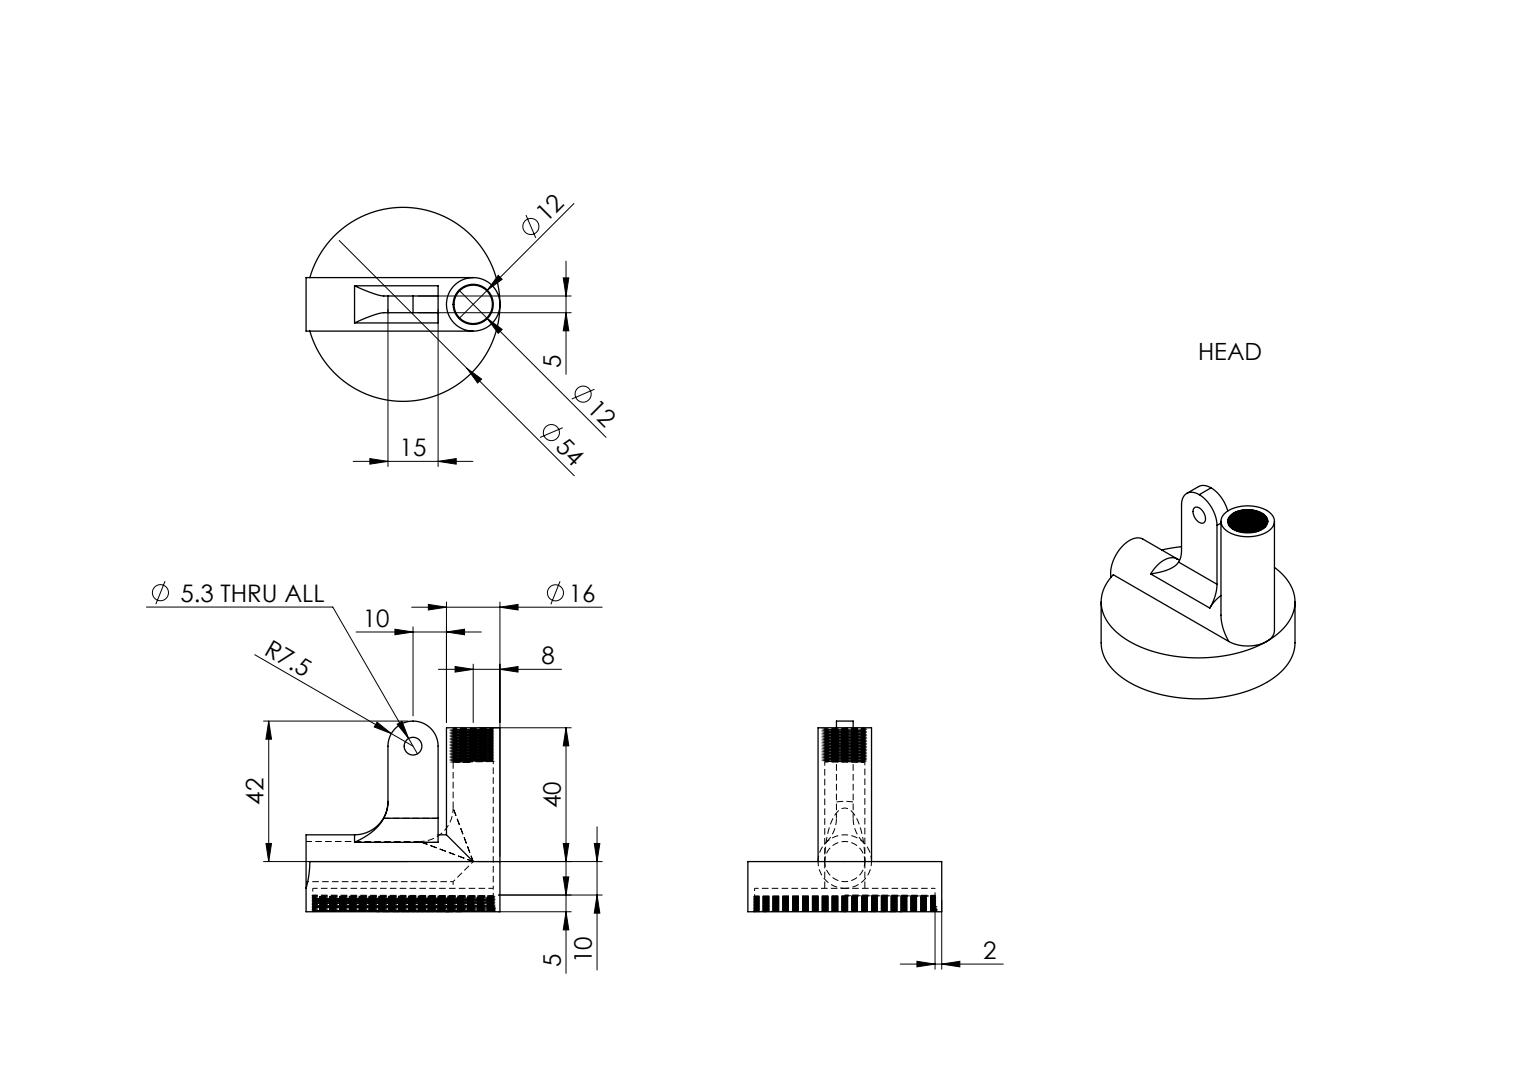
ISO-10303-21;
HEADER;
FILE_DESCRIPTION (('STEP AP214'),
    '1' );
FILE_NAME ('head.step',
    '2026-10-31T03:36:27',
    ( '' ),
    ( '' ),
    'SwSTEP 2.0',
    'SolidWorks 2026',
    '' );
FILE_SCHEMA (( 'AUTOMOTIVE_DESIGN' ));
ENDSEC;

DATA;
#9=CARTESIAN_POINT ( 'NONE',  ( -13.62178482187498396, 196.7843750006145456, 23.59362340125808188 ) ) ;
#16=CARTESIAN_POINT ( 'NONE',  ( 18.00000000000000000, 239.6312500012290343, -5.196152422706630247 ) ) ;
#27=CARTESIAN_POINT ( 'NONE',  ( 26.75643035624999655, 248.1718750006145342, -7.049594010296217766E-16 ) ) ;
#29=CARTESIAN_POINT ( 'NONE',  ( -17.60279642935561029, 194.9999999999999716, 20.73731651351060989 ) ) ;
#47=CARTESIAN_POINT ( 'NONE',  ( 22.60769515458672529, 246.3236538117967029, -6.000000000000004441 ) ) ;
#48=CARTESIAN_POINT ( 'NONE',  ( 26.75643035624999655, 244.7218750006145456, -3.323476615752271712 ) ) ;
#50=LINE ( 'NONE', #15224, #14231 ) ;
#52=ORIENTED_EDGE ( 'NONE', *, *, #4531, .T. ) ;
#54=CARTESIAN_POINT ( 'NONE',  ( 23.99999999999999645, 245.8562500012290570, -5.196152422706631135 ) ) ;
#63=ORIENTED_EDGE ( 'NONE', *, *, #14775, .T. ) ;
#69=CARTESIAN_POINT ( 'NONE',  ( 23.87821517812499650, 246.8968750006145285, -4.985214923628404904 ) ) ;
#73=CARTESIAN_POINT ( 'NONE',  ( 19.06670604969950489, 215.1554505341192964, -5.693556627486040966 ) ) ;
#95=DIRECTION ( 'NONE',  ( 0.000000000000000000, 0.000000000000000000, 1.000000000000000000 ) ) ;
#99=CARTESIAN_POINT ( 'NONE',  ( 5.727106289114498080E-15, 196.0625000000000000, 31.17691453623979214 ) ) ;
#102=CARTESIAN_POINT ( 'NONE',  ( 26.75643035624999655, 247.8718750006145228, -3.323476615752271268 ) ) ;
#110=CARTESIAN_POINT ( 'NONE',  ( 26.99999999999999645, 240.2874999999999659, 3.464101615137751278 ) ) ;
#116=VECTOR ( 'NONE', #35899, 1000.000000000000000 ) ;
#117=CARTESIAN_POINT ( 'NONE',  ( 26.99999999999999645, 194.9750000012290343, -15.58845726811990495 ) ) ;
#120=ADVANCED_FACE ( 'NONE', ( #26675 ), #705, .F. ) ;
#132=CARTESIAN_POINT ( 'NONE',  ( -1.926257025242585782E-15, 195.6968750006145683, -31.45816453501075927 ) ) ;
#144=CYLINDRICAL_SURFACE ( 'NONE', #32201, 27.00000000000000000 ) ;
#145=CARTESIAN_POINT ( 'NONE',  ( 22.60769515458672885, 244.9174038105676630, -5.999999999999998224 ) ) ;
#146=ADVANCED_FACE ( 'NONE', ( #11518 ), #17218, .F. ) ;
#148=CARTESIAN_POINT ( 'NONE',  ( -13.50000000000000533, 195.0875000012290457, -23.38268590217984411 ) ) ;
#149=VERTEX_POINT ( 'NONE', #2983 ) ;
#152=LINE ( 'NONE', #25749, #18668 ) ;
#156=CARTESIAN_POINT ( 'NONE',  ( 18.00000000000000355, 248.7249999999999943, 5.196152422706632912 ) ) ;
#157=CARTESIAN_POINT ( 'NONE',  ( 27.24356964374999279, 197.8156250006145171, -15.72908226750539207 ) ) ;
#163=CARTESIAN_POINT ( 'NONE',  ( -13.62178482187498396, 198.5281250006145228, 23.59362340125808188 ) ) ;
#164=CARTESIAN_POINT ( 'NONE',  ( 23.87821517812500005, 243.1468750006145285, 4.985214923628404016 ) ) ;
#169=CARTESIAN_POINT ( 'NONE',  ( 23.87821517812499650, 246.5593750006145228, -4.985214923628404904 ) ) ;
#173=CARTESIAN_POINT ( 'NONE',  ( 26.75643035624999655, 241.9093750006145171, -3.323476615752271268 ) ) ;
#175=EDGE_CURVE ( 'NONE', #2711, #16688, #11211, .T. ) ;
#176=CARTESIAN_POINT ( 'NONE',  ( 26.99999999999999645, 246.6812500012290457, -7.347880794884117764E-16 ) ) ;
#177=AXIS2_PLACEMENT_3D ( 'NONE', #6579, #20812, #23648 ) ;
#189=CARTESIAN_POINT ( 'NONE',  ( 21.00000000000000000, 241.9843750006145058, -6.646953231504538984 ) ) ;
#190=VERTEX_POINT ( 'NONE', #2796 ) ;
#196=DIRECTION ( 'NONE',  ( -0.000000000000000000, -0.000000000000000000, 1.000000000000000000 ) ) ;
#197=CARTESIAN_POINT ( 'NONE',  ( 5.778771075727756162E-15, 195.0218750006145569, 31.45816453501075927 ) ) ;
#198=EDGE_CURVE ( 'NONE', #717, #36155, #34079, .T. ) ;
#200=CARTESIAN_POINT ( 'NONE',  ( -7.234628195640263826, 196.8700961906613713, -27.00000000000003553 ) ) ;
#206=CARTESIAN_POINT ( 'NONE',  ( 26.75643035624999655, 249.4843750006145058, 3.323476615752267715 ) ) ;
#211=EDGE_CURVE ( 'NONE', #2909, #23659, #28387, .T. ) ;
#217=CARTESIAN_POINT ( 'NONE',  ( 15.24356964375000167, 248.4343750006145513, 3.323476615752272600 ) ) ;
#219=CARTESIAN_POINT ( 'NONE',  ( -17.17757150371551944, 194.9999999999999716, 21.09399746705422984 ) ) ;
#223=CARTESIAN_POINT ( 'NONE',  ( -28.99999999999999645, 201.9999999999999716, -1.007612034238798379E-23 ) ) ;
#224=CARTESIAN_POINT ( 'NONE',  ( 20.99999999999997868, 210.0000000000000000, -5.999999999999999112 ) ) ;
#234=CARTESIAN_POINT ( 'NONE',  ( 21.00000000000000000, 242.4625000000000057, 5.999999999999998224 ) ) ;
#237=CARTESIAN_POINT ( 'NONE',  ( 26.99999999999999645, 196.3250000012290570, -15.58845726811990495 ) ) ;
#239=CARTESIAN_POINT ( 'NONE',  ( 22.60769515458672885, 246.1388461906613827, 5.999999999999997335 ) ) ;
#240=CARTESIAN_POINT ( 'NONE',  ( 21.00000000000000000, 244.5718750006145115, 6.646953231504538984 ) ) ;
#245=CARTESIAN_POINT ( 'NONE',  ( 15.00000000000000000, 246.4562500012290513, 0.000000000000000000 ) ) ;
#248=CARTESIAN_POINT ( 'NONE',  ( 20.99999999999997868, 246.9625000000000057, 5.999999999999999112 ) ) ;
#253=VERTEX_POINT ( 'NONE', #25549 ) ;
#257=CARTESIAN_POINT ( 'NONE',  ( 15.24356964374999990, 246.1468750006145285, 0.000000000000000000 ) ) ;
#261=CARTESIAN_POINT ( 'NONE',  ( 17.34006124879648425, 219.7598366698888981, -4.770645753573318437 ) ) ;
#272=ORIENTED_EDGE ( 'NONE', *, *, #322, .F. ) ;
#282=LINE ( 'NONE', #23417, #32949 ) ;
#284=CARTESIAN_POINT ( 'NONE',  ( -26.99999999999998934, 195.9875000000000114, 15.58845726811991561 ) ) ;
#287=CARTESIAN_POINT ( 'NONE',  ( 20.99999999999999645, 245.9218750006145626, 6.646953231504538984 ) ) ;
#291=CARTESIAN_POINT ( 'NONE',  ( 20.99999999999999645, 185.0294372515228645, -5.999999999999999112 ) ) ;
#295=CARTESIAN_POINT ( 'NONE',  ( 26.99999999999999645, 241.6374999999999886, 3.464101615137751278 ) ) ;
#299=EDGE_LOOP ( 'NONE', ( #11498, #11713, #35971, #5755 ) ) ;
#306=CARTESIAN_POINT ( 'NONE',  ( 15.24356964374999990, 239.9593750006145285, 0.000000000000000000 ) ) ;
#316=CARTESIAN_POINT ( 'NONE',  ( 25.00272249592519103, 194.9999999999998863, 10.65893590749716324 ) ) ;
#317=CARTESIAN_POINT ( 'NONE',  ( -27.24356964375000345, 195.8093750006145513, 0.000000000000000000 ) ) ;
#321=CARTESIAN_POINT ( 'NONE',  ( 15.00000000000000000, 244.6187500012290741, -3.464101615137752610 ) ) ;
#322=EDGE_CURVE ( 'NONE', #20414, #21332, #8073, .T. ) ;
#334=CARTESIAN_POINT ( 'NONE',  ( -20.80563922340697403, 195.0000000000000284, -17.20829382900668136 ) ) ;
#339=CARTESIAN_POINT ( 'NONE',  ( -1.926257025242585782E-15, 196.5968750006145456, -31.45816453501076637 ) ) ;
#343=CARTESIAN_POINT ( 'NONE',  ( 26.99999999999999645, 249.3249999999999886, -7.347880794884117764E-16 ) ) ;
#344=CARTESIAN_POINT ( 'NONE',  ( 13.62178482187499640, 197.4031250006145228, -23.59362340125807123 ) ) ;
#346=APPLICATION_CONTEXT ( 'automotive_design' ) ;
#350=CARTESIAN_POINT ( 'NONE',  ( 27.24356964375000700, 195.0406250006145399, 15.72908226750537075 ) ) ;
#351=CARTESIAN_POINT ( 'NONE',  ( 21.00000000000000000, 241.5343750006145171, -6.646953231504538984 ) ) ;
#355=CARTESIAN_POINT ( 'NONE',  ( 15.24356964375000167, 248.0968750006145456, 3.323476615752272600 ) ) ;
#356=( BOUNDED_CURVE ( )  B_SPLINE_CURVE ( 2, ( #17925, #26623, #26814, #31940, #5972, #15073, #12223, #29469, #653 ),
 .UNSPECIFIED., .F., .F. ) 
 B_SPLINE_CURVE_WITH_KNOTS ( ( 3, 2, 2, 2, 3 ),
 ( 0.7934782608695651884, 0.7971014492753623060, 0.8043478260869565410, 0.8115942028985507761, 0.8152173913043478937 ),
 .UNSPECIFIED. ) 
 CURVE ( )  GEOMETRIC_REPRESENTATION_ITEM ( )  RATIONAL_B_SPLINE_CURVE ( ( 0.9330127018922194093, 0.9330127018922194093, 1.000000000000000000, 0.8660254037844387076, 1.000000000000000000, 0.8660254037844387076, 1.000000000000000000, 0.9330127018922182991, 0.9330127018922192983 ) ) 
 REPRESENTATION_ITEM ( '' )  );
#360=CARTESIAN_POINT ( 'NONE',  ( 23.87821517812499650, 241.9468750006145115, -4.985214923628404904 ) ) ;
#367=CARTESIAN_POINT ( 'NONE',  ( 0.000000000000000000, 210.0000000000000284, 0.000000000000000000 ) ) ;
#369=CARTESIAN_POINT ( 'NONE',  ( 12.48663586349064403, 194.9999999999999716, 24.21355016816918493 ) ) ;
#376=CARTESIAN_POINT ( 'NONE',  ( 23.87821517812499650, 241.4968750006144944, -4.985214923628404904 ) ) ;
#382=CARTESIAN_POINT ( 'NONE',  ( 26.99999999999999645, 241.6375000000000171, 3.464101615137751278 ) ) ;
#390=CARTESIAN_POINT ( 'NONE',  ( 26.75643035624999655, 248.6593750006145171, -3.323476615752271712 ) ) ;
#394=CARTESIAN_POINT ( 'NONE',  ( 2.999999999999997335, 244.5000000000000000, 2.500000000000000000 ) ) ;
#401=CARTESIAN_POINT ( 'NONE',  ( 20.99999999999999289, 245.4437500012290343, -5.999999999999997335 ) ) ;
#406=AXIS2_PLACEMENT_3D ( 'NONE', #8514, #8149, #2814 ) ;
#408=CARTESIAN_POINT ( 'NONE',  ( 15.00000000000000000, 248.6500000000000057, 0.000000000000000000 ) ) ;
#414=EDGE_CURVE ( 'NONE', #36155, #4778, #26130, .T. ) ;
#421=CARTESIAN_POINT ( 'NONE',  ( 13.50000000000001421, 195.7625000012290570, 23.38268590217984055 ) ) ;
#422=CARTESIAN_POINT ( 'NONE',  ( -1.045839947578415010E-13, 196.1750000012290229, 27.00000000000000355 ) ) ;
#425=EDGE_CURVE ( 'NONE', #21070, #14808, #25046, .T. ) ;
#426=CARTESIAN_POINT ( 'NONE',  ( 21.00000000000000000, 245.2468750006145228, -6.646953231504538984 ) ) ;
#428=CARTESIAN_POINT ( 'NONE',  ( 18.12178482187500350, 240.0343750006145171, 4.985214923628407568 ) ) ;
#431=VECTOR ( 'NONE', #33908, 1000.000000000000000 ) ;
#432=CARTESIAN_POINT ( 'NONE',  ( 21.00000000000000000, 247.2437500012290457, -6.928203230275506996 ) ) ;
#439=ORIENTED_EDGE ( 'NONE', *, *, #30910, .T. ) ;
#443=CARTESIAN_POINT ( 'NONE',  ( 26.75643035624999655, 247.6843750006145513, 3.323476615752267715 ) ) ;
#446=CARTESIAN_POINT ( 'NONE',  ( 20.28004929559795499, 210.7199507044251732, -5.999999999998712141 ) ) ;
#472=CARTESIAN_POINT ( 'NONE',  ( 26.75643035624999655, 245.6218750006145513, -3.323476615752271268 ) ) ;
#473=ORIENTED_EDGE ( 'NONE', *, *, #4147, .F. ) ;
#480=CARTESIAN_POINT ( 'NONE',  ( 15.00000000000000000, 241.4124999999999943, -3.464101615137752166 ) ) ;
#483=VERTEX_POINT ( 'NONE', #17594 ) ;
#485=ORIENTED_EDGE ( 'NONE', *, *, #35805, .T. ) ;
#488=CARTESIAN_POINT ( 'NONE',  ( 23.99999999999999645, 243.1000000000000227, -5.196152422706631135 ) ) ;
#493=CARTESIAN_POINT ( 'NONE',  ( 26.75643035624999655, 241.4968750006145228, 3.323476615752267715 ) ) ;
#502=CARTESIAN_POINT ( 'NONE',  ( 27.24356964374999635, 196.0718750006145683, -15.72908226750539029 ) ) ;
#511=( BOUNDED_CURVE ( )  B_SPLINE_CURVE ( 2, ( #32601, #35627, #6825, #12519, #18216, #9301, #29756, #1322, #32976, #12324, #3608, #27109, #24272, #35815, #30140, #26534, #15740, #564, #35248, #20873, #32412, #6454, #18026, #30707, #4726, #36373, #1507, #16302, #27480, #16490, #19157, #25003, #21994, #1694, #2070, #4909, #7769, #10976, #19347, #30522, #36559, #10419, #13082, #13268, #27849, #10231, #24636, #28038, #30328, #8146, #13644, #36187, #22180, #31076, #30886, #25197, #2254, #36750, #10790, #33727, #33359, #4541, #7394, #10600, #21806, #22364, #1882, #33912, #33541, #4352, #22547, #18967, #7954, #19529, #5099, #16678, #34096, #28225, #7581, #15932, #13453, #25379, #13833, #16118, #27669, #36929, #24820, #339, #20454, #34647, #20266, #34468, #5842, #5284, #28584, #37482, #8511, #14381, #6025, #22737, #2998, #20077, #34286, #23291, #19718, #14568, #31805, #8330, #16864, #8692, #37302, #19900, #17420, #11904, #23104, #5463, #28960, #35024, #11533, #34836, #31258, #2811, #31441, #17611, #28401, #17046, #14198, #26120, #25939, #31622, #2622 ),
 .UNSPECIFIED., .F., .F. ) 
 B_SPLINE_CURVE_WITH_KNOTS ( ( 3, 2, 2, 2, 2, 2, 2, 2, 2, 2, 2, 2, 2, 2, 2, 2, 2, 2, 2, 2, 2, 2, 2, 2, 2, 2, 2, 2, 2, 2, 2, 2, 2, 2, 2, 2, 2, 2, 2, 2, 2, 2, 2, 2, 2, 2, 2, 2, 2, 2, 2, 2, 2, 2, 2, 2, 2, 2, 2, 2, 2, 2, 2, 2, 2, 3 ),
 ( 0.000000000000000000, 0.01388888888888888812, 0.02777777777777777624, 0.04166666666666666435, 0.05555555555555555247, 0.06944444444444444753, 0.08333333333333332871, 0.09722222222222222376, 0.1111111111111111049, 0.1250000000000000000, 0.1388888888888888951, 0.1527777777777777901, 0.1666666666666666574, 0.1805555555555555525, 0.1944444444444444475, 0.2083333333333333426, 0.2222222222222222099, 0.2361111111111111049, 0.2500000000000000000, 0.2638888888888888951, 0.2777777777777777901, 0.2916666666666666852, 0.3055555555555555802, 0.3194444444444444198, 0.3333333333333333148, 0.3472222222222222099, 0.3611111111111111049, 0.3750000000000000000, 0.3888888888888888951, 0.4027777777777777901, 0.4166666666666666852, 0.4305555555555555802, 0.4444444444444444198, 0.4583333333333333148, 0.4722222222222222099, 0.4861111111111111049, 0.5000000000000000000, 0.5138888888888888395, 0.5277777777777777901, 0.5416666666666666297, 0.5555555555555555802, 0.5694444444444444198, 0.5833333333333333703, 0.5972222222222222099, 0.6111111111111111605, 0.6250000000000000000, 0.6388888888888888395, 0.6527777777777777901, 0.6666666666666666297, 0.6805555555555555802, 0.6944444444444444198, 0.7083333333333333703, 0.7222222222222222099, 0.7361111111111111605, 0.7500000000000000000, 0.7638888888888888395, 0.7777777777777777901, 0.7916666666666666297, 0.8055555555555555802, 0.8194444444444444198, 0.8333333333333333703, 0.8472222222222222099, 0.8611111111111111605, 0.8750000000000000000, 0.8888888888888888395, 0.8996968925187518451 ),
 .UNSPECIFIED. ) 
 CURVE ( )  GEOMETRIC_REPRESENTATION_ITEM ( )  RATIONAL_B_SPLINE_CURVE ( ( 1.000000000000000000, 0.8660254037844387076, 1.000000000000000000, 0.8660254037844387076, 1.000000000000000000, 0.8660254037844387076, 1.000000000000000000, 0.8660254037844387076, 1.000000000000000000, 0.8660254037844387076, 1.000000000000000000, 0.8660254037844387076, 1.000000000000000000, 0.8660254037844387076, 1.000000000000000000, 0.8660254037844387076, 1.000000000000000000, 0.8660254037844387076, 1.000000000000000000, 0.8660254037844387076, 1.000000000000000000, 0.8660254037844387076, 1.000000000000000000, 0.8660254037844387076, 1.000000000000000000, 0.8660254037844387076, 1.000000000000000000, 0.8660254037844387076, 1.000000000000000000, 0.8660254037844387076, 1.000000000000000000, 0.8660254037844387076, 1.000000000000000000, 0.8660254037844387076, 1.000000000000000000, 0.8660254037844387076, 1.000000000000000000, 0.8660254037844387076, 1.000000000000000000, 0.8660254037844387076, 1.000000000000000000, 0.8660254037844387076, 1.000000000000000000, 0.8660254037844387076, 1.000000000000000000, 0.8660254037844387076, 1.000000000000000000, 0.8660254037844387076, 1.000000000000000000, 0.8660254037844387076, 1.000000000000000000, 0.8660254037844387076, 1.000000000000000000, 0.8660254037844387076, 1.000000000000000000, 0.8660254037844387076, 1.000000000000000000, 0.8660254037844387076, 1.000000000000000000, 0.8660254037844387076, 1.000000000000000000, 0.8660254037844387076, 1.000000000000000000, 0.8660254037844387076, 1.000000000000000000, 0.8660254037844387076, 1.000000000000000000, 0.8660254037844387076, 1.000000000000000000, 0.8660254037844387076, 1.000000000000000000, 0.8660254037844387076, 1.000000000000000000, 0.8660254037844387076, 1.000000000000000000, 0.8660254037844387076, 1.000000000000000000, 0.8660254037844387076, 1.000000000000000000, 0.8660254037844387076, 1.000000000000000000, 0.8660254037844387076, 1.000000000000000000, 0.8660254037844387076, 1.000000000000000000, 0.8660254037844387076, 1.000000000000000000, 0.8660254037844387076, 1.000000000000000000, 0.8660254037844387076, 1.000000000000000000, 0.8660254037844387076, 1.000000000000000000, 0.8660254037844387076, 1.000000000000000000, 0.8660254037844387076, 1.000000000000000000, 0.8660254037844387076, 1.000000000000000000, 0.8660254037844387076, 1.000000000000000000, 0.8660254037844387076, 1.000000000000000000, 0.8660254037844387076, 1.000000000000000000, 0.8660254037844387076, 1.000000000000000000, 0.8660254037844387076, 1.000000000000000000, 0.8660254037844387076, 1.000000000000000000, 0.8660254037844387076, 1.000000000000000000, 0.8660254037844387076, 1.000000000000000000, 0.8660254037844387076, 1.000000000000000000, 0.8660254037844387076, 1.000000000000000000, 0.8660254037844387076, 1.000000000000000000, 0.8660254037844387076, 1.000000000000000000, 0.8660254037844387076, 1.000000000000000000, 0.8660254037844387076, 1.000000000000000000, 0.8660254037844387076, 1.000000000000000000, 0.8957441496010808413, 0.9537471549767810863 ) ) 
 REPRESENTATION_ITEM ( '' )  );
#516=CARTESIAN_POINT ( 'NONE',  ( 7.234628195640312676, 199.5299038117966859, -27.00000000000000711 ) ) ;
#521=CARTESIAN_POINT ( 'NONE',  ( 1.120210788295102201E-13, 195.5000000012290400, -27.00000000000000711 ) ) ;
#525=CARTESIAN_POINT ( 'NONE',  ( 23.99999999999999645, 248.0499999999999829, -5.196152422706631135 ) ) ;
#526=CARTESIAN_POINT ( 'NONE',  ( 27.24356964374999279, 197.3656250006145285, -15.72908226750539207 ) ) ;
#529=VERTEX_POINT ( 'NONE', #35570 ) ;
#530=ORIENTED_EDGE ( 'NONE', *, *, #7271, .T. ) ;
#531=CARTESIAN_POINT ( 'NONE',  ( 13.62178482187501416, 195.0031250006145456, 23.59362340125806767 ) ) ;
#532=CARTESIAN_POINT ( 'NONE',  ( 26.75643035624999655, 240.1093750006145342, -3.323476615752271712 ) ) ;
#536=CARTESIAN_POINT ( 'NONE',  ( 15.24356964374999990, 247.1218750006145228, -3.323476615752268604 ) ) ;
#542=CARTESIAN_POINT ( 'NONE',  ( 26.75643035624999655, 241.0093750006145115, -3.323476615752271268 ) ) ;
#549=CYLINDRICAL_SURFACE ( 'NONE', #10694, 27.00000000000000000 ) ;
#552=CARTESIAN_POINT ( 'NONE',  ( 26.99999999999999645, 248.4250000000000114, -7.347880794884117764E-16 ) ) ;
#556=CARTESIAN_POINT ( 'NONE',  ( 19.39230484541326049, 247.7138461906614282, -5.999999999999994671 ) ) ;
#557=ADVANCED_FACE ( 'NONE', ( #3167 ), #20623, .F. ) ;
#560=CARTESIAN_POINT ( 'NONE',  ( 21.00000000000000000, 242.8843750006145399, -6.646953231504538984 ) ) ;
#563=CARTESIAN_POINT ( 'NONE',  ( 21.00000000000000000, 243.8687500012290172, 5.999999999999998224 ) ) ;
#564=CARTESIAN_POINT ( 'NONE',  ( 27.24356964374999279, 199.2218750006145171, -15.72908226750539207 ) ) ;
#567=DIRECTION ( 'NONE',  ( -0.000000000000000000, 1.000000000000000000, -0.000000000000000000 ) ) ;
#572=CARTESIAN_POINT ( 'NONE',  ( 21.00000000000000000, 249.6343750006145399, -6.646953231504538984 ) ) ;
#576=CARTESIAN_POINT ( 'NONE',  ( 26.99999999999999645, 248.0124999999999602, -3.464101615137755275 ) ) ;
#577=EDGE_LOOP ( 'NONE', ( #17705, #26737, #27106, #20978 ) ) ;
#581=EDGE_CURVE ( 'NONE', #7872, #24534, #12201, .T. ) ;
#584=CARTESIAN_POINT ( 'NONE',  ( 20.99999999999999645, 248.5093750006144830, 6.646953231504538984 ) ) ;
#586=EDGE_CURVE ( 'NONE', #12855, #5744, #3208, .T. ) ;
#591=CARTESIAN_POINT ( 'NONE',  ( 18.00000000000000355, 248.7249999999999943, 5.196152422706632912 ) ) ;
#605=CARTESIAN_POINT ( 'NONE',  ( 20.99999999999999645, 185.0294372515228645, 5.999999999999999112 ) ) ;
#609=CARTESIAN_POINT ( 'NONE',  ( 15.24356964374999990, 243.1093750006145342, 0.000000000000000000 ) ) ;
#614=CARTESIAN_POINT ( 'NONE',  ( 15.00000000000000000, 245.5562500012290457, 0.000000000000000000 ) ) ;
#618=( BOUNDED_CURVE ( )  B_SPLINE_CURVE ( 2, ( #14056, #30566, #4584, #23146, #34688, #17273, #8919, #2664, #563 ),
 .UNSPECIFIED., .F., .F. ) 
 B_SPLINE_CURVE_WITH_KNOTS ( ( 3, 2, 2, 2, 3 ),
 ( 0.5326086956521739468, 0.5362318840579710644, 0.5434782608695651884, 0.5507246376811594235, 0.5543478260869565410 ),
 .UNSPECIFIED. ) 
 CURVE ( )  GEOMETRIC_REPRESENTATION_ITEM ( )  RATIONAL_B_SPLINE_CURVE ( ( 0.9330127018922194093, 0.9330127018922194093, 1.000000000000000000, 0.8660254037844387076, 1.000000000000000000, 0.8660254037844387076, 1.000000000000000000, 0.9330127018922194093, 0.9330127018922194093 ) ) 
 REPRESENTATION_ITEM ( '' )  );
#627=CARTESIAN_POINT ( 'NONE',  ( 18.12178482187499640, 246.0718750006145115, -4.985214923628404904 ) ) ;
#637=( BOUNDED_CURVE ( )  B_SPLINE_CURVE ( 2, ( #9247, #31797, #17784, #9061, #32362, #11896, #20632, #20820, #23284 ),
 .UNSPECIFIED., .F., .F. ) 
 B_SPLINE_CURVE_WITH_KNOTS ( ( 3, 2, 2, 2, 3 ),
 ( 0.4021739130434782705, 0.4057971014492753881, 0.4130434782608695676, 0.4202898550724637472, 0.4239130434782608647 ),
 .UNSPECIFIED. ) 
 CURVE ( )  GEOMETRIC_REPRESENTATION_ITEM ( )  RATIONAL_B_SPLINE_CURVE ( ( 0.9330127018922194093, 0.9330127018922194093, 1.000000000000000000, 0.8660254037844387076, 1.000000000000000000, 0.8660254037844387076, 1.000000000000000000, 0.9330127018922194093, 0.9330127018922194093 ) ) 
 REPRESENTATION_ITEM ( '' )  );
#645=CARTESIAN_POINT ( 'NONE',  ( 19.95811093400027403, 239.6067736145540152, -5.908846518073574750 ) ) ;
#647=AXIS2_PLACEMENT_3D ( 'NONE', #18195, #29735, #18006 ) ;
#649=CARTESIAN_POINT ( 'NONE',  ( 21.00000000000001066, 247.0187500012290513, 5.999999999999998224 ) ) ;
#653=CARTESIAN_POINT ( 'NONE',  ( 20.99999999999995381, 241.1687500012290570, 5.999999999999998224 ) ) ;
#656=CARTESIAN_POINT ( 'NONE',  ( 20.99999999999999645, 245.6968750006145399, -6.646953231504538984 ) ) ;
#659=DIRECTION ( 'NONE',  ( 0.000000000000000000, 0.000000000000000000, -1.000000000000000000 ) ) ;
#660=DIRECTION ( 'NONE',  ( 0.000000000000000000, 1.000000000000000000, 0.000000000000000000 ) ) ;
#663=CARTESIAN_POINT ( 'NONE',  ( 21.00000000000000000, 241.1125000000000114, 6.928203230275506996 ) ) ;
#670=EDGE_CURVE ( 'NONE', #32512, #7058, #35888, .T. ) ;
#677=CARTESIAN_POINT ( 'NONE',  ( 20.99999999999999289, 249.2125000000000057, 5.999999999999999112 ) ) ;
#679=VECTOR ( 'NONE', #1496, 1000.000000000000000 ) ;
#688=CARTESIAN_POINT ( 'NONE',  ( -1.926257025242585782E-15, 198.3406250006145228, -31.45816453501075927 ) ) ;
#691=ORIENTED_EDGE ( 'NONE', *, *, #2981, .T. ) ;
#693=CARTESIAN_POINT ( 'NONE',  ( 18.00000000000000000, 244.5812500012290513, -5.196152422706630247 ) ) ;
#700=CARTESIAN_POINT ( 'NONE',  ( 20.99999999999999645, 250.0000000000000000, -5.999999999999999112 ) ) ;
#704=CARTESIAN_POINT ( 'NONE',  ( -29.00000000000002487, 210.0000000000000000, 0.000000000000000000 ) ) ;
#705=CYLINDRICAL_SURFACE ( 'NONE', #13506, 5.999999999999999112 ) ;
#713=CARTESIAN_POINT ( 'NONE',  ( 26.99999999999999645, 247.9375000000000000, 3.464101615137751278 ) ) ;
#714=CARTESIAN_POINT ( 'NONE',  ( 13.62178482187499640, 195.6031250006145115, -23.59362340125807123 ) ) ;
#717=VERTEX_POINT ( 'NONE', #4111 ) ;
#718=CARTESIAN_POINT ( 'NONE',  ( -27.24356964374999635, 196.6906250006145456, 15.72908226750539384 ) ) ;
#719=CARTESIAN_POINT ( 'NONE',  ( 19.00081547855239350, 239.7604221912915818, -5.492723509887031952 ) ) ;
#722=CARTESIAN_POINT ( 'NONE',  ( 23.87821517812499650, 248.8093750006145228, -4.985214923628404904 ) ) ;
#730=CARTESIAN_POINT ( 'NONE',  ( 20.99999999999999645, 241.5343750006145171, -6.646953231504538984 ) ) ;
#741=CARTESIAN_POINT ( 'NONE',  ( 26.99999999999999645, 248.4625000000000057, -3.464101615137755275 ) ) ;
#749=CARTESIAN_POINT ( 'NONE',  ( 21.00000000000000000, 243.3343750006145285, -6.646953231504538984 ) ) ;
#764=CARTESIAN_POINT ( 'NONE',  ( 21.00000000000000000, 246.4843750006145058, -6.646953231504538984 ) ) ;
#770=EDGE_LOOP ( 'NONE', ( #13450, #36497, #28822 ) ) ;
#776=EDGE_CURVE ( 'NONE', #35917, #28635, #13022, .T. ) ;
#778=CARTESIAN_POINT ( 'NONE',  ( 18.00000000000000355, 245.6312500012290343, 5.196152422706632912 ) ) ;
#779=CARTESIAN_POINT ( 'NONE',  ( 13.50000000000001421, 196.5500000000000114, 23.38268590217984055 ) ) ;
#784=CARTESIAN_POINT ( 'NONE',  ( 2.999999999999997335, 252.0000000000000000, -2.500000000000000000 ) ) ;
#799=CARTESIAN_POINT ( 'NONE',  ( 1.255007937094097924E-14, 199.4375000000000284, -27.00000000000000355 ) ) ;
#806=CARTESIAN_POINT ( 'NONE',  ( 26.99999999999999645, 244.3937500012290513, 3.464101615137751278 ) ) ;
#809=FACE_BOUND ( 'NONE', #24901, .T. ) ;
#818=CARTESIAN_POINT ( 'NONE',  ( 26.75643035624999655, 244.1593750006145171, -3.323476615752271712 ) ) ;
#819=ADVANCED_FACE ( 'NONE', ( #19094 ), #30646, .F. ) ;
#824=FILL_AREA_STYLE_COLOUR ( '', #4427 ) ;
#843=CARTESIAN_POINT ( 'NONE',  ( -27.00000000000000355, 195.4625000000000057, -15.58845726811989429 ) ) ;
#847=CARTESIAN_POINT ( 'NONE',  ( 26.75643035624999655, 246.0718750006145399, -3.323476615752271268 ) ) ;
#848=CIRCLE ( 'NONE', #26888, 5.999999999999999112 ) ;
#862=CARTESIAN_POINT ( 'NONE',  ( 27.00000000000000355, 196.7375000012290229, -3.306546357697854128E-15 ) ) ;
#864=CARTESIAN_POINT ( 'NONE',  ( 27.00000000000001421, 195.2375000000000114, 15.58845726811988897 ) ) ;
#869=CARTESIAN_POINT ( 'NONE',  ( 11.24016333012528257, 213.6599387512013095, 4.770645753574775050 ) ) ;
#878=CARTESIAN_POINT ( 'NONE',  ( 15.00000000000000000, 241.0000000000000000, 0.000000000000000000 ) ) ;
#879=CARTESIAN_POINT ( 'NONE',  ( -13.62178482187498396, 199.4281250006145569, 23.59362340125808188 ) ) ;
#884=CARTESIAN_POINT ( 'NONE',  ( -5.023457906468643763, 224.4868866335225448, -2.499999999999999556 ) ) ;
#885=CARTESIAN_POINT ( 'NONE',  ( 20.00041244883536606, 239.7473985345926053, -5.668978318349186196 ) ) ;
#889=EDGE_CURVE ( 'NONE', #36288, #26422, #2026, .T. ) ;
#897=CARTESIAN_POINT ( 'NONE',  ( 21.00000000000000000, 247.4687500012290400, 5.999999999999998224 ) ) ;
#898=ORIENTED_EDGE ( 'NONE', *, *, #5997, .F. ) ;
#906=CARTESIAN_POINT ( 'NONE',  ( 24.00000000000000000, 247.4500000000000171, 5.196152422706629359 ) ) ;
#907=CARTESIAN_POINT ( 'NONE',  ( -13.62178482187498396, 196.7281250006145399, 23.59362340125808188 ) ) ;
#913=CARTESIAN_POINT ( 'NONE',  ( -27.24356964374999990, 196.1656250006145399, -15.72908226750537786 ) ) ;
#918=TOROIDAL_SURFACE ( 'NONE', #30587, 18.00000000000000355, 10.00000000000000000 ) ;
#919=CARTESIAN_POINT ( 'NONE',  ( 21.00000000000000000, 248.1718750006145342, 6.646953231504538984 ) ) ;
#921=CARTESIAN_POINT ( 'NONE',  ( 1.069080835302379631E-14, 197.9750000012290343, 27.00000000000000000 ) ) ;
#925=CARTESIAN_POINT ( 'NONE',  ( 15.24356964374999990, 240.7093750006144717, -3.323476615752268604 ) ) ;
#935=CARTESIAN_POINT ( 'NONE',  ( 5.438367727407757144E-14, 198.5374999999999943, -27.00000000000000000 ) ) ;
#940=CARTESIAN_POINT ( 'NONE',  ( 26.75643035624999655, 240.4843750006145058, 3.323476615752267715 ) ) ;
#944=CARTESIAN_POINT ( 'NONE',  ( 22.60769515458672885, 242.4825961894323143, 5.999999999999997335 ) ) ;
#947=DIRECTION ( 'NONE',  ( -0.000000000000000000, 1.000000000000000000, -0.000000000000000000 ) ) ;
#953=CARTESIAN_POINT ( 'NONE',  ( 26.75643035624999655, 247.7218750006145171, -7.049594010296217766E-16 ) ) ;
#959=ORIENTED_EDGE ( 'NONE', *, *, #15902, .F. ) ;
#966=CARTESIAN_POINT ( 'NONE',  ( 20.99999999999999645, 245.5843750006145285, -6.646953231504538984 ) ) ;
#981=CARTESIAN_POINT ( 'NONE',  ( 3.253724281355069334E-15, 199.8875000000000455, -27.00000000000000355 ) ) ;
#987=CARTESIAN_POINT ( 'NONE',  ( 27.00000000000000355, 195.2750000000000057, -3.306546357697854128E-15 ) ) ;
#989=DIRECTION ( 'NONE',  ( 0.000000000000000000, 0.000000000000000000, -1.000000000000000000 ) ) ;
#994=CARTESIAN_POINT ( 'NONE',  ( 24.00000000000000000, 243.9062500012290400, 5.196152422706629359 ) ) ;
#997=CARTESIAN_POINT ( 'NONE',  ( 18.00000000000000355, 242.8750000000000000, 5.196152422706632912 ) ) ;
#1000=ORIENTED_EDGE ( 'NONE', *, *, #22405, .T. ) ;
#1001=ORIENTED_EDGE ( 'NONE', *, *, #29790, .F. ) ;
#1003=CARTESIAN_POINT ( 'NONE',  ( 15.24356964374999990, 244.3468750006145171, 0.000000000000000000 ) ) ;
#1018=VECTOR ( 'NONE', #12976, 1000.000000000000000 ) ;
#1028=EDGE_CURVE ( 'NONE', #1047, #2118, #24063, .T. ) ;
#1030=DIRECTION ( 'NONE',  ( -0.000000000000000000, 1.000000000000000000, -0.000000000000000000 ) ) ;
#1034=CARTESIAN_POINT ( 'NONE',  ( 20.99999999999999645, 240.7187500012290400, 5.999999999999998224 ) ) ;
#1036=CARTESIAN_POINT ( 'NONE',  ( 20.99999999999999645, 247.2718750006145001, 6.646953231504538984 ) ) ;
#1047=VERTEX_POINT ( 'NONE', #31380 ) ;
#1048=CARTESIAN_POINT ( 'NONE',  ( 1.120210788295102201E-13, 196.8500000012290343, -27.00000000000000711 ) ) ;
#1054=CARTESIAN_POINT ( 'NONE',  ( 22.60769515458672885, 243.4388461906613657, 5.999999999999997335 ) ) ;
#1066=CARTESIAN_POINT ( 'NONE',  ( 26.99999999999999645, 247.0374999999999943, 3.464101615137751278 ) ) ;
#1067=CARTESIAN_POINT ( 'NONE',  ( 13.62178482187499640, 197.8531250006145399, -23.59362340125807123 ) ) ;
#1074=CARTESIAN_POINT ( 'NONE',  ( 18.00000000000000355, 244.7312500012290570, 5.196152422706632912 ) ) ;
#1081=CARTESIAN_POINT ( 'NONE',  ( 15.00000000000000000, 240.6062500012290286, 0.000000000000000000 ) ) ;
#1083=DIRECTION ( 'NONE',  ( 0.000000000000000000, 0.000000000000000000, 1.000000000000000000 ) ) ;
#1086=CARTESIAN_POINT ( 'NONE',  ( 22.60769515458672885, 247.6736538117966973, -6.000000000000000000 ) ) ;
#1094=CARTESIAN_POINT ( 'NONE',  ( 15.00000000000000000, 246.8500000000000227, 0.000000000000000000 ) ) ;
#1095=CARTESIAN_POINT ( 'NONE',  ( -13.62178482187500528, 196.5781250006145342, -23.59362340125807123 ) ) ;
#1102=CARTESIAN_POINT ( 'NONE',  ( 5.778771075727756162E-15, 195.4156250006145399, 31.45816453501075927 ) ) ;
#1103=CARTESIAN_POINT ( 'NONE',  ( 18.12178482187499640, 239.7718750006145001, -4.985214923628404904 ) ) ;
#1106=CARTESIAN_POINT ( 'NONE',  ( 26.75643035624999655, 245.1718750006145058, -3.323476615752271712 ) ) ;
#1109=EDGE_CURVE ( 'NONE', #28768, #2711, #7134, .T. ) ;
#1112=VECTOR ( 'NONE', #33253, 1000.000000000000000 ) ;
#1114=CARTESIAN_POINT ( 'NONE',  ( 27.24356964374999635, 199.6718750006145058, -15.72908226750539029 ) ) ;
#1126=CARTESIAN_POINT ( 'NONE',  ( 15.00000000000000178, 248.2937500012290286, 3.464101615137757051 ) ) ;
#1129=CARTESIAN_POINT ( 'NONE',  ( 19.00081571707366379, 239.7604221881839521, -5.492723647597353320 ) ) ;
#1140=ORIENTED_EDGE ( 'NONE', *, *, #13192, .F. ) ;
#1141=CARTESIAN_POINT ( 'NONE',  ( 26.75643035624999655, 245.8843750006145399, 3.323476615752267715 ) ) ;
#1147=FACE_BOUND ( 'NONE', #16732, .T. ) ;
#1148=VERTEX_POINT ( 'NONE', #21138 ) ;
#1156=CARTESIAN_POINT ( 'NONE',  ( 20.99999999999999645, 245.8093750006144944, 6.646953231504538984 ) ) ;
#1176=CARTESIAN_POINT ( 'NONE',  ( -27.24356964375000345, 199.4093750006145456, 0.000000000000000000 ) ) ;
#1182=CARTESIAN_POINT ( 'NONE',  ( 23.99999999999999645, 244.0562500012290457, -5.196152422706631135 ) ) ;
#1185=CARTESIAN_POINT ( 'NONE',  ( 27.24356964375000700, 199.5406250006145683, 15.72908226750537075 ) ) ;
#1190=CARTESIAN_POINT ( 'NONE',  ( 26.75643035624999655, 244.1218750006145228, -7.049594010296217766E-16 ) ) ;
#1195=( LENGTH_UNIT ( ) NAMED_UNIT ( * ) SI_UNIT ( .MILLI., .METRE. ) );
#1205=DIRECTION ( 'NONE',  ( 1.000000000000000000, 0.000000000000000000, 0.000000000000000000 ) ) ;
#1208=LINE ( 'NONE', #15819, #2920 ) ;
#1218=CARTESIAN_POINT ( 'NONE',  ( 21.00000000000000000, 249.2968750006145342, -6.646953231504538984 ) ) ;
#1220=CARTESIAN_POINT ( 'NONE',  ( 23.87821517812499650, 244.3093750006145228, -4.985214923628404904 ) ) ;
#1227=CARTESIAN_POINT ( 'NONE',  ( 0.000000000000000000, 210.0000000000000284, 0.000000000000000000 ) ) ;
#1232=ORIENTED_EDGE ( 'NONE', *, *, #16331, .T. ) ;
#1233=CARTESIAN_POINT ( 'NONE',  ( -13.50000000000000533, 195.8750000000000284, -23.38268590217984411 ) ) ;
#1241=DIRECTION ( 'NONE',  ( 0.000000000000000000, 1.000000000000000000, 0.000000000000000000 ) ) ;
#1243=CARTESIAN_POINT ( 'NONE',  ( 15.00000000000000178, 243.7937500012290570, 3.464101615137757051 ) ) ;
#1251=AXIS2_PLACEMENT_3D ( 'NONE', #32704, #15845, #15660 ) ;
#1253=CARTESIAN_POINT ( 'NONE',  ( -27.24356964375000345, 197.5531250006145285, 0.000000000000000000 ) ) ;
#1256=ORIENTED_EDGE ( 'NONE', *, *, #6674, .F. ) ;
#1267=CARTESIAN_POINT ( 'NONE',  ( 20.99999999999995381, 242.9124999999999943, 5.999999999999998224 ) ) ;
#1270=CARTESIAN_POINT ( 'NONE',  ( 26.99999999999999645, 247.6187500012290741, -3.464101615137755275 ) ) ;
#1276=CARTESIAN_POINT ( 'NONE',  ( -13.49999999999998401, 195.6875000012290400, 23.38268590217985476 ) ) ;
#1279=CARTESIAN_POINT ( 'NONE',  ( 23.99999999999999645, 245.3500000000000227, -5.196152422706631135 ) ) ;
#1280=CARTESIAN_POINT ( 'NONE',  ( 13.62178482187499640, 195.1531250006145513, -23.59362340125807123 ) ) ;
#1284=AXIS2_PLACEMENT_3D ( 'NONE', #6745, #7064, #30364 ) ;
#1286=CARTESIAN_POINT ( 'NONE',  ( 27.00000000000000355, 198.0875000012290457, -3.306546357697854128E-15 ) ) ;
#1291=CARTESIAN_POINT ( 'NONE',  ( 23.87821517812500005, 244.1593750006145171, 4.985214923628404016 ) ) ;
#1294=FACE_OUTER_BOUND ( 'NONE', #9316, .T. ) ;
#1299=CARTESIAN_POINT ( 'NONE',  ( 26.75643035624999655, 240.0718750006145399, -7.049594010296217766E-16 ) ) ;
#1305=CYLINDRICAL_SURFACE ( 'NONE', #17735, 27.00000000000000000 ) ;
#1307=VECTOR ( 'NONE', #7532, 1000.000000000000000 ) ;
#1314=( BOUNDED_CURVE ( )  B_SPLINE_CURVE ( 3, ( #224, #25821, #19966, #5910 ),
 .UNSPECIFIED., .F., .F. ) 
 B_SPLINE_CURVE_WITH_KNOTS ( ( 4, 4 ),
 ( 4.712388980384690562, 6.283185307179586232 ),
 .UNSPECIFIED. ) 
 CURVE ( )  GEOMETRIC_REPRESENTATION_ITEM ( )  RATIONAL_B_SPLINE_CURVE ( ( 1.000000000000000000, 0.8047378541243652705, 0.8047378541243652705, 1.000000000000000000 ) ) 
 REPRESENTATION_ITEM ( '' )  );
#1317=CARTESIAN_POINT ( 'NONE',  ( 15.24356964374999990, 249.8218750006145399, -3.323476615752268604 ) ) ;
#1321=EDGE_CURVE ( 'NONE', #18637, #7872, #9377, .T. ) ;
#1322=CARTESIAN_POINT ( 'NONE',  ( 27.24356964375000700, 199.5968750006145740, 15.72908226750537075 ) ) ;
#1323=CARTESIAN_POINT ( 'NONE',  ( 2.999999999999997780, 244.5000000000000000, 2.500000000000000000 ) ) ;
#1326=CARTESIAN_POINT ( 'NONE',  ( 26.75643035624999655, 241.9843750006145342, -7.049594010296217766E-16 ) ) ;
#1331=ORIENTED_EDGE ( 'NONE', *, *, #25346, .T. ) ;
#1333=CARTESIAN_POINT ( 'NONE',  ( 21.00000000000000000, 247.8343750006144717, -6.646953231504538984 ) ) ;
#1338=VERTEX_POINT ( 'NONE', #20951 ) ;
#1345=CARTESIAN_POINT ( 'NONE',  ( 26.75643035624999655, 246.7843750006145171, 3.323476615752267271 ) ) ;
#1347=CARTESIAN_POINT ( 'NONE',  ( -26.99999999999999645, 199.2500000012290116, 15.58845726811991561 ) ) ;
#1358=CARTESIAN_POINT ( 'NONE',  ( 20.99999999999997513, 246.3437500012290684, -5.999999999999999112 ) ) ;
#1369=CARTESIAN_POINT ( 'NONE',  ( -26.99999999999998934, 196.4375000000000284, 15.58845726811991561 ) ) ;
#1374=EDGE_LOOP ( 'NONE', ( #17403, #25108, #14081, #5850 ) ) ;
#1376=CARTESIAN_POINT ( 'NONE',  ( 26.99999999999999645, 243.9437500012290343, 3.464101615137751278 ) ) ;
#1383=CARTESIAN_POINT ( 'NONE',  ( 23.87821517812499650, 245.0968750006145171, -4.985214923628404904 ) ) ;
#1388=DIRECTION ( 'NONE',  ( -0.000000000000000000, 1.000000000000000000, -0.000000000000000000 ) ) ;
#1393=CARTESIAN_POINT ( 'NONE',  ( -3.253724281355068545E-15, 196.2874999999999659, -27.00000000000000355 ) ) ;
#1400=CARTESIAN_POINT ( 'NONE',  ( -4.500000000000000888, 210.0000000000000284, 2.500000000000000000 ) ) ;
#1405=CARTESIAN_POINT ( 'NONE',  ( 1.069080835302379631E-14, 199.2125000000000057, 27.00000000000000000 ) ) ;
#1409=CARTESIAN_POINT ( 'NONE',  ( 15.24356964374999990, 248.9593750006145285, 0.000000000000000000 ) ) ;
#1411=CARTESIAN_POINT ( 'NONE',  ( 23.87821517812499650, 245.2093750006145569, -4.985214923628404904 ) ) ;
#1413=CARTESIAN_POINT ( 'NONE',  ( -29.00000000000002487, 210.0000000000000000, 0.000000000000000000 ) ) ;
#1422=ORIENTED_EDGE ( 'NONE', *, *, #30812, .T. ) ;
#1425=FACE_OUTER_BOUND ( 'NONE', #9140, .T. ) ;
#1431=AXIS2_PLACEMENT_3D ( 'NONE', #12225, #7297, #26816 ) ;
#1432=CARTESIAN_POINT ( 'NONE',  ( -4.694659320240884604E-14, 197.4124999999999943, 27.00000000000000000 ) ) ;
#1433=CARTESIAN_POINT ( 'NONE',  ( 19.39230484541326049, 243.6638461906613600, -5.999999999999997335 ) ) ;
#1441=CARTESIAN_POINT ( 'NONE',  ( 18.00000000000000355, 241.0750000000000171, 5.196152422706632912 ) ) ;
#1442=CARTESIAN_POINT ( 'NONE',  ( -1.926257025242585782E-15, 198.7906250006145399, -31.45816453501075927 ) ) ;
#1445=ORIENTED_EDGE ( 'NONE', *, *, #16238, .T. ) ;
#1448=CARTESIAN_POINT ( 'NONE',  ( -13.49999999999998401, 197.8249999999999886, 23.38268590217985476 ) ) ;
#1459=STYLED_ITEM('',(#37556),#33379);
#1466=ORIENTED_EDGE ( 'NONE', *, *, #32719, .T. ) ;
#1471=CARTESIAN_POINT ( 'NONE',  ( 18.00000000000000355, 245.1250000000000000, 5.196152422706632912 ) ) ;
#1477=CARTESIAN_POINT ( 'NONE',  ( -13.49999999999998401, 199.2875000012290627, 23.38268590217985476 ) ) ;
#1481=CARTESIAN_POINT ( 'NONE',  ( 26.75643035624999655, 244.6468750006145285, 3.323476615752267715 ) ) ;
#1487=EDGE_CURVE ( 'NONE', #21289, #23722, #29129, .T. ) ;
#1496=DIRECTION ( 'NONE',  ( -0.000000000000000000, 1.000000000000000000, -0.000000000000000000 ) ) ;
#1502=CARTESIAN_POINT ( 'NONE',  ( 15.24356964374999990, 240.7093750006145285, -3.323476615752268604 ) ) ;
#1507=CARTESIAN_POINT ( 'NONE',  ( -13.62178482187500528, 198.8843750006145399, -23.59362340125807123 ) ) ;
#1509=DIRECTION ( 'NONE',  ( 0.000000000000000000, 0.000000000000000000, 1.000000000000000000 ) ) ;
#1511=CARTESIAN_POINT ( 'NONE',  ( 15.24356964374999990, 244.0093750006145399, 0.000000000000000000 ) ) ;
#1516=CARTESIAN_POINT ( 'NONE',  ( 21.00000000000000000, 247.1593750006145171, 6.646953231504538984 ) ) ;
#1524=ORIENTED_EDGE ( 'NONE', *, *, #889, .T. ) ;
#1530=CARTESIAN_POINT ( 'NONE',  ( 15.24356964375000167, 247.5343750006144887, 3.323476615752272600 ) ) ;
#1533=EDGE_CURVE ( 'NONE', #6008, #20414, #27720, .T. ) ;
#1553=CARTESIAN_POINT ( 'NONE',  ( 10.49999999999999467, 215.7563705986615901, -5.555555555555558911 ) ) ;
#1554=CARTESIAN_POINT ( 'NONE',  ( 27.24356964375000700, 196.8968750006145285, 15.72908226750537075 ) ) ;
#1559=CARTESIAN_POINT ( 'NONE',  ( 26.99999999999999645, 243.4937500012290741, 3.464101615137751278 ) ) ;
#1562=CARTESIAN_POINT ( 'NONE',  ( 20.99999999999999645, 242.9687500012290684, 5.999999999999998224 ) ) ;
#1579=ADVANCED_FACE ( 'NONE', ( #30215 ), #27924, .F. ) ;
#1590=CARTESIAN_POINT ( 'NONE',  ( -28.86277965861013328, 202.5120511701786654, -2.828156894100585461 ) ) ;
#1597=CARTESIAN_POINT ( 'NONE',  ( -27.00000000000000355, 195.5000000000000000, 0.000000000000000000 ) ) ;
#1599=CARTESIAN_POINT ( 'NONE',  ( 21.00000000000000000, 247.4968750006145513, -6.646953231504538984 ) ) ;
#1601=CARTESIAN_POINT ( 'NONE',  ( 23.87821517812500005, 243.7093750006145285, 4.985214923628404016 ) ) ;
#1621=ADVANCED_FACE ( 'NONE', ( #36077 ), #7283, .F. ) ;
#1622=CARTESIAN_POINT ( 'NONE',  ( -13.49999999999998401, 197.3750000000000284, 23.38268590217985476 ) ) ;
#1623=CARTESIAN_POINT ( 'NONE',  ( 16.22935424640221669, 222.7217220096020469, 3.659938751166898374 ) ) ;
#1633=CARTESIAN_POINT ( 'NONE',  ( -27.24356964374999990, 196.1656250006145399, -15.72908226750537786 ) ) ;
#1660=CARTESIAN_POINT ( 'NONE',  ( 26.99999999999999645, 245.6875000000000000, 3.464101615137751278 ) ) ;
#1666=CARTESIAN_POINT ( 'NONE',  ( 13.49999999999999645, 199.0625000012290400, -23.38268590217984766 ) ) ;
#1667=CARTESIAN_POINT ( 'NONE',  ( -26.99999999999999645, 196.8875000000000171, 15.58845726811991561 ) ) ;
#1668=AXIS2_PLACEMENT_3D ( 'NONE', #15479, #33098, #18715 ) ;
#1671=CARTESIAN_POINT ( 'NONE',  ( 15.24356964374999990, 244.4218750006145058, -3.323476615752268604 ) ) ;
#1677=CARTESIAN_POINT ( 'NONE',  ( 20.99999999999999645, 240.1843750006145513, -6.646953231504538984 ) ) ;
#1689=CARTESIAN_POINT ( 'NONE',  ( 26.75643035624999655, 240.9718750006145171, -7.049594010296217766E-16 ) ) ;
#1690=ORIENTED_EDGE ( 'NONE', *, *, #33509, .F. ) ;
#1692=VECTOR ( 'NONE', #23370, 1000.000000000000000 ) ;
#1694=CARTESIAN_POINT ( 'NONE',  ( 5.778771075727756162E-15, 198.6218750006145513, 31.45816453501076637 ) ) ;
#1695=CARTESIAN_POINT ( 'NONE',  ( 20.99999999999999645, 185.0294372515228645, 0.000000000000000000 ) ) ;
#1697=CARTESIAN_POINT ( 'NONE',  ( 15.24356964374999990, 243.0718750006145115, -3.323476615752268604 ) ) ;
#1699=EDGE_CURVE ( 'NONE', #7705, #7058, #22066, .T. ) ;
#1704=CARTESIAN_POINT ( 'NONE',  ( 23.87821517812499650, 244.1968750006145115, -4.985214923628404904 ) ) ;
#1720=CARTESIAN_POINT ( 'NONE',  ( 26.75643035624999655, 247.2718750006145001, -7.049594010296217766E-16 ) ) ;
#1726=EDGE_CURVE ( 'NONE', #9537, #27444, #10675, .T. ) ;
#1741=( BOUNDED_CURVE ( )  B_SPLINE_CURVE ( 2, ( #21748, #9984, #1448, #6767, #30269, #15304, #18727, #13212, #12645 ),
 .UNSPECIFIED., .F., .F. ) 
 B_SPLINE_CURVE_WITH_KNOTS ( ( 3, 2, 2, 2, 3 ),
 ( 0.3958333333333333703, 0.4027777777777777901, 0.4166666666666666852, 0.4305555555555555802, 0.4375000000000000000 ),
 .UNSPECIFIED. ) 
 CURVE ( )  GEOMETRIC_REPRESENTATION_ITEM ( )  RATIONAL_B_SPLINE_CURVE ( ( 0.9330127018922194093, 0.9330127018922196314, 1.000000000000000000, 0.8660254037844387076, 1.000000000000000000, 0.8660254037844387076, 1.000000000000000000, 0.9330127018922194093, 0.9330127018922194093 ) ) 
 REPRESENTATION_ITEM ( '' )  );
#1743=CARTESIAN_POINT ( 'NONE',  ( -27.24356964374999635, 198.5468750006145626, 15.72908226750539384 ) ) ;
#1745=CARTESIAN_POINT ( 'NONE',  ( 24.00000000000000000, 243.8500000000000227, 5.196152422706629359 ) ) ;
#1748=ORIENTED_EDGE ( 'NONE', *, *, #10047, .T. ) ;
#1749=CARTESIAN_POINT ( 'NONE',  ( 23.99999999999999645, 241.3562500012290286, -5.196152422706631135 ) ) ;
#1753=CARTESIAN_POINT ( 'NONE',  ( 5.778771075727756162E-15, 199.4656250006145797, 31.45816453501075927 ) ) ;
#1769=CARTESIAN_POINT ( 'NONE',  ( -12.83399793243727238, 216.5739059620414082, -4.792798303949182603 ) ) ;
#1776=EDGE_CURVE ( 'NONE', #14300, #10569, #1955, .T. ) ;
#1785=CARTESIAN_POINT ( 'NONE',  ( 21.00000000000000000, 247.0468750006145058, -6.646953231504538984 ) ) ;
#1787=CARTESIAN_POINT ( 'NONE',  ( 26.75643035624999655, 243.2968750006145342, 3.323476615752267271 ) ) ;
#1790=CARTESIAN_POINT ( 'NONE',  ( 15.00000000000000000, 248.7062500012290229, 0.000000000000000000 ) ) ;
#1803=CARTESIAN_POINT ( 'NONE',  ( 19.39230484541326760, 242.0486538117967257, 5.999999999999999112 ) ) ;
#1808=CARTESIAN_POINT ( 'NONE',  ( 15.61591388112558398, 224.3575629836673500, -2.655215585728295302 ) ) ;
#1810=DIRECTION ( 'NONE',  ( -0.000000000000000000, 1.000000000000000000, -0.000000000000000000 ) ) ;
#1817=CARTESIAN_POINT ( 'NONE',  ( -27.24356964374999635, 196.2406250006145285, 15.72908226750539384 ) ) ;
#1820=EDGE_LOOP ( 'NONE', ( #14528, #16312, #11727, #22043 ) ) ;
#1821=DIRECTION ( 'NONE',  ( 0.000000000000000000, 0.000000000000000000, -1.000000000000000000 ) ) ;
#1840=CARTESIAN_POINT ( 'NONE',  ( 19.39230484541326760, 241.9924038105676800, 5.999999999999999112 ) ) ;
#1845=CARTESIAN_POINT ( 'NONE',  ( 26.99999999999999645, 246.2125000000000057, -3.464101615137755275 ) ) ;
#1852=CARTESIAN_POINT ( 'NONE',  ( 13.49999999999999645, 197.2625000012290286, -23.38268590217984766 ) ) ;
#1853=CARTESIAN_POINT ( 'NONE',  ( -13.50000000000000533, 196.7750000000000057, -23.38268590217984411 ) ) ;
#1856=CARTESIAN_POINT ( 'NONE',  ( 23.87821517812499650, 244.7593750006145399, -4.985214923628404904 ) ) ;
#1862=CARTESIAN_POINT ( 'NONE',  ( 13.62178482187499640, 197.9093750006145456, -23.59362340125807123 ) ) ;
#1867=CARTESIAN_POINT ( 'NONE',  ( 18.00000000000000355, 247.3750000000000000, 5.196152422706632912 ) ) ;
#1879=ORIENTED_EDGE ( 'NONE', *, *, #30260, .F. ) ;
#1882=CARTESIAN_POINT ( 'NONE',  ( 27.24356964375000345, 197.3843750006145399, -3.336375036156643733E-15 ) ) ;
#1886=CARTESIAN_POINT ( 'NONE',  ( 21.00000000000000000, 243.4468750006145683, -6.646953231504538984 ) ) ;
#1892=CARTESIAN_POINT ( 'NONE',  ( 26.75643035624999655, 245.4718750006145171, -7.049594010296217766E-16 ) ) ;
#1896=CARTESIAN_POINT ( 'NONE',  ( 26.99999999999999645, 244.3750000000000000, -7.347880794884117764E-16 ) ) ;
#1905=CARTESIAN_POINT ( 'NONE',  ( 23.87821517812499650, 243.7468750006145228, -4.985214923628404904 ) ) ;
#1906=DIRECTION ( 'NONE',  ( 1.000000000000000000, 0.000000000000000000, 0.000000000000000000 ) ) ;
#1909=EDGE_CURVE ( 'NONE', #28735, #6593, #13629, .T. ) ;
#1912=CARTESIAN_POINT ( 'NONE',  ( 20.99999999999999289, 245.4437500012290343, -5.999999999999997335 ) ) ;
#1925=CARTESIAN_POINT ( 'NONE',  ( 27.24356964375000345, 199.1843750006145228, -3.336375036156643733E-15 ) ) ;
#1926=CARTESIAN_POINT ( 'NONE',  ( -29.00000000000002487, 210.0000000000000000, 0.000000000000000000 ) ) ;
#1927=CARTESIAN_POINT ( 'NONE',  ( 26.99999999999999645, 242.0875000000000057, 3.464101615137751278 ) ) ;
#1932=CARTESIAN_POINT ( 'NONE',  ( 18.00000000000000355, 242.4812500012290570, 5.196152422706632912 ) ) ;
#1935=CARTESIAN_POINT ( 'NONE',  ( 27.24356964374999635, 198.2656250006145058, -15.72908226750539029 ) ) ;
#1944=CARTESIAN_POINT ( 'NONE',  ( -3.253724281355068545E-15, 197.3000000012290229, -27.00000000000000355 ) ) ;
#1948=EDGE_CURVE ( 'NONE', #16763, #28735, #10973, .T. ) ;
#1955=LINE ( 'NONE', #28988, #36989 ) ;
#1959=CARTESIAN_POINT ( 'NONE',  ( 20.99999999999997868, 246.9625000000000057, 5.999999999999999112 ) ) ;
#1962=CARTESIAN_POINT ( 'NONE',  ( -13.50000000000000533, 195.9875000012290229, -23.38268590217984411 ) ) ;
#1968=CARTESIAN_POINT ( 'NONE',  ( 23.87821517812499650, 246.5593750006145228, -4.985214923628404904 ) ) ;
#1970=CARTESIAN_POINT ( 'NONE',  ( 15.24356964375000167, 243.5968750006144887, 3.323476615752272600 ) ) ;
#1973=EDGE_CURVE ( 'NONE', #30190, #35202, #32023, .T. ) ;
#1974=CARTESIAN_POINT ( 'NONE',  ( 18.00000000000000355, 248.7812500012290400, 5.196152422706632912 ) ) ;
#1980=AXIS2_PLACEMENT_3D ( 'NONE', #7089, #18659, #4225 ) ;
#1987=CYLINDRICAL_SURFACE ( 'NONE', #10033, 27.00000000000000000 ) ;
#1989=CARTESIAN_POINT ( 'NONE',  ( 15.24356964374999990, 248.8468750006145171, 0.000000000000000000 ) ) ;
#1993=CARTESIAN_POINT ( 'NONE',  ( 15.20136072254650372, 225.4630380732105550, -1.553813268098525935 ) ) ;
#1995=CARTESIAN_POINT ( 'NONE',  ( 20.99999999999999645, 185.0294372515228645, 5.999999999999999112 ) ) ;
#2002=CARTESIAN_POINT ( 'NONE',  ( -1.926257025242585782E-15, 196.9906250006145569, -31.45816453501075927 ) ) ;
#2006=DIRECTION ( 'NONE',  ( -1.000000000000000000, -6.123233995736766036E-17, 0.000000000000000000 ) ) ;
#2012=AXIS2_PLACEMENT_3D ( 'NONE', #21693, #33244, #1205 ) ;
#2019=CARTESIAN_POINT ( 'NONE',  ( 13.50000000000001421, 198.3499999999999943, 23.38268590217984055 ) ) ;
#2023=CARTESIAN_POINT ( 'NONE',  ( 27.00000000000001421, 198.5000000012290684, 15.58845726811988897 ) ) ;
#2024=ORIENTED_EDGE ( 'NONE', *, *, #23373, .F. ) ;
#2026=( BOUNDED_CURVE ( )  B_SPLINE_CURVE ( 2, ( #36868, #8629, #22677, #14501, #31560, #34036, #13771, #7894, #14135 ),
 .UNSPECIFIED., .F., .F. ) 
 B_SPLINE_CURVE_WITH_KNOTS ( ( 3, 2, 2, 2, 3 ),
 ( 0.05434782608695652717, 0.05797101449275362389, 0.06521739130434782428, 0.07246376811594203160, 0.07608695652173913526 ),
 .UNSPECIFIED. ) 
 CURVE ( )  GEOMETRIC_REPRESENTATION_ITEM ( )  RATIONAL_B_SPLINE_CURVE ( ( 0.9330127018922194093, 0.9330127018922194093, 1.000000000000000000, 0.8660254037844387076, 1.000000000000000000, 0.8660254037844387076, 1.000000000000000000, 0.9330127018922191873, 0.9330127018922192983 ) ) 
 REPRESENTATION_ITEM ( '' )  );
#2031=CARTESIAN_POINT ( 'NONE',  ( 24.00000000000000000, 242.5000000000000000, 5.196152422706629359 ) ) ;
#2036=ORIENTED_EDGE ( 'NONE', *, *, #21240, .F. ) ;
#2037=CARTESIAN_POINT ( 'NONE',  ( 27.00000000000000355, 197.1875000012290400, -3.306546357697854128E-15 ) ) ;
#2041=CARTESIAN_POINT ( 'NONE',  ( 15.24356964374999990, 243.1093750006145342, 0.000000000000000000 ) ) ;
#2048=CARTESIAN_POINT ( 'NONE',  ( -1.926257025242585782E-15, 198.3968750006145285, -31.45816453501075927 ) ) ;
#2054=EDGE_CURVE ( 'NONE', #32985, #22802, #12313, .T. ) ;
#2066=CARTESIAN_POINT ( 'NONE',  ( 22.60769515458673240, 248.3888461906613543, 6.000000000000000000 ) ) ;
#2070=CARTESIAN_POINT ( 'NONE',  ( -13.62178482187498396, 198.5843750006145569, 23.59362340125808188 ) ) ;
#2072=( BOUNDED_CURVE ( )  B_SPLINE_CURVE ( 2, ( #2525, #25644, #36454, #34361, #8407, #24903, #1962, #36644, #3266 ),
 .UNSPECIFIED., .F., .F. ) 
 B_SPLINE_CURVE_WITH_KNOTS ( ( 3, 2, 2, 2, 3 ),
 ( 0.6458333333333333703, 0.6527777777777777901, 0.6666666666666666297, 0.6805555555555555802, 0.6875000000000000000 ),
 .UNSPECIFIED. ) 
 CURVE ( )  GEOMETRIC_REPRESENTATION_ITEM ( )  RATIONAL_B_SPLINE_CURVE ( ( 0.9330127018922192983, 0.9330127018922198534, 1.000000000000000000, 0.8660254037844387076, 1.000000000000000000, 0.8660254037844387076, 1.000000000000000000, 0.9330127018922194093, 0.9330127018922194093 ) ) 
 REPRESENTATION_ITEM ( '' )  );
#2075=CARTESIAN_POINT ( 'NONE',  ( 26.99999999999999645, 249.7750000000000057, -7.347880794884117764E-16 ) ) ;
#2082=CARTESIAN_POINT ( 'NONE',  ( 21.00000000000000000, 245.3593750006145342, 6.646953231504538984 ) ) ;
#2087=CARTESIAN_POINT ( 'NONE',  ( 20.99999999999999645, 244.2624999999999602, 5.999999999999998224 ) ) ;
#2095=CARTESIAN_POINT ( 'NONE',  ( 15.24356964374999990, 244.3093750006144944, -3.323476615752268604 ) ) ;
#2096=CARTESIAN_POINT ( 'NONE',  ( -4.694659320240884604E-14, 197.5250000012290172, 27.00000000000000000 ) ) ;
#2110=CYLINDRICAL_SURFACE ( 'NONE', #30301, 5.999999999999999112 ) ;
#2112=CARTESIAN_POINT ( 'NONE',  ( 18.00000000000000355, 246.9812500012290570, 5.196152422706632912 ) ) ;
#2113=CARTESIAN_POINT ( 'NONE',  ( -27.24356964374999635, 197.1968750006145115, 15.72908226750539384 ) ) ;
#2115=CARTESIAN_POINT ( 'NONE',  ( 21.00000000000000000, 242.0124999999999886, 5.999999999999998224 ) ) ;
#2118=VERTEX_POINT ( 'NONE', #15541 ) ;
#2119=CARTESIAN_POINT ( 'NONE',  ( 26.99999999999999645, 242.2187500012290684, -3.464101615137755275 ) ) ;
#2122=CARTESIAN_POINT ( 'NONE',  ( -27.24356964374999635, 198.9406250006145171, 15.72908226750539384 ) ) ;
#2133=CARTESIAN_POINT ( 'NONE',  ( -26.99999999999999645, 196.4375000000000284, 15.58845726811991561 ) ) ;
#2138=DIRECTION ( 'NONE',  ( 0.000000000000000000, 0.000000000000000000, 1.000000000000000000 ) ) ;
#2146=VERTEX_POINT ( 'NONE', #35428 ) ;
#2154=CARTESIAN_POINT ( 'NONE',  ( 21.00000000000000000, 247.7218750006145171, 6.646953231504538984 ) ) ;
#2156=CARTESIAN_POINT ( 'NONE',  ( 23.87821517812499650, 242.5093750006145399, -4.985214923628404904 ) ) ;
#2158=CYLINDRICAL_SURFACE ( 'NONE', #6659, 5.999999999999999112 ) ;
#2159=CARTESIAN_POINT ( 'NONE',  ( 24.00000000000000000, 247.9562500012290229, 5.196152422706629359 ) ) ;
#2166=VERTEX_POINT ( 'NONE', #35239 ) ;
#2167=VERTEX_POINT ( 'NONE', #29940 ) ;
#2173=CARTESIAN_POINT ( 'NONE',  ( 18.12178482187500350, 248.0218750006145001, 4.985214923628407568 ) ) ;
#2177=CARTESIAN_POINT ( 'NONE',  ( 15.38158308873944158, 224.9824450966943346, -2.114697272284929763 ) ) ;
#2183=ADVANCED_FACE ( 'NONE', ( #24261 ), #18015, .T. ) ;
#2185=CARTESIAN_POINT ( 'NONE',  ( -13.62178482187498396, 197.1781250006145569, 23.59362340125808188 ) ) ;
#2189=VERTEX_POINT ( 'NONE', #21239 ) ;
#2204=CARTESIAN_POINT ( 'NONE',  ( 26.99999999999999645, 197.5624999999999716, -15.58845726811990495 ) ) ;
#2208=CARTESIAN_POINT ( 'NONE',  ( 15.24356964375000167, 248.9968750006145513, 3.323476615752272600 ) ) ;
#2215=CARTESIAN_POINT ( 'NONE',  ( 21.00000000000000000, 244.4874999999999829, -6.928203230275506996 ) ) ;
#2216=CARTESIAN_POINT ( 'NONE',  ( 1.069080835302379631E-14, 195.6124999999999829, 27.00000000000000000 ) ) ;
#2220=CARTESIAN_POINT ( 'NONE',  ( 13.49999999999999645, 196.8125000012290400, -23.38268590217984766 ) ) ;
#2226=CARTESIAN_POINT ( 'NONE',  ( 21.00000000000000000, 242.0968750006145456, -6.646953231504538984 ) ) ;
#2228=VECTOR ( 'NONE', #19325, 1000.000000000000000 ) ;
#2229=CARTESIAN_POINT ( 'NONE',  ( 20.00041244883536606, 239.7473985345926053, -5.668978318349186196 ) ) ;
#2234=CARTESIAN_POINT ( 'NONE',  ( -13.62178482187498396, 199.0343750006145456, 23.59362340125808188 ) ) ;
#2249=CARTESIAN_POINT ( 'NONE',  ( 26.99999999999999645, 248.5187500012290513, -3.464101615137755275 ) ) ;
#2250=ORIENTED_EDGE ( 'NONE', *, *, #33561, .F. ) ;
#2253=AXIS2_PLACEMENT_3D ( 'NONE', #35133, #26231, #3115 ) ;
#2254=CARTESIAN_POINT ( 'NONE',  ( 13.62178482187501416, 197.7593750006145399, 23.59362340125806767 ) ) ;
#2258=CARTESIAN_POINT ( 'NONE',  ( 26.75643035624999655, 241.0468750006145058, 3.323476615752267715 ) ) ;
#2259=DIRECTION ( 'NONE',  ( 0.000000000000000000, 0.000000000000000000, -1.000000000000000000 ) ) ;
#2264=CARTESIAN_POINT ( 'NONE',  ( 15.24356964374999990, 244.3468750006145171, 0.000000000000000000 ) ) ;
#2278=CARTESIAN_POINT ( 'NONE',  ( 20.99999999999999645, 243.7843750006145171, -6.646953231504538984 ) ) ;
#2285=DIRECTION ( 'NONE',  ( -0.000000000000000000, -1.000000000000000000, -0.000000000000000000 ) ) ;
#2295=CARTESIAN_POINT ( 'NONE',  ( 20.99999999999999645, 185.0294372515228645, 0.000000000000000000 ) ) ;
#2300=CARTESIAN_POINT ( 'NONE',  ( -13.62178482187498396, 197.6843750006145228, 23.59362340125808188 ) ) ;
#2301=EDGE_CURVE ( 'NONE', #8916, #12071, #18778, .T. ) ;
#2307=ORIENTED_EDGE ( 'NONE', *, *, #11411, .F. ) ;
#2309=CARTESIAN_POINT ( 'NONE',  ( 23.99999999999999645, 240.9062500012290684, -5.196152422706631135 ) ) ;
#2317=AXIS2_PLACEMENT_3D ( 'NONE', #21030, #26883, #32566 ) ;
#2329=CARTESIAN_POINT ( 'NONE',  ( -28.81129111113878594, 202.7130252932614383, 3.311965150308325612 ) ) ;
#2342=CARTESIAN_POINT ( 'NONE',  ( -3.253724281355068545E-15, 198.9874999999999829, -27.00000000000000000 ) ) ;
#2346=CARTESIAN_POINT ( 'NONE',  ( 18.12178482187499640, 247.9843750006145342, -4.985214923628404904 ) ) ;
#2348=CARTESIAN_POINT ( 'NONE',  ( 20.99999999999999645, 242.5468750006145342, -6.646953231504538984 ) ) ;
#2349=ORIENTED_EDGE ( 'NONE', *, *, #7960, .F. ) ;
#2363=FACE_OUTER_BOUND ( 'NONE', #30294, .T. ) ;
#2364=CARTESIAN_POINT ( 'NONE',  ( 21.00000000000000000, 249.6343750006145399, -6.646953231504538984 ) ) ;
#2367=CARTESIAN_POINT ( 'NONE',  ( 5.205286459873386562, 215.9230175775471423, -0.9779651927395711652 ) ) ;
#2369=CARTESIAN_POINT ( 'NONE',  ( 1.120210788295102201E-13, 197.1875000000000568, -27.00000000000000711 ) ) ;
#2375=CARTESIAN_POINT ( 'NONE',  ( 13.62178482187499640, 196.5031250006145456, -23.59362340125807123 ) ) ;
#2379=CARTESIAN_POINT ( 'NONE',  ( 20.99999999999999289, 240.8874999999999886, -5.999999999999997335 ) ) ;
#2392=CARTESIAN_POINT ( 'NONE',  ( -1.909035429704832693E-15, 198.0875000000000341, -31.17691453623979214 ) ) ;
#2393=CYLINDRICAL_SURFACE ( 'NONE', #17194, 5.999999999999999112 ) ;
#2396=CARTESIAN_POINT ( 'NONE',  ( 15.24356964375000167, 249.4468750006144830, 3.323476615752272600 ) ) ;
#2397=ORIENTED_EDGE ( 'NONE', *, *, #35638, .F. ) ;
#2402=CARTESIAN_POINT ( 'NONE',  ( 18.00000000000000000, 244.5250000000000057, -5.196152422706630247 ) ) ;
#2407=VERTEX_POINT ( 'NONE', #6535 ) ;
#2408=CARTESIAN_POINT ( 'NONE',  ( -13.49999999999998401, 196.1375000012290286, 23.38268590217985476 ) ) ;
#2413=CARTESIAN_POINT ( 'NONE',  ( 23.87821517812500005, 241.9093750006145456, 4.985214923628404016 ) ) ;
#2421=CARTESIAN_POINT ( 'NONE',  ( -27.24356964374999990, 197.5718750006145399, -15.72908226750537786 ) ) ;
#2427=CARTESIAN_POINT ( 'NONE',  ( 20.99999999999999289, 242.2374999999999545, -5.999999999999997335 ) ) ;
#2430=AXIS2_PLACEMENT_3D ( 'NONE', #11023, #32038, #6068 ) ;
#2434=CARTESIAN_POINT ( 'NONE',  ( 22.60769515458672885, 248.9674038105676459, -5.999999999999998224 ) ) ;
#2439=CARTESIAN_POINT ( 'NONE',  ( -1.045839947578415010E-13, 196.0625000000000284, 27.00000000000000355 ) ) ;
#2440=EDGE_CURVE ( 'NONE', #17126, #14209, #3309, .T. ) ;
#2443=CARTESIAN_POINT ( 'NONE',  ( 1.069080835302379631E-14, 198.3124999999999716, 27.00000000000000000 ) ) ;
#2444=CARTESIAN_POINT ( 'NONE',  ( 18.12178482187499640, 241.2343750006145342, -4.985214923628404904 ) ) ;
#2445=CARTESIAN_POINT ( 'NONE',  ( -27.24356964375000345, 198.9031250006145228, 0.000000000000000000 ) ) ;
#2451=CARTESIAN_POINT ( 'NONE',  ( 23.87821517812499650, 243.2968750006145058, -4.985214923628404904 ) ) ;
#2452=EDGE_CURVE ( 'NONE', #25376, #8033, #29837, .T. ) ;
#2461=ADVANCED_FACE ( 'NONE', ( #21331 ), #11842, .F. ) ;
#2463=CARTESIAN_POINT ( 'NONE',  ( 20.99999999999999645, 243.5593750006144944, 6.646953231504538984 ) ) ;
#2475=CARTESIAN_POINT ( 'NONE',  ( 22.60769515458672885, 244.5236538117967200, -5.999999999999998224 ) ) ;
#2479=ORIENTED_EDGE ( 'NONE', *, *, #2440, .F. ) ;
#2483=DIRECTION ( 'NONE',  ( 0.000000000000000000, 0.000000000000000000, 1.000000000000000000 ) ) ;
#2484=CARTESIAN_POINT ( 'NONE',  ( -1.926257025242585782E-15, 195.2468750006145513, -31.45816453501075927 ) ) ;
#2488=DIRECTION ( 'NONE',  ( -0.000000000000000000, -1.000000000000000000, -0.000000000000000000 ) ) ;
#2490=CARTESIAN_POINT ( 'NONE',  ( 15.00000000000000000, 242.4062500012290400, 0.000000000000000000 ) ) ;
#2495=AXIS2_PLACEMENT_3D ( 'NONE', #12120, #9663, #15162 ) ;
#2496=ORIENTED_EDGE ( 'NONE', *, *, #19625, .T. ) ;
#2504=EDGE_CURVE ( 'NONE', #13411, #31515, #16569, .T. ) ;
#2507=EDGE_CURVE ( 'NONE', #149, #36238, #24352, .T. ) ;
#2511=CARTESIAN_POINT ( 'NONE',  ( 1.069080835302379631E-14, 197.9750000012290343, 27.00000000000000000 ) ) ;
#2517=EDGE_CURVE ( 'NONE', #18936, #37055, #3453, .T. ) ;
#2525=CARTESIAN_POINT ( 'NONE',  ( -1.045839947578415010E-13, 196.1750000012290229, 27.00000000000000355 ) ) ;
#2530=CARTESIAN_POINT ( 'NONE',  ( 20.99999999999999645, 250.0000000000000000, 5.999999999999999112 ) ) ;
#2531=( BOUNDED_CURVE ( )  B_SPLINE_CURVE ( 2, ( #12084, #1086, #27060, #1270, #30091, #29707, #24408, #4496, #897 ),
 .UNSPECIFIED., .F., .F. ) 
 B_SPLINE_CURVE_WITH_KNOTS ( ( 3, 2, 2, 2, 3 ),
 ( 0.1847826086956521618, 0.1884057971014492794, 0.1956521739130434867, 0.2028985507246376940, 0.2065217391304347838 ),
 .UNSPECIFIED. ) 
 CURVE ( )  GEOMETRIC_REPRESENTATION_ITEM ( )  RATIONAL_B_SPLINE_CURVE ( ( 0.9330127018922194093, 0.9330127018922190762, 1.000000000000000000, 0.8660254037844387076, 1.000000000000000000, 0.8660254037844387076, 1.000000000000000000, 0.9330127018922194093, 0.9330127018922194093 ) ) 
 REPRESENTATION_ITEM ( '' )  );
#2532=CARTESIAN_POINT ( 'NONE',  ( 15.24356964375000167, 244.4968750006145228, 3.323476615752272600 ) ) ;
#2534=CARTESIAN_POINT ( 'NONE',  ( 26.75643035624999655, 241.5718750006145399, -3.323476615752271268 ) ) ;
#2538=CARTESIAN_POINT ( 'NONE',  ( 18.00000000000000355, 249.2312500012290570, 5.196152422706632912 ) ) ;
#2551=CARTESIAN_POINT ( 'NONE',  ( 26.75643035624999655, 248.1343750006145115, 3.323476615752267715 ) ) ;
#2554=CARTESIAN_POINT ( 'NONE',  ( 4.999999999999997335, 215.9999999999999716, 0.1963495407219033040 ) ) ;
#2571=( BOUNDED_CURVE ( )  B_SPLINE_CURVE ( 2, ( #3457, #27152, #12370, #29227, #32263, #20914, #421, #23939, #15026 ),
 .UNSPECIFIED., .F., .F. ) 
 B_SPLINE_CURVE_WITH_KNOTS ( ( 3, 2, 2, 2, 3 ),
 ( 0.6875000000000000000, 0.6944444444444444198, 0.7083333333333333703, 0.7222222222222222099, 0.7291666666666667407 ),
 .UNSPECIFIED. ) 
 CURVE ( )  GEOMETRIC_REPRESENTATION_ITEM ( )  RATIONAL_B_SPLINE_CURVE ( ( 0.9330127018922194093, 0.9330127018922194093, 1.000000000000000000, 0.8660254037844387076, 1.000000000000000000, 0.8660254037844387076, 1.000000000000000000, 0.9330127018922187432, 0.9330127018922192983 ) ) 
 REPRESENTATION_ITEM ( '' )  );
#2576=VECTOR ( 'NONE', #17244, 1000.000000000000000 ) ;
#2579=CARTESIAN_POINT ( 'NONE',  ( 26.99999999999999645, 198.0125000000000455, -15.58845726811990495 ) ) ;
#2581=CARTESIAN_POINT ( 'NONE',  ( 26.75643035624999655, 248.7718750006145001, -3.323476615752271268 ) ) ;
#2584=CARTESIAN_POINT ( 'NONE',  ( 23.99999999999999645, 243.5499999999999829, -5.196152422706631135 ) ) ;
#2588=CARTESIAN_POINT ( 'NONE',  ( 15.00000000000000000, 243.2500000000000000, 0.000000000000000000 ) ) ;
#2593=CARTESIAN_POINT ( 'NONE',  ( -27.00000000000000355, 196.9250000012290229, -15.58845726811989429 ) ) ;
#2597=CARTESIAN_POINT ( 'NONE',  ( 23.87821517812500005, 243.2593750006145399, 4.985214923628404016 ) ) ;
#2603=CARTESIAN_POINT ( 'NONE',  ( 27.10290335425204233, 195.0000000000000000, -0.6671862432530482057 ) ) ;
#2604=CARTESIAN_POINT ( 'NONE',  ( -27.24356964374999990, 199.3718750006145513, -15.72908226750537786 ) ) ;
#2609=CARTESIAN_POINT ( 'NONE',  ( 23.99999999999999645, 245.3500000000000227, -5.196152422706631135 ) ) ;
#2613=DIRECTION ( 'NONE',  ( 0.000000000000000000, 0.000000000000000000, -1.000000000000000000 ) ) ;
#2617=CARTESIAN_POINT ( 'NONE',  ( 22.60769515458673595, 249.8674038105676516, -6.000000000000000000 ) ) ;
#2618=DIRECTION ( 'NONE',  ( -0.000000000000000000, 1.000000000000000000, -0.000000000000000000 ) ) ;
#2622=CARTESIAN_POINT ( 'NONE',  ( -7.946041369334237991, 195.0000000000000000, 26.05901981062767092 ) ) ;
#2626=CARTESIAN_POINT ( 'NONE',  ( 26.99999999999999645, 249.7374999999999829, 3.464101615137751278 ) ) ;
#2627=CARTESIAN_POINT ( 'NONE',  ( -1.926257025242585782E-15, 199.6906250006145456, -31.45816453501076637 ) ) ;
#2632=CARTESIAN_POINT ( 'NONE',  ( 23.87821517812500005, 241.3468750006145171, 4.985214923628404016 ) ) ;
#2643=CARTESIAN_POINT ( 'NONE',  ( 15.24356964375000167, 243.4843750006145058, 3.323476615752272600 ) ) ;
#2650=CARTESIAN_POINT ( 'NONE',  ( -7.234628195640302017, 198.8549038117967029, 27.00000000000000711 ) ) ;
#2652=EDGE_CURVE ( 'NONE', #21280, #24290, #22616, .T. ) ;
#2659=ORIENTED_EDGE ( 'NONE', *, *, #22083, .T. ) ;
#2664=CARTESIAN_POINT ( 'NONE',  ( 22.60769515458672885, 243.8888461906613543, 5.999999999999997335 ) ) ;
#2667=CARTESIAN_POINT ( 'NONE',  ( -13.62178482187498396, 195.8843750006145399, 23.59362340125808188 ) ) ;
#2673=ORIENTED_EDGE ( 'NONE', *, *, #581, .F. ) ;
#2674=VERTEX_POINT ( 'NONE', #1959 ) ;
#2675=CARTESIAN_POINT ( 'NONE',  ( 26.75643035624999655, 249.0718750006145115, -7.049594010296217766E-16 ) ) ;
#2688=CARTESIAN_POINT ( 'NONE',  ( -18.84057396323613176, 195.0000000000000000, 19.60903927252854118 ) ) ;
#2708=CARTESIAN_POINT ( 'NONE',  ( 15.24356964375000167, 245.8468750006145171, 3.323476615752272600 ) ) ;
#2710=CARTESIAN_POINT ( 'NONE',  ( 20.99999999999999645, 240.9718750006145456, 6.646953231504538984 ) ) ;
#2711=VERTEX_POINT ( 'NONE', #28480 ) ;
#2712=DIRECTION ( 'NONE',  ( 0.000000000000000000, 0.000000000000000000, 1.000000000000000000 ) ) ;
#2714=CARTESIAN_POINT ( 'NONE',  ( 21.00000000000000000, 245.6687500012290570, 6.928203230275506996 ) ) ;
#2715=ORIENTED_EDGE ( 'NONE', *, *, #2992, .F. ) ;
#2723=ORIENTED_EDGE ( 'NONE', *, *, #30417, .T. ) ;
#2735=CARTESIAN_POINT ( 'NONE',  ( 17.03503949639525317, 220.5732280096082150, -4.520320870633828036 ) ) ;
#2745=AXIS2_PLACEMENT_3D ( 'NONE', #12131, #34882, #9488 ) ;
#2746=VERTEX_POINT ( 'NONE', #16751 ) ;
#2752=( BOUNDED_CURVE ( )  B_SPLINE_CURVE ( 2, ( #3093, #17700, #34931, #3280, #8976, #14661, #11625, #23200, #20925 ),
 .UNSPECIFIED., .F., .F. ) 
 B_SPLINE_CURVE_WITH_KNOTS ( ( 3, 2, 2, 2, 3 ),
 ( 0.2708333333333333703, 0.2777777777777777901, 0.2916666666666666852, 0.3055555555555555802, 0.3125000000000000000 ),
 .UNSPECIFIED. ) 
 CURVE ( )  GEOMETRIC_REPRESENTATION_ITEM ( )  RATIONAL_B_SPLINE_CURVE ( ( 0.9330127018922194093, 0.9330127018922196314, 1.000000000000000000, 0.8660254037844387076, 1.000000000000000000, 0.8660254037844387076, 1.000000000000000000, 0.9330127018922194093, 0.9330127018922194093 ) ) 
 REPRESENTATION_ITEM ( '' )  );
#2758=CARTESIAN_POINT ( 'NONE',  ( 18.00000000000000355, 243.3812500012290343, 5.196152422706632912 ) ) ;
#2760=CARTESIAN_POINT ( 'NONE',  ( 27.00000000000001066, 197.4875000000000114, 15.58845726811988897 ) ) ;
#2763=CARTESIAN_POINT ( 'NONE',  ( 15.24356964375000167, 248.0968750006145456, 3.323476615752272600 ) ) ;
#2770=CARTESIAN_POINT ( 'NONE',  ( 21.00000000000000000, 240.8875000000000171, -6.928203230275506996 ) ) ;
#2771=EDGE_CURVE ( 'NONE', #31898, #11836, #30370, .T. ) ;
#2777=CARTESIAN_POINT ( 'NONE',  ( 13.49999999999999645, 195.9125000012290343, -23.38268590217984766 ) ) ;
#2782=CARTESIAN_POINT ( 'NONE',  ( 23.87821517812500005, 243.7093750006145285, 4.985214923628404016 ) ) ;
#2789=CARTESIAN_POINT ( 'NONE',  ( 17.55485740163879527, 195.0000000000000000, 20.80657516995691836 ) ) ;
#2790=CARTESIAN_POINT ( 'NONE',  ( -13.62178482187498396, 196.3343750006145285, 23.59362340125808188 ) ) ;
#2792=( BOUNDED_CURVE ( )  B_SPLINE_CURVE ( 2, ( #25036, #28068, #36593, #19750, #10633, #31109, #13862, #25410, #22580 ),
 .UNSPECIFIED., .F., .F. ) 
 B_SPLINE_CURVE_WITH_KNOTS ( ( 3, 2, 2, 2, 3 ),
 ( 0.06250000000000000000, 0.06944444444444444753, 0.08333333333333332871, 0.09722222222222222376, 0.1041666666666666713 ),
 .UNSPECIFIED. ) 
 CURVE ( )  GEOMETRIC_REPRESENTATION_ITEM ( )  RATIONAL_B_SPLINE_CURVE ( ( 0.9330127018922194093, 0.9330127018922194093, 1.000000000000000000, 0.8660254037844387076, 1.000000000000000000, 0.8660254037844387076, 1.000000000000000000, 0.9330127018922192983, 0.9330127018922194093 ) ) 
 REPRESENTATION_ITEM ( '' )  );
#2794=ORIENTED_EDGE ( 'NONE', *, *, #25444, .T. ) ;
#2796=CARTESIAN_POINT ( 'NONE',  ( -4.694659320240884604E-14, 197.8625000000000114, 27.00000000000000000 ) ) ;
#2797=LINE ( 'NONE', #14369, #8396 ) ;
#2803=CARTESIAN_POINT ( 'NONE',  ( 0.000000000000000000, 210.0000000000000284, 0.000000000000000000 ) ) ;
#2807=CARTESIAN_POINT ( 'NONE',  ( -7.234628195640302017, 195.2549038117967086, 27.00000000000000711 ) ) ;
#2811=CARTESIAN_POINT ( 'NONE',  ( -27.24356964375000345, 195.3218750006145399, -15.72908226750537786 ) ) ;
#2814=DIRECTION ( 'NONE',  ( 0.000000000000000000, 0.000000000000000000, 1.000000000000000000 ) ) ;
#2815=CARTESIAN_POINT ( 'NONE',  ( 21.00000000000000000, 240.9718750006145456, 6.646953231504538984 ) ) ;
#2816=CARTESIAN_POINT ( 'NONE',  ( 5.778771075727756162E-15, 199.0156250006145342, 31.45816453501076637 ) ) ;
#2819=ORIENTED_EDGE ( 'NONE', *, *, #13347, .T. ) ;
#2821=CARTESIAN_POINT ( 'NONE',  ( 5.778771075727756162E-15, 197.2156250006145513, 31.45816453501075927 ) ) ;
#2822=CARTESIAN_POINT ( 'NONE',  ( 18.12178482187499640, 241.1218750006145228, -4.985214923628404904 ) ) ;
#2829=CARTESIAN_POINT ( 'NONE',  ( 23.87821517812500005, 242.6968750006145115, 4.985214923628404016 ) ) ;
#2832=CARTESIAN_POINT ( 'NONE',  ( 22.60769515458672885, 240.2325961894323143, 5.999999999999997335 ) ) ;
#2836=CARTESIAN_POINT ( 'NONE',  ( 26.99999999999999645, 239.8937500012290229, 3.464101615137751278 ) ) ;
#2842=CARTESIAN_POINT ( 'NONE',  ( 15.00000000000000000, 241.4687500012290684, -3.464101615137752610 ) ) ;
#2844=EDGE_CURVE ( 'NONE', #14300, #3985, #33020, .T. ) ;
#2845=ORIENTED_EDGE ( 'NONE', *, *, #16439, .F. ) ;
#2849=DIRECTION ( 'NONE',  ( -0.000000000000000000, 1.000000000000000000, -0.000000000000000000 ) ) ;
#2851=CARTESIAN_POINT ( 'NONE',  ( -27.24356964374999990, 195.3218750006145399, -15.72908226750537786 ) ) ;
#2858=CARTESIAN_POINT ( 'NONE',  ( 18.12178482187499640, 248.3218750006145115, -4.985214923628404904 ) ) ;
#2870=CARTESIAN_POINT ( 'NONE',  ( 15.24356964374999990, 249.7468750006145228, 0.000000000000000000 ) ) ;
#2871=CARTESIAN_POINT ( 'NONE',  ( -27.03767660310608889, 194.9999999999999432, 1.836876173757454378 ) ) ;
#2890=CARTESIAN_POINT ( 'NONE',  ( 7.234628195640363302, 196.3799038117967086, -26.99999999999996803 ) ) ;
#2891=CARTESIAN_POINT ( 'NONE',  ( 20.99999999999999645, 185.0294372515228645, 0.000000000000000000 ) ) ;
#2893=CARTESIAN_POINT ( 'NONE',  ( 15.24356964375000167, 246.2968750006145626, 3.323476615752272600 ) ) ;
#2895=CARTESIAN_POINT ( 'NONE',  ( 26.75643035624999655, 240.5968750006145456, 3.323476615752267271 ) ) ;
#2900=CARTESIAN_POINT ( 'NONE',  ( 15.00000000000000178, 246.9437500012290343, 3.464101615137757051 ) ) ;
#2903=ADVANCED_FACE ( 'NONE', ( #26909 ), #32593, .F. ) ;
#2909=VERTEX_POINT ( 'NONE', #15165 ) ;
#2915=CARTESIAN_POINT ( 'NONE',  ( 26.75643035624999655, 247.7218750006145171, -7.049594010296217766E-16 ) ) ;
#2920=VECTOR ( 'NONE', #26806, 1000.000000000000000 ) ;
#2935=CARTESIAN_POINT ( 'NONE',  ( 15.00000000000000000, 243.2500000000000000, 0.000000000000000000 ) ) ;
#2938=CARTESIAN_POINT ( 'NONE',  ( 26.99999999999999645, 247.1687500012290286, -3.464101615137755275 ) ) ;
#2945=CARTESIAN_POINT ( 'NONE',  ( 27.00000000000000355, 196.6250000000000284, -3.306546357697854128E-15 ) ) ;
#2946=CARTESIAN_POINT ( 'NONE',  ( 20.99999999999998579, 247.9187500012290002, 5.999999999999998224 ) ) ;
#2948=CARTESIAN_POINT ( 'NONE',  ( 18.12178482187499640, 247.9843750006145342, -4.985214923628404904 ) ) ;
#2951=CARTESIAN_POINT ( 'NONE',  ( 22.60769515458672885, 243.5674038105676686, -5.999999999999998224 ) ) ;
#2956=CARTESIAN_POINT ( 'NONE',  ( 26.99999999999999645, 241.6750000000000114, -7.347880794884117764E-16 ) ) ;
#2960=ORIENTED_EDGE ( 'NONE', *, *, #36329, .F. ) ;
#2961=CARTESIAN_POINT ( 'NONE',  ( 20.99999999999999289, 245.8374999999999773, -5.999999999999997335 ) ) ;
#2962=EDGE_CURVE ( 'NONE', #18271, #22884, #7403, .T. ) ;
#2963=CARTESIAN_POINT ( 'NONE',  ( 13.49999999999999645, 195.0125000012290570, -23.38268590217984766 ) ) ;
#2976=CARTESIAN_POINT ( 'NONE',  ( 26.08383412631443932, 195.0000000000000284, 7.525172168543629247 ) ) ;
#2977=CARTESIAN_POINT ( 'NONE',  ( 13.62178482187501416, 195.0593750006145513, 23.59362340125806767 ) ) ;
#2981=EDGE_CURVE ( 'NONE', #11333, #2407, #9779, .T. ) ;
#2983=CARTESIAN_POINT ( 'NONE',  ( 20.99999999999999645, 210.0000000000000284, -8.000000000000000000 ) ) ;
#2992=EDGE_CURVE ( 'NONE', #29774, #30702, #21427, .T. ) ;
#2998=CARTESIAN_POINT ( 'NONE',  ( 13.62178482187499640, 196.1093750006145342, -23.59362340125807123 ) ) ;
#3002=CARTESIAN_POINT ( 'NONE',  ( 23.99999999999999645, 248.5000000000000000, -5.196152422706631135 ) ) ;
#3003=CARTESIAN_POINT ( 'NONE',  ( -27.24356964375000345, 197.9656250006145797, -15.72908226750537786 ) ) ;
#3008=VERTEX_POINT ( 'NONE', #7021 ) ;
#3009=CARTESIAN_POINT ( 'NONE',  ( -13.62178482187500528, 198.8281250006145342, -23.59362340125807123 ) ) ;
#3010=CARTESIAN_POINT ( 'NONE',  ( 18.12178482187499640, 242.4718750006145171, -4.985214923628404904 ) ) ;
#3013=CARTESIAN_POINT ( 'NONE',  ( 18.12178482187500350, 248.1343750006145399, 4.985214923628407568 ) ) ;
#3018=CARTESIAN_POINT ( 'NONE',  ( 23.87821517812500005, 243.1468750006145285, 4.985214923628404016 ) ) ;
#3021=VECTOR ( 'NONE', #31303, 1000.000000000000000 ) ;
#3025=FACE_OUTER_BOUND ( 'NONE', #7069, .T. ) ;
#3029=DIRECTION ( 'NONE',  ( -0.000000000000000000, -1.000000000000000000, -0.000000000000000000 ) ) ;
#3030=CARTESIAN_POINT ( 'NONE',  ( 24.00000000000000000, 244.3562500012290286, 5.196152422706629359 ) ) ;
#3033=CARTESIAN_POINT ( 'NONE',  ( 23.87821517812500005, 242.6968750006145115, 4.985214923628404016 ) ) ;
#3041=CARTESIAN_POINT ( 'NONE',  ( 27.24356964375000700, 196.4468750006145115, 15.72908226750537075 ) ) ;
#3048=CARTESIAN_POINT ( 'NONE',  ( 26.75643035624999655, 248.2093750006145285, -3.323476615752271712 ) ) ;
#3058=VECTOR ( 'NONE', #11865, 1000.000000000000000 ) ;
#3060=CARTESIAN_POINT ( 'NONE',  ( 23.87821517812500005, 249.4468750006145115, 4.985214923628404016 ) ) ;
#3062=CARTESIAN_POINT ( 'NONE',  ( -27.10924108586912951, 194.9999999999999716, 0.1804593864224422750 ) ) ;
#3066=ORIENTED_EDGE ( 'NONE', *, *, #18177, .T. ) ;
#3067=CARTESIAN_POINT ( 'NONE',  ( -13.50000000000000533, 197.7875000012290627, -23.38268590217984411 ) ) ;
#3074=( BOUNDED_CURVE ( )  B_SPLINE_CURVE ( 2, ( #2369, #22106, #7509, #33655, #37044, #16605, #13379, #13568, #11091 ),
 .UNSPECIFIED., .F., .F. ) 
 B_SPLINE_CURVE_WITH_KNOTS ( ( 3, 2, 2, 2, 3 ),
 ( 0.5208333333333333703, 0.5277777777777777901, 0.5416666666666666297, 0.5555555555555555802, 0.5625000000000000000 ),
 .UNSPECIFIED. ) 
 CURVE ( )  GEOMETRIC_REPRESENTATION_ITEM ( )  RATIONAL_B_SPLINE_CURVE ( ( 0.9330127018922192983, 0.9330127018922198534, 1.000000000000000000, 0.8660254037844387076, 1.000000000000000000, 0.8660254037844387076, 1.000000000000000000, 0.9330127018922194093, 0.9330127018922194093 ) ) 
 REPRESENTATION_ITEM ( '' )  );
#3075=VERTEX_POINT ( 'NONE', #29563 ) ;
#3080=CARTESIAN_POINT ( 'NONE',  ( 1.120210788295102201E-13, 196.4000000012290741, -27.00000000000000711 ) ) ;
#3081=CYLINDRICAL_SURFACE ( 'NONE', #6138, 5.999999999999999112 ) ;
#3083=CARTESIAN_POINT ( 'NONE',  ( 15.24356964374999990, 245.8093750006145228, 0.000000000000000000 ) ) ;
#3090=CARTESIAN_POINT ( 'NONE',  ( 24.00000000000000000, 245.7062500012290513, 5.196152422706629359 ) ) ;
#3093=CARTESIAN_POINT ( 'NONE',  ( 5.438367727407757144E-14, 198.2000000012290002, -27.00000000000000000 ) ) ;
#3102=CARTESIAN_POINT ( 'NONE',  ( 18.12178482187500350, 247.1218750006145228, 4.985214923628407568 ) ) ;
#3110=VECTOR ( 'NONE', #6108, 1000.000000000000000 ) ;
#3115=DIRECTION ( 'NONE',  ( -1.000000000000000000, 0.000000000000000000, 0.000000000000000000 ) ) ;
#3118=ORIENTED_EDGE ( 'NONE', *, *, #23504, .F. ) ;
#3130=CARTESIAN_POINT ( 'NONE',  ( 1.120210788295102201E-13, 195.8375000000000057, -27.00000000000000711 ) ) ;
#3132=CARTESIAN_POINT ( 'NONE',  ( 26.99999999999999645, 195.3125000000000284, -15.58845726811990495 ) ) ;
#3133=CARTESIAN_POINT ( 'NONE',  ( 18.00000000000000355, 240.1750000000000114, 5.196152422706632912 ) ) ;
#3135=CARTESIAN_POINT ( 'NONE',  ( 23.87821517812500005, 246.4093750006145171, 4.985214923628404016 ) ) ;
#3143=CARTESIAN_POINT ( 'NONE',  ( 18.00000000000000000, 241.8250000000000171, -5.196152422706630247 ) ) ;
#3163=CARTESIAN_POINT ( 'NONE',  ( 5.778771075727756162E-15, 195.4718750006145456, 31.45816453501075927 ) ) ;
#3167=FACE_OUTER_BOUND ( 'NONE', #12620, .T. ) ;
#3168=DIRECTION ( 'NONE',  ( 0.000000000000000000, 0.000000000000000000, 1.000000000000000000 ) ) ;
#3172=( BOUNDED_CURVE ( )  B_SPLINE_CURVE ( 2, ( #15702, #26489, #1276, #3372, #29711, #20828, #17981, #12847, #521 ),
 .UNSPECIFIED., .F., .F. ) 
 B_SPLINE_CURVE_WITH_KNOTS ( ( 3, 2, 2, 2, 3 ),
 ( 0.7291666666666667407, 0.7361111111111111605, 0.7500000000000000000, 0.7638888888888888395, 0.7708333333333333703 ),
 .UNSPECIFIED. ) 
 CURVE ( )  GEOMETRIC_REPRESENTATION_ITEM ( )  RATIONAL_B_SPLINE_CURVE ( ( 0.9330127018922192983, 0.9330127018922198534, 1.000000000000000000, 0.8660254037844387076, 1.000000000000000000, 0.8660254037844387076, 1.000000000000000000, 0.9330127018922187432, 0.9330127018922192983 ) ) 
 REPRESENTATION_ITEM ( '' )  );
#3182=CARTESIAN_POINT ( 'NONE',  ( 7.234628195640309123, 196.2674038105676573, -27.00000000000000711 ) ) ;
#3185=CARTESIAN_POINT ( 'NONE',  ( -27.00000000000000355, 198.2000000000000171, 0.000000000000000000 ) ) ;
#3186=CARTESIAN_POINT ( 'NONE',  ( 21.00000000000000000, 247.8625000000000114, 6.928203230275506996 ) ) ;
#3187=CARTESIAN_POINT ( 'NONE',  ( -13.62178482187498396, 198.0781250006145342, 23.59362340125808188 ) ) ;
#3190=EDGE_LOOP ( 'NONE', ( #2250, #8751, #30136, #10651 ) ) ;
#3192=CARTESIAN_POINT ( 'NONE',  ( -27.24356964374999990, 198.8656250006145569, -15.72908226750537786 ) ) ;
#3193=CARTESIAN_POINT ( 'NONE',  ( 21.00000000000000000, 241.9843750006145058, -6.646953231504538984 ) ) ;
#3197=CARTESIAN_POINT ( 'NONE',  ( 23.87821517812500005, 248.2093750006145285, 4.985214923628404016 ) ) ;
#3204=CARTESIAN_POINT ( 'NONE',  ( 18.12178482187500350, 243.0718750006145399, 4.985214923628407568 ) ) ;
#3208=CIRCLE ( 'NONE', #26199, 2.649999999999990585 ) ;
#3213=DIRECTION ( 'NONE',  ( -0.000000000000000000, -1.000000000000000000, -0.000000000000000000 ) ) ;
#3222=CARTESIAN_POINT ( 'NONE',  ( 26.75643035624999655, 241.8343750006145001, 3.323476615752267715 ) ) ;
#3227=CARTESIAN_POINT ( 'NONE',  ( 22.60769515458672885, 241.7674038105676573, -5.999999999999998224 ) ) ;
#3228=FACE_OUTER_BOUND ( 'NONE', #7592, .T. ) ;
#3229=CARTESIAN_POINT ( 'NONE',  ( 20.99999999999999645, 202.0000000000000000, 5.999999999999999112 ) ) ;
#3231=CARTESIAN_POINT ( 'NONE',  ( -13.50000000000000533, 196.8875000012290286, -23.38268590217984411 ) ) ;
#3236=CARTESIAN_POINT ( 'NONE',  ( 18.91622474583366653, 239.6197971919061160, -5.725135026351895640 ) ) ;
#3241=VECTOR ( 'NONE', #12985, 1000.000000000000000 ) ;
#3242=FACE_OUTER_BOUND ( 'NONE', #33221, .T. ) ;
#3248=CARTESIAN_POINT ( 'NONE',  ( 23.87821517812500005, 248.5468750006145058, 4.985214923628404016 ) ) ;
#3250=CARTESIAN_POINT ( 'NONE',  ( -26.01826704599283246, 194.9999999999999716, -7.493920110828625525 ) ) ;
#3254=ORIENTED_EDGE ( 'NONE', *, *, #14770, .T. ) ;
#3255=CARTESIAN_POINT ( 'NONE',  ( 22.60769515458673240, 247.9388461906613372, 6.000000000000000000 ) ) ;
#3266=CARTESIAN_POINT ( 'NONE',  ( -3.253724281355068545E-15, 195.9500000012290002, -27.00000000000000000 ) ) ;
#3272=CARTESIAN_POINT ( 'NONE',  ( 18.12178482187500350, 245.4343750006145228, 4.985214923628407568 ) ) ;
#3277=CARTESIAN_POINT ( 'NONE',  ( 15.00000000000000000, 245.5187500012290513, -3.464101615137752166 ) ) ;
#3280=CARTESIAN_POINT ( 'NONE',  ( 26.99999999999999645, 198.1250000012290400, -15.58845726811990495 ) ) ;
#3281=( BOUNDED_CURVE ( )  B_SPLINE_CURVE ( 2, ( #18782, #2434, #5458, #16859, #34091, #20072, #28396, #25559, #34281 ),
 .UNSPECIFIED., .F., .F. ) 
 B_SPLINE_CURVE_WITH_KNOTS ( ( 3, 2, 2, 2, 3 ),
 ( 0.09782608695652174335, 0.1014492753623188470, 0.1086956521739130405, 0.1159420289855072478, 0.1195652173913043653 ),
 .UNSPECIFIED. ) 
 CURVE ( )  GEOMETRIC_REPRESENTATION_ITEM ( )  RATIONAL_B_SPLINE_CURVE ( ( 0.9330127018922194093, 0.9330127018922194093, 1.000000000000000000, 0.8660254037844387076, 1.000000000000000000, 0.8660254037844387076, 1.000000000000000000, 0.9330127018922190762, 0.9330127018922194093 ) ) 
 REPRESENTATION_ITEM ( '' )  );
#3285=ORIENTED_EDGE ( 'NONE', *, *, #31093, .F. ) ;
#3290=CARTESIAN_POINT ( 'NONE',  ( 18.12178482187500350, 246.2218750006145171, 4.985214923628407568 ) ) ;
#3293=CARTESIAN_POINT ( 'NONE',  ( 17.52409618573022954, 213.4759038142404677, -5.188047882447234471 ) ) ;
#3299=( BOUNDED_CURVE ( )  B_SPLINE_CURVE ( 2, ( #8475, #19868, #31773, #37452, #17573, #8846, #31961, #22887, #5993 ),
 .UNSPECIFIED., .F., .T. ) 
 B_SPLINE_CURVE_WITH_KNOTS ( ( 3, 2, 2, 2, 3 ),
 ( 0.5625000000000000000, 0.5694444444444444198, 0.5833333333333333703, 0.5972222222222222099, 0.6041666666666667407 ),
 .UNSPECIFIED. ) 
 CURVE ( )  GEOMETRIC_REPRESENTATION_ITEM ( )  RATIONAL_B_SPLINE_CURVE ( ( 0.9330127018922194093, 0.9330127018922194093, 1.000000000000000000, 0.8660254037844387076, 1.000000000000000000, 0.8660254037844387076, 1.000000000000000000, 0.9330127018922187432, 0.9330127018922192983 ) ) 
 REPRESENTATION_ITEM ( '' )  );
#3304=ORIENTED_EDGE ( 'NONE', *, *, #22225, .T. ) ;
#3305=CARTESIAN_POINT ( 'NONE',  ( 21.00000000000000000, 240.6624999999999943, 5.999999999999998224 ) ) ;
#3309=LINE ( 'NONE', #27184, #33714 ) ;
#3318=CARTESIAN_POINT ( 'NONE',  ( -27.24356964375000345, 199.8593750006145342, 0.000000000000000000 ) ) ;
#3321=CARTESIAN_POINT ( 'NONE',  ( 18.12178482187500350, 247.6843750006145228, 4.985214923628407568 ) ) ;
#3328=CARTESIAN_POINT ( 'NONE',  ( 23.99999999999999645, 242.1999999999999886, -5.196152422706631135 ) ) ;
#3334=CARTESIAN_POINT ( 'NONE',  ( -27.00000000000000355, 194.6888594429640591, -9.827195528215911580 ) ) ;
#3340=EDGE_CURVE ( 'NONE', #18271, #21289, #36364, .T. ) ;
#3344=DIRECTION ( 'NONE',  ( 1.000000000000000000, 0.000000000000000000, 0.000000000000000000 ) ) ;
#3350=AXIS2_PLACEMENT_3D ( 'NONE', #33502, #24964, #10381 ) ;
#3351=CARTESIAN_POINT ( 'NONE',  ( 20.71295208575482505, 194.9999999999999716, -17.38774714927576071 ) ) ;
#3352=CARTESIAN_POINT ( 'NONE',  ( 27.24356964375000345, 195.1343750006145399, -3.336375036156643733E-15 ) ) ;
#3358=CARTESIAN_POINT ( 'NONE',  ( 15.00000000000000000, 247.2999999999999829, 0.000000000000000000 ) ) ;
#3365=CARTESIAN_POINT ( 'NONE',  ( 26.99999999999999645, 244.8249999999999886, -7.347880794884117764E-16 ) ) ;
#3369=CARTESIAN_POINT ( 'NONE',  ( 26.99999999999999645, 244.8812500012290343, -7.347880794884117764E-16 ) ) ;
#3372=CARTESIAN_POINT ( 'NONE',  ( -26.99999999999999645, 195.6500000012290457, 15.58845726811991561 ) ) ;
#3377=CARTESIAN_POINT ( 'NONE',  ( 23.99999999999999645, 247.5999999999999943, -5.196152422706631135 ) ) ;
#3378=CARTESIAN_POINT ( 'NONE',  ( 13.62178482187501416, 195.0031250006145456, 23.59362340125806767 ) ) ;
#3383=VERTEX_POINT ( 'NONE', #33905 ) ;
#3384=CARTESIAN_POINT ( 'NONE',  ( -27.24356964375001056, 194.8294844423495533, -9.915847621322177119 ) ) ;
#3389=CARTESIAN_POINT ( 'NONE',  ( 15.24356964375000167, 247.1968750006145115, 3.323476615752272600 ) ) ;
#3395=CARTESIAN_POINT ( 'NONE',  ( 15.24356964374999990, 242.0593750006145228, -3.323476615752268604 ) ) ;
#3400=AXIS2_PLACEMENT_3D ( 'NONE', #30928, #4582, #28263 ) ;
#3406=CARTESIAN_POINT ( 'NONE',  ( 20.99999999999999289, 244.0374999999999943, -5.999999999999997335 ) ) ;
#3408=CARTESIAN_POINT ( 'NONE',  ( 1.069080835302379631E-14, 198.8750000012290400, 27.00000000000000000 ) ) ;
#3411=CARTESIAN_POINT ( 'NONE',  ( 21.00000000000000000, 241.3093750006145228, 6.646953231504538984 ) ) ;
#3417=DIRECTION ( 'NONE',  ( 1.000000000000000000, 0.000000000000000000, 0.000000000000000000 ) ) ;
#3419=CARTESIAN_POINT ( 'NONE',  ( 20.99999999999997868, 210.0000000000000000, 5.999999999999999112 ) ) ;
#3424=CARTESIAN_POINT ( 'NONE',  ( 18.00000000000000355, 240.2312500012290570, 5.196152422706632912 ) ) ;
#3431=ORIENTED_EDGE ( 'NONE', *, *, #30942, .T. ) ;
#3435=DIRECTION ( 'NONE',  ( -0.000000000000000000, -1.000000000000000000, -0.000000000000000000 ) ) ;
#3437=CARTESIAN_POINT ( 'NONE',  ( -26.52865046747503186, 195.0000000000000568, 5.702742731586317504 ) ) ;
#3442=CARTESIAN_POINT ( 'NONE',  ( -27.89350125246770418, 208.9432337700812354, 7.934313662097031816 ) ) ;
#3453=( BOUNDED_CURVE ( )  B_SPLINE_CURVE ( 2, ( #12781, #30602, #22258, #36451, #21517, #36082, #10679, #7847, #4619 ),
 .UNSPECIFIED., .F., .F. ) 
 B_SPLINE_CURVE_WITH_KNOTS ( ( 3, 2, 2, 2, 3 ),
 ( 0.5108695652173913526, 0.5144927536231883591, 0.5217391304347825942, 0.5289855072463768293, 0.5326086956521739468 ),
 .UNSPECIFIED. ) 
 CURVE ( )  GEOMETRIC_REPRESENTATION_ITEM ( )  RATIONAL_B_SPLINE_CURVE ( ( 0.9330127018922192983, 0.9330127018922202975, 1.000000000000000000, 0.8660254037844387076, 1.000000000000000000, 0.8660254037844387076, 1.000000000000000000, 0.9330127018922194093, 0.9330127018922194093 ) ) 
 REPRESENTATION_ITEM ( '' )  );
#3457=CARTESIAN_POINT ( 'NONE',  ( -3.253724281355068545E-15, 195.9500000012290002, -27.00000000000000000 ) ) ;
#3458=DIRECTION ( 'NONE',  ( -0.000000000000000000, -1.000000000000000000, -0.000000000000000000 ) ) ;
#3461=CARTESIAN_POINT ( 'NONE',  ( 18.12178482187500350, 241.8343750006145285, 4.985214923628407568 ) ) ;
#3464=ORIENTED_EDGE ( 'NONE', *, *, #11515, .T. ) ;
#3468=CARTESIAN_POINT ( 'NONE',  ( 26.99999999999999645, 246.6437500012290513, 3.464101615137751278 ) ) ;
#3479=CARTESIAN_POINT ( 'NONE',  ( 18.12178482187500350, 245.7718750006145001, 4.985214923628407568 ) ) ;
#3502=( BOUNDED_CURVE ( )  B_SPLINE_CURVE ( 2, ( #28574, #14557, #25554, #31432, #5640, #7943, #28762, #11523, #28951 ),
 .UNSPECIFIED., .F., .F. ) 
 B_SPLINE_CURVE_WITH_KNOTS ( ( 3, 2, 2, 2, 3 ),
 ( 0.4375000000000000000, 0.4444444444444444198, 0.4583333333333333148, 0.4722222222222222099, 0.4791666666666666852 ),
 .UNSPECIFIED. ) 
 CURVE ( )  GEOMETRIC_REPRESENTATION_ITEM ( )  RATIONAL_B_SPLINE_CURVE ( ( 0.9330127018922194093, 0.9330127018922194093, 1.000000000000000000, 0.8660254037844387076, 1.000000000000000000, 0.8660254037844387076, 1.000000000000000000, 0.9330127018922190762, 0.9330127018922194093 ) ) 
 REPRESENTATION_ITEM ( '' )  );
#3505=CARTESIAN_POINT ( 'NONE',  ( 19.39230484541326049, 249.0075961894323484, -5.999999999999997335 ) ) ;
#3509=CARTESIAN_POINT ( 'NONE',  ( 15.24356964374999990, 246.2218750006145456, -3.323476615752268604 ) ) ;
#3517=CARTESIAN_POINT ( 'NONE',  ( 21.00000000000000000, 242.0125000000000171, 6.928203230275506996 ) ) ;
#3518=CARTESIAN_POINT ( 'NONE',  ( -5.732297079746171420, 222.9518338469886203, 2.500000000000000000 ) ) ;
#3522=VECTOR ( 'NONE', #2849, 1000.000000000000000 ) ;
#3525=CARTESIAN_POINT ( 'NONE',  ( 18.00000000000000355, 243.7750000000000057, 5.196152422706632912 ) ) ;
#3532=( BOUNDED_CURVE ( )  B_SPLINE_CURVE ( 2, ( #34643, #20262, #20450, #31992, #17788, #6021, #334 ),
 .UNSPECIFIED., .F., .F. ) 
 B_SPLINE_CURVE_WITH_KNOTS ( ( 3, 2, 2, 3 ),
 ( 0.8958333333333333703, 0.9027777777777777901, 0.9166666666666666297, 0.9257860730087129619 ),
 .UNSPECIFIED. ) 
 CURVE ( )  GEOMETRIC_REPRESENTATION_ITEM ( )  RATIONAL_B_SPLINE_CURVE ( ( 0.9330127018922192983, 0.9330127018922198534, 1.000000000000000000, 0.8660254037844387076, 1.000000000000000000, 0.9120326476671077875, 0.9395835397633095498 ) ) 
 REPRESENTATION_ITEM ( '' )  );
#3544=CARTESIAN_POINT ( 'NONE',  ( 27.24356964374999635, 199.1656250006145399, -15.72908226750539029 ) ) ;
#3547=ORIENTED_EDGE ( 'NONE', *, *, #27779, .F. ) ;
#3549=CARTESIAN_POINT ( 'NONE',  ( 26.99999999999999645, 245.2937500012290570, 3.464101615137751278 ) ) ;
#3559=EDGE_CURVE ( 'NONE', #17126, #2909, #8345, .T. ) ;
#3562=DIRECTION ( 'NONE',  ( -0.000000000000000000, 1.000000000000000000, -0.000000000000000000 ) ) ;
#3569=CARTESIAN_POINT ( 'NONE',  ( -4.694659320240884604E-14, 197.0750000012290570, 27.00000000000000000 ) ) ;
#3570=CARTESIAN_POINT ( 'NONE',  ( 18.00000000000000000, 249.0250000000000057, -5.196152422706630247 ) ) ;
#3571=CARTESIAN_POINT ( 'NONE',  ( -27.24356964375000345, 196.1656250006145399, -15.72908226750537786 ) ) ;
#3576=CARTESIAN_POINT ( 'NONE',  ( 27.24356964374999635, 195.5656250006145171, -15.72908226750539029 ) ) ;
#3577=CARTESIAN_POINT ( 'NONE',  ( 23.87821517812499650, 240.5968750006145171, -4.985214923628404904 ) ) ;
#3580=CARTESIAN_POINT ( 'NONE',  ( 18.12178482187499640, 247.9843750006145342, -4.985214923628404904 ) ) ;
#3582=CARTESIAN_POINT ( 'NONE',  ( 0.000000000000000000, 210.0000000000000284, 0.000000000000000000 ) ) ;
#3585=ADVANCED_FACE ( 'NONE', ( #34639 ), #144, .F. ) ;
#3587=CARTESIAN_POINT ( 'NONE',  ( 15.24356964374999990, 242.0968750006145171, 0.000000000000000000 ) ) ;
#3603=CARTESIAN_POINT ( 'NONE',  ( 18.12178482187499640, 241.1218750006145228, -4.985214923628404904 ) ) ;
#3608=CARTESIAN_POINT ( 'NONE',  ( -13.62178482187498396, 199.4843750006145626, 23.59362340125808188 ) ) ;
#3615=ORIENTED_EDGE ( 'NONE', *, *, #16784, .F. ) ;
#3617=CARTESIAN_POINT ( 'NONE',  ( 23.87821517812500005, 248.0968750006144887, 4.985214923628404016 ) ) ;
#3639=CARTESIAN_POINT ( 'NONE',  ( 18.00000000000000000, 249.0812500012290513, -5.196152422706630247 ) ) ;
#3647=AXIS2_PLACEMENT_3D ( 'NONE', #15808, #1388, #36069 ) ;
#3651=CARTESIAN_POINT ( 'NONE',  ( 1.255007937094097924E-14, 199.1000000012290627, -27.00000000000000355 ) ) ;
#3655=CARTESIAN_POINT ( 'NONE',  ( 15.00000000000000178, 242.8937500012290513, 3.464101615137757051 ) ) ;
#3662=ORIENTED_EDGE ( 'NONE', *, *, #5683, .T. ) ;
#3667=CARTESIAN_POINT ( 'NONE',  ( 15.24356964374999990, 246.1093750006145342, -3.323476615752268604 ) ) ;
#3683=CARTESIAN_POINT ( 'NONE',  ( 20.99999999999999645, 185.0294372515228645, -5.999999999999999112 ) ) ;
#3687=DIRECTION ( 'NONE',  ( -0.000000000000000000, 1.000000000000000000, -0.000000000000000000 ) ) ;
#3693=CARTESIAN_POINT ( 'NONE',  ( 27.00000000000001421, 195.6875000000000000, 15.58845726811988897 ) ) ;
#3695=CARTESIAN_POINT ( 'NONE',  ( 15.24356964374999990, 249.4093750006145171, 0.000000000000000000 ) ) ;
#3697=CARTESIAN_POINT ( 'NONE',  ( 15.24356964375000167, 245.3968750006145285, 3.323476615752272600 ) ) ;
#3700=DIRECTION ( 'NONE',  ( -1.000000000000000000, -4.130293990420971855E-17, 0.000000000000000000 ) ) ;
#3701=DIRECTION ( 'NONE',  ( -0.000000000000000000, 1.000000000000000000, -0.000000000000000000 ) ) ;
#3708=DIRECTION ( 'NONE',  ( -1.000000000000000000, -6.123233995736766036E-17, -0.000000000000000000 ) ) ;
#3711=CARTESIAN_POINT ( 'NONE',  ( 20.99999999999995381, 242.9124999999999943, 5.999999999999998224 ) ) ;
#3724=CARTESIAN_POINT ( 'NONE',  ( -13.62178482187498396, 197.6281250006145171, 23.59362340125808188 ) ) ;
#3741=CARTESIAN_POINT ( 'NONE',  ( 20.99999999999999645, 185.0294372515228645, 5.999999999999999112 ) ) ;
#3743=CARTESIAN_POINT ( 'NONE',  ( 20.99999999999997513, 244.9937500012290457, -5.999999999999999112 ) ) ;
#3745=CARTESIAN_POINT ( 'NONE',  ( -7.234628195640302017, 198.4049038117967143, 27.00000000000000711 ) ) ;
#3749=CARTESIAN_POINT ( 'NONE',  ( 21.00000000000000000, 247.6374999999999886, -6.928203230275506996 ) ) ;
#3750=CARTESIAN_POINT ( 'NONE',  ( -27.24356964375000345, 195.7531250006145456, 0.000000000000000000 ) ) ;
#3754=EDGE_LOOP ( 'NONE', ( #7663, #26831, #26253, #20177 ) ) ;
#3756=CARTESIAN_POINT ( 'NONE',  ( -27.00000000000000355, 199.6250000012290684, -15.58845726811989429 ) ) ;
#3757=CARTESIAN_POINT ( 'NONE',  ( 15.24356964375000167, 240.3343750006145001, 3.323476615752272600 ) ) ;
#3760=CARTESIAN_POINT ( 'NONE',  ( 15.24356964374999990, 247.6093750006145342, 0.000000000000000000 ) ) ;
#3763=DIRECTION ( 'NONE',  ( 0.000000000000000000, 0.000000000000000000, -1.000000000000000000 ) ) ;
#3767=CARTESIAN_POINT ( 'NONE',  ( 18.12178482187499640, 240.2218750006145171, -4.985214923628404904 ) ) ;
#3777=DIRECTION ( 'NONE',  ( -0.000000000000000000, 1.000000000000000000, -0.000000000000000000 ) ) ;
#3783=CARTESIAN_POINT ( 'NONE',  ( 26.75643035624999655, 242.2843750006145171, 3.323476615752267715 ) ) ;
#3787=CARTESIAN_POINT ( 'NONE',  ( 19.96869161633227208, 239.9653672772770392, -5.848880403311082610 ) ) ;
#3788=DIRECTION ( 'NONE',  ( -0.000000000000000000, 1.000000000000000000, -0.000000000000000000 ) ) ;
#3789=CARTESIAN_POINT ( 'NONE',  ( 20.99999999999999645, 185.0294372515228645, 5.999999999999999112 ) ) ;
#3790=ADVANCED_FACE ( 'NONE', ( #17412 ), #34826, .F. ) ;
#3795=ORIENTED_EDGE ( 'NONE', *, *, #10580, .F. ) ;
#3796=CARTESIAN_POINT ( 'NONE',  ( 23.87821517812499650, 246.4468750006145115, -4.985214923628404904 ) ) ;
#3801=EDGE_CURVE ( 'NONE', #23017, #36288, #12273, .T. ) ;
#3810=CARTESIAN_POINT ( 'NONE',  ( 26.75643035624999655, 245.9593750006145285, -3.323476615752271268 ) ) ;
#3818=CARTESIAN_POINT ( 'NONE',  ( 26.99999999999999645, 241.7312500012290570, -7.347880794884117764E-16 ) ) ;
#3839=CARTESIAN_POINT ( 'NONE',  ( 23.87821517812499650, 240.2593750006145399, -4.985214923628404904 ) ) ;
#3840=ORIENTED_EDGE ( 'NONE', *, *, #24664, .F. ) ;
#3841=CARTESIAN_POINT ( 'NONE',  ( 18.00000000000000000, 244.1312500012290343, -5.196152422706630247 ) ) ;
#3845=CARTESIAN_POINT ( 'NONE',  ( -29.00000000000002487, 210.0000000000000000, 0.000000000000000000 ) ) ;
#3852=CARTESIAN_POINT ( 'NONE',  ( 26.75643035624999655, 245.4343750006145228, 3.323476615752267715 ) ) ;
#3858=( LENGTH_UNIT ( ) NAMED_UNIT ( * ) SI_UNIT ( .MILLI., .METRE. ) );
#3877=CYLINDRICAL_SURFACE ( 'NONE', #6782, 5.999999999999999112 ) ;
#3881=CARTESIAN_POINT ( 'NONE',  ( 26.75643035624999655, 249.6343750006145399, -7.049594010296217766E-16 ) ) ;
#3883=CARTESIAN_POINT ( 'NONE',  ( 23.87821517812499650, 246.5593750006145228, -4.985214923628404904 ) ) ;
#3884=ORIENTED_EDGE ( 'NONE', *, *, #7534, .T. ) ;
#3893=DIRECTION ( 'NONE',  ( -0.000000000000000000, -1.000000000000000000, -0.000000000000000000 ) ) ;
#3896=VERTEX_POINT ( 'NONE', #700 ) ;
#3898=CARTESIAN_POINT ( 'NONE',  ( 1.120210788295102201E-13, 195.8375000000000057, -27.00000000000000711 ) ) ;
#3904=CARTESIAN_POINT ( 'NONE',  ( 0.000000000000000000, 210.0000000000000284, 0.000000000000000000 ) ) ;
#3913=CARTESIAN_POINT ( 'NONE',  ( 20.99999999999999289, 248.8187500012290911, 5.999999999999999112 ) ) ;
#3914=CARTESIAN_POINT ( 'NONE',  ( 27.24356964374999635, 198.2656250006145058, -15.72908226750539029 ) ) ;
#3919=DIRECTION ( 'NONE',  ( 1.000000000000000000, 0.000000000000000000, 0.000000000000000000 ) ) ;
#3936=CARTESIAN_POINT ( 'NONE',  ( -7.234628195640289583, 198.2200961906613372, -27.00000000000001421 ) ) ;
#3939=CARTESIAN_POINT ( 'NONE',  ( 18.00000000000000000, 244.9749999999999943, -5.196152422706630247 ) ) ;
#3940=CARTESIAN_POINT ( 'NONE',  ( -13.62178482187498396, 195.3781250006145171, 23.59362340125808188 ) ) ;
#3944=ORIENTED_EDGE ( 'NONE', *, *, #27886, .F. ) ;
#3946=CARTESIAN_POINT ( 'NONE',  ( 13.49999999999999645, 199.5125000012290286, -23.38268590217984766 ) ) ;
#3947=CARTESIAN_POINT ( 'NONE',  ( 26.75643035624999655, 240.5593750006145513, -3.323476615752271712 ) ) ;
#3951=CARTESIAN_POINT ( 'NONE',  ( 21.00000000000000000, 245.4718750006145456, 6.646953231504538984 ) ) ;
#3963=FACE_OUTER_BOUND ( 'NONE', #10758, .T. ) ;
#3968=CARTESIAN_POINT ( 'NONE',  ( 1.069080835302379631E-14, 198.3124999999999716, 27.00000000000000000 ) ) ;
#3971=( BOUNDED_SURFACE ( )  B_SPLINE_SURFACE ( 1, 2, ( 
 ( #4071, #21527, #18305, #29845, #30037, #23988, #3881, #15455, #21340, #27007, #29659, #15643, #3695, #18688, #27193, #1218, #24360, #35903, #9946, #33073, #7117, #4255, #15831, #27379, #1409, #34185, #33997, #30790, #16760, #37018, #13541, #22266, #16207, #24908, #10502, #13167, #27938, #4627, #8230, #8041, #11064, #27755, #33819, #4813, #7857, #25094, #22638, #28307, #36651, #10877, #2346, #19429, #36273, #31340, #13735, #21891, #22450, #2154, #36460, #16393, #10688, #19805, #19059, #1599, #30979, #4997, #28124, #19617, #5367, #25283, #10318, #30611, #33440, #36834, #19250, #1785, #16579, #16946, #13918, #31163, #24722, #7481, #33632, #13353, #5186, #22080, #25468, #7671, #1968, #8781, #20162, #25835, #17504, #31895, #28859, #2893, #14652, #17693, #11435, #17317, #11991, #6111, #20539, #5924, #26393, #23190, #14466, #2708, #3083, #11615, #23002, #28488, #23563, #5549, #17134, #9156, #26020, #34551, #3272, #28670, #37203, #14098, #37383, #426, #20353, #14284, #20723, #8591, #31710, #34738, #29039, #5737, #32267, #29232, #35108, #32082, #14845, #48, #26203, #31523, #11804, #240, #6310, #2532, #23374, #34923, #25650, #8967, #11250, #22820, #34369, #8412, #19981, #33544, #16306, #30331, #1511, #32980, #4174, #27295, #29427, #7218, #20918, #13457, #13270, #27853, #7034, #13085, #10046, #24639, #4355, #1886, #7586, #15935, #27671, #19162, #36190, #15031, #10604, #30525, #609, #1697, #18970, #15744, #21623, #27484, #25007, #35291, #17882, #10234, #21809, #7398, #24823, #36563, #4545, #26580, #9347, #12178, #16121, #36008, #18601, #33362, #22184, #30711, #36376, #33732, #23752, #12894, #30144, #10422, #1326, #21997, #4731, #24459, #3461, #33174, #18790, #34291, #11168, #8150, #19722, #31445, #34472, #28229, #34100, #28775, #22927, #37306, #22741, #5654, #2444, #31262, #19532, #19904, #28405, #2258, #7773, #2815, #22368, #33916, #25943, #5288, #13837, #20082, #7958, #16494, #30890, #16682, #17236, #37120, #31080, #37486, #5103, #25384, #14018, #25568, #36934, #11537, #8515, #14385, #11356, #31626, #10980, #8334, #10795, #28588, #16868, #23108, #19351 ),
 ( #36754, #4913, #22551, #5468, #17050, #28042, #2075, #2626, #14202, #13648, #25753, #25201, #26875, #9260, #17424, #6412, #35210, #20458, #343, #20642, #18175, #14572, #34652, #29339, #32189, #23666, #3570, #15324, #20832, #5846, #26124, #28963, #32374, #14761, #156, #6223, #32559, #35397, #17796, #6601, #3002, #29145, #34840, #15131, #17615, #17987, #29530, #31999, #14946, #26306, #6029, #26683, #525, #35028, #9072, #713, #23858, #3186, #23475, #29716, #12285, #9445, #12092, #3749, #3377, #26493, #8880, #21024, #906, #11908, #8696, #12476, #11721, #23295, #20270, #31809, #18559, #36334, #24231, #32750, #9634, #32937, #21955, #15894, #1094, #16268, #12663, #4133, #30290, #4315, #30101, #4686, #13234, #33501, #27630, #10380, #35775, #24600, #27070, #7359, #21585, #1845, #27817, #35966, #10004, #21211, #27439, #7546, #18361, #15705, #24044, #15514, #19118, #18931, #27256, #1660, #30668, #33132, #7175, #9819, #21396, #6991, #35589, #12850, #1279, #6787, #30484, #29910, #24418, #18748, #1471, #13045, #24783, #36150, #3939, #10193, #21769, #33319, #4504, #16081, #36713, #25712, #31405, #10565, #37265, #5424, #2402, #2215, #10940, #25344, #22142, #22880, #13797, #4875, #8468, #20038, #19680, #5248, #22703, #7919, #33877, #8106, #25158, #19493, #31039, #36893, #5061, #28732, #22513, #24963, #19862, #31219, #13977, #16825, #28367, #33688, #31584, #34060, #17005, #17192, #2588, #34247, #19312, #25527, #13415, #37080, #11126, #36521, #7729, #14158, #30850, #11312, #16454, #28184, #10752, #27998, #13609, #34431, #8290, #28546, #2031, #5608, #22325, #16643, #8652, #23249, #31767, #12235, #3328, #14899, #6553, #20975, #34795, #3517, #20595, #29100, #17565, #23063, #3143, #12047, #26259, #20782, #2956, #295, #20221, #17378, #26447, #26081, #11860, #480, #35162, #32136, #5798, #9211, #11494, #20411, #35347, #663, #28921, #18126, #17748, #9400, #14711, #2770, #15084, #8839, #32508, #14343, #25897, #34609, #31953, #37445, #32325, #23617, #29480, #5985, #14525, #6365, #17936, #110, #26634, #11674, #23429, #34981, #23806, #9023, #6176, #29289, #27579 ) ),
 .UNSPECIFIED., .F., .F., .F. ) 
 B_SPLINE_SURFACE_WITH_KNOTS ( ( 2, 2 ),
 ( 3, 2, 2, 2, 2, 2, 2, 2, 2, 2, 2, 2, 2, 2, 2, 2, 2, 2, 2, 2, 2, 2, 2, 2, 2, 2, 2, 2, 2, 2, 2, 2, 2, 2, 2, 2, 2, 2, 2, 2, 2, 2, 2, 2, 2, 2, 2, 2, 2, 2, 2, 2, 2, 2, 2, 2, 2, 2, 2, 2, 2, 2, 2, 2, 2, 2, 2, 2, 2, 2, 2, 2, 2, 2, 2, 2, 2, 2, 2, 2, 2, 2, 2, 2, 2, 2, 2, 2, 2, 2, 2, 2, 2, 2, 2, 2, 2, 2, 2, 2, 2, 2, 2, 2, 2, 2, 2, 2, 2, 2, 2, 2, 2, 2, 2, 2, 2, 2, 2, 2, 2, 2, 2, 2, 2, 2, 2, 2, 2, 2, 2, 2, 2, 2, 3 ),
 ( 0.000000000000000000, 1.000000000000000000 ),
 ( 0.000000000000000000, 0.007246376811594202987, 0.01449275362318840597, 0.02173913043478260809, 0.02898550724637681195, 0.03623188405797101580, 0.04347826086956521618, 0.05072463768115942351, 0.05797101449275362389, 0.06521739130434782428, 0.07246376811594203160, 0.07971014492753622505, 0.08695652173913043237, 0.09420289855072463969, 0.1014492753623188470, 0.1086956521739130405, 0.1159420289855072478, 0.1231884057971014551, 0.1304347826086956486, 0.1376811594202898559, 0.1449275362318840632, 0.1521739130434782705, 0.1594202898550724501, 0.1666666666666666574, 0.1739130434782608647, 0.1811594202898550721, 0.1884057971014492794, 0.1956521739130434867, 0.2028985507246376940, 0.2101449275362318736, 0.2173913043478260809, 0.2246376811594202882, 0.2318840579710144956, 0.2391304347826087029, 0.2463768115942029102, 0.2536231884057971175, 0.2608695652173912971, 0.2681159420289855322, 0.2753623188405797118, 0.2826086956521738913, 0.2898550724637681264, 0.2971014492753623060, 0.3043478260869565410, 0.3115942028985507206, 0.3188405797101449002, 0.3260869565217391353, 0.3333333333333333148, 0.3405797101449275499, 0.3478260869565217295, 0.3550724637681159646, 0.3623188405797101441, 0.3695652173913043237, 0.3768115942028985588, 0.3840579710144927383, 0.3913043478260869734, 0.3985507246376811530, 0.4057971014492753881, 0.4130434782608695676, 0.4202898550724637472, 0.4275362318840579823, 0.4347826086956521618, 0.4420289855072463969, 0.4492753623188405765, 0.4565217391304347561, 0.4637681159420289911, 0.4710144927536231707, 0.4782608695652174058, 0.4855072463768115854, 0.4927536231884058204, 0.5000000000000000000, 0.5072463768115942351, 0.5144927536231883591, 0.5217391304347825942, 0.5289855072463768293, 0.5362318840579710644, 0.5434782608695651884, 0.5507246376811594235, 0.5579710144927536586, 0.5652173913043477826, 0.5724637681159420177, 0.5797101449275362528, 0.5869565217391304879, 0.5942028985507246119, 0.6014492753623188470, 0.6086956521739130821, 0.6159420289855072062, 0.6231884057971014412, 0.6304347826086956763, 0.6376811594202898004, 0.6449275362318840354, 0.6521739130434782705, 0.6594202898550725056, 0.6666666666666666297, 0.6739130434782608647, 0.6811594202898550998, 0.6884057971014492239, 0.6956521739130434590, 0.7028985507246376940, 0.7101449275362319291, 0.7173913043478260532, 0.7246376811594202882, 0.7318840579710145233, 0.7391304347826086474, 0.7463768115942028825, 0.7536231884057971175, 0.7608695652173913526, 0.7681159420289854767, 0.7753623188405797118, 0.7826086956521739468, 0.7898550724637680709, 0.7971014492753623060, 0.8043478260869565410, 0.8115942028985507761, 0.8188405797101449002, 0.8260869565217391353, 0.8333333333333333703, 0.8405797101449274944, 0.8478260869565217295, 0.8550724637681159646, 0.8623188405797101996, 0.8695652173913043237, 0.8768115942028985588, 0.8840579710144927938, 0.8913043478260869179, 0.8985507246376811530, 0.9057971014492753881, 0.9130434782608695121, 0.9202898550724637472, 0.9275362318840579823, 0.9347826086956522174, 0.9420289855072463414, 0.9492753623188405765, 0.9565217391304348116, 0.9637681159420289356, 0.9662082973083874204 ),
 .UNSPECIFIED. ) 
 GEOMETRIC_REPRESENTATION_ITEM ( )  RATIONAL_B_SPLINE_SURFACE ( (
 ( 1.000000000000000000, 0.8660254037844387076, 1.000000000000000000, 0.8660254037844387076, 1.000000000000000000, 0.8660254037844387076, 1.000000000000000000, 0.8660254037844387076, 1.000000000000000000, 0.8660254037844387076, 1.000000000000000000, 0.8660254037844387076, 1.000000000000000000, 0.8660254037844387076, 1.000000000000000000, 0.8660254037844387076, 1.000000000000000000, 0.8660254037844387076, 1.000000000000000000, 0.8660254037844387076, 1.000000000000000000, 0.8660254037844387076, 1.000000000000000000, 0.8660254037844387076, 1.000000000000000000, 0.8660254037844387076, 1.000000000000000000, 0.8660254037844387076, 1.000000000000000000, 0.8660254037844387076, 1.000000000000000000, 0.8660254037844387076, 1.000000000000000000, 0.8660254037844387076, 1.000000000000000000, 0.8660254037844387076, 1.000000000000000000, 0.8660254037844387076, 1.000000000000000000, 0.8660254037844387076, 1.000000000000000000, 0.8660254037844387076, 1.000000000000000000, 0.8660254037844387076, 1.000000000000000000, 0.8660254037844387076, 1.000000000000000000, 0.8660254037844387076, 1.000000000000000000, 0.8660254037844387076, 1.000000000000000000, 0.8660254037844387076, 1.000000000000000000, 0.8660254037844387076, 1.000000000000000000, 0.8660254037844387076, 1.000000000000000000, 0.8660254037844387076, 1.000000000000000000, 0.8660254037844387076, 1.000000000000000000, 0.8660254037844387076, 1.000000000000000000, 0.8660254037844387076, 1.000000000000000000, 0.8660254037844387076, 1.000000000000000000, 0.8660254037844387076, 1.000000000000000000, 0.8660254037844387076, 1.000000000000000000, 0.8660254037844387076, 1.000000000000000000, 0.8660254037844387076, 1.000000000000000000, 0.8660254037844387076, 1.000000000000000000, 0.8660254037844387076, 1.000000000000000000, 0.8660254037844387076, 1.000000000000000000, 0.8660254037844387076, 1.000000000000000000, 0.8660254037844387076, 1.000000000000000000, 0.8660254037844387076, 1.000000000000000000, 0.8660254037844387076, 1.000000000000000000, 0.8660254037844387076, 1.000000000000000000, 0.8660254037844387076, 1.000000000000000000, 0.8660254037844387076, 1.000000000000000000, 0.8660254037844387076, 1.000000000000000000, 0.8660254037844387076, 1.000000000000000000, 0.8660254037844387076, 1.000000000000000000, 0.8660254037844387076, 1.000000000000000000, 0.8660254037844387076, 1.000000000000000000, 0.8660254037844387076, 1.000000000000000000, 0.8660254037844387076, 1.000000000000000000, 0.8660254037844387076, 1.000000000000000000, 0.8660254037844387076, 1.000000000000000000, 0.8660254037844387076, 1.000000000000000000, 0.8660254037844387076, 1.000000000000000000, 0.8660254037844387076, 1.000000000000000000, 0.8660254037844387076, 1.000000000000000000, 0.8660254037844387076, 1.000000000000000000, 0.8660254037844387076, 1.000000000000000000, 0.8660254037844387076, 1.000000000000000000, 0.8660254037844387076, 1.000000000000000000, 0.8660254037844387076, 1.000000000000000000, 0.8660254037844387076, 1.000000000000000000, 0.8660254037844387076, 1.000000000000000000, 0.8660254037844387076, 1.000000000000000000, 0.8660254037844387076, 1.000000000000000000, 0.8660254037844387076, 1.000000000000000000, 0.8660254037844387076, 1.000000000000000000, 0.8660254037844387076, 1.000000000000000000, 0.8660254037844387076, 1.000000000000000000, 0.8660254037844387076, 1.000000000000000000, 0.8660254037844387076, 1.000000000000000000, 0.8660254037844387076, 1.000000000000000000, 0.8660254037844387076, 1.000000000000000000, 0.8660254037844387076, 1.000000000000000000, 0.8660254037844387076, 1.000000000000000000, 0.8660254037844387076, 1.000000000000000000, 0.8660254037844387076, 1.000000000000000000, 0.8660254037844387076, 1.000000000000000000, 0.8660254037844387076, 1.000000000000000000, 0.8660254037844387076, 1.000000000000000000, 0.8660254037844387076, 1.000000000000000000, 0.8660254037844387076, 1.000000000000000000, 0.8660254037844387076, 1.000000000000000000, 0.8660254037844387076, 1.000000000000000000, 0.8660254037844387076, 1.000000000000000000, 0.8660254037844387076, 1.000000000000000000, 0.8660254037844387076, 1.000000000000000000, 0.8660254037844387076, 1.000000000000000000, 0.8660254037844387076, 1.000000000000000000, 0.8660254037844387076, 1.000000000000000000, 0.8660254037844387076, 1.000000000000000000, 0.8660254037844387076, 1.000000000000000000, 0.8660254037844387076, 1.000000000000000000, 0.8660254037844387076, 1.000000000000000000, 0.8660254037844387076, 1.000000000000000000, 0.8660254037844387076, 1.000000000000000000, 0.8660254037844387076, 1.000000000000000000, 0.8660254037844387076, 1.000000000000000000, 0.8660254037844387076, 1.000000000000000000, 0.8660254037844387076, 1.000000000000000000, 0.8660254037844387076, 1.000000000000000000, 0.8660254037844387076, 1.000000000000000000, 0.8660254037844387076, 1.000000000000000000, 0.8660254037844387076, 1.000000000000000000, 0.8660254037844387076, 1.000000000000000000, 0.8660254037844387076, 1.000000000000000000, 0.8660254037844387076, 1.000000000000000000, 0.8660254037844387076, 1.000000000000000000, 0.8660254037844387076, 1.000000000000000000, 0.8660254037844387076, 1.000000000000000000, 0.8660254037844387076, 1.000000000000000000, 0.8660254037844387076, 1.000000000000000000, 0.8660254037844387076, 1.000000000000000000, 0.8660254037844387076, 1.000000000000000000, 0.8660254037844387076, 1.000000000000000000, 0.8660254037844387076, 1.000000000000000000, 0.8660254037844387076, 1.000000000000000000, 0.8660254037844387076, 1.000000000000000000, 0.8660254037844387076, 1.000000000000000000, 0.8660254037844387076, 1.000000000000000000, 0.8660254037844387076, 1.000000000000000000, 0.8660254037844387076, 1.000000000000000000, 0.8660254037844387076, 1.000000000000000000, 0.8660254037844387076, 1.000000000000000000, 0.8660254037844387076, 1.000000000000000000, 0.8660254037844387076, 1.000000000000000000, 0.8660254037844387076, 1.000000000000000000, 0.8660254037844387076, 1.000000000000000000, 0.8660254037844387076, 1.000000000000000000, 0.9548847207714155072, 0.9401541335272467492),
 ( 1.000000000000000000, 0.8660254037844387076, 1.000000000000000000, 0.8660254037844387076, 1.000000000000000000, 0.8660254037844387076, 1.000000000000000000, 0.8660254037844387076, 1.000000000000000000, 0.8660254037844387076, 1.000000000000000000, 0.8660254037844387076, 1.000000000000000000, 0.8660254037844387076, 1.000000000000000000, 0.8660254037844387076, 1.000000000000000000, 0.8660254037844387076, 1.000000000000000000, 0.8660254037844387076, 1.000000000000000000, 0.8660254037844387076, 1.000000000000000000, 0.8660254037844387076, 1.000000000000000000, 0.8660254037844387076, 1.000000000000000000, 0.8660254037844387076, 1.000000000000000000, 0.8660254037844387076, 1.000000000000000000, 0.8660254037844387076, 1.000000000000000000, 0.8660254037844387076, 1.000000000000000000, 0.8660254037844387076, 1.000000000000000000, 0.8660254037844387076, 1.000000000000000000, 0.8660254037844387076, 1.000000000000000000, 0.8660254037844387076, 1.000000000000000000, 0.8660254037844387076, 1.000000000000000000, 0.8660254037844387076, 1.000000000000000000, 0.8660254037844387076, 1.000000000000000000, 0.8660254037844387076, 1.000000000000000000, 0.8660254037844387076, 1.000000000000000000, 0.8660254037844387076, 1.000000000000000000, 0.8660254037844387076, 1.000000000000000000, 0.8660254037844387076, 1.000000000000000000, 0.8660254037844387076, 1.000000000000000000, 0.8660254037844387076, 1.000000000000000000, 0.8660254037844387076, 1.000000000000000000, 0.8660254037844387076, 1.000000000000000000, 0.8660254037844387076, 1.000000000000000000, 0.8660254037844387076, 1.000000000000000000, 0.8660254037844387076, 1.000000000000000000, 0.8660254037844387076, 1.000000000000000000, 0.8660254037844387076, 1.000000000000000000, 0.8660254037844387076, 1.000000000000000000, 0.8660254037844387076, 1.000000000000000000, 0.8660254037844387076, 1.000000000000000000, 0.8660254037844387076, 1.000000000000000000, 0.8660254037844387076, 1.000000000000000000, 0.8660254037844387076, 1.000000000000000000, 0.8660254037844387076, 1.000000000000000000, 0.8660254037844387076, 1.000000000000000000, 0.8660254037844387076, 1.000000000000000000, 0.8660254037844387076, 1.000000000000000000, 0.8660254037844387076, 1.000000000000000000, 0.8660254037844387076, 1.000000000000000000, 0.8660254037844387076, 1.000000000000000000, 0.8660254037844387076, 1.000000000000000000, 0.8660254037844387076, 1.000000000000000000, 0.8660254037844387076, 1.000000000000000000, 0.8660254037844387076, 1.000000000000000000, 0.8660254037844387076, 1.000000000000000000, 0.8660254037844387076, 1.000000000000000000, 0.8660254037844387076, 1.000000000000000000, 0.8660254037844387076, 1.000000000000000000, 0.8660254037844387076, 1.000000000000000000, 0.8660254037844387076, 1.000000000000000000, 0.8660254037844387076, 1.000000000000000000, 0.8660254037844387076, 1.000000000000000000, 0.8660254037844387076, 1.000000000000000000, 0.8660254037844387076, 1.000000000000000000, 0.8660254037844387076, 1.000000000000000000, 0.8660254037844387076, 1.000000000000000000, 0.8660254037844387076, 1.000000000000000000, 0.8660254037844387076, 1.000000000000000000, 0.8660254037844387076, 1.000000000000000000, 0.8660254037844387076, 1.000000000000000000, 0.8660254037844387076, 1.000000000000000000, 0.8660254037844387076, 1.000000000000000000, 0.8660254037844387076, 1.000000000000000000, 0.8660254037844387076, 1.000000000000000000, 0.8660254037844387076, 1.000000000000000000, 0.8660254037844387076, 1.000000000000000000, 0.8660254037844387076, 1.000000000000000000, 0.8660254037844387076, 1.000000000000000000, 0.8660254037844387076, 1.000000000000000000, 0.8660254037844387076, 1.000000000000000000, 0.8660254037844387076, 1.000000000000000000, 0.8660254037844387076, 1.000000000000000000, 0.8660254037844387076, 1.000000000000000000, 0.8660254037844387076, 1.000000000000000000, 0.8660254037844387076, 1.000000000000000000, 0.8660254037844387076, 1.000000000000000000, 0.8660254037844387076, 1.000000000000000000, 0.8660254037844387076, 1.000000000000000000, 0.8660254037844387076, 1.000000000000000000, 0.8660254037844387076, 1.000000000000000000, 0.8660254037844387076, 1.000000000000000000, 0.8660254037844387076, 1.000000000000000000, 0.8660254037844387076, 1.000000000000000000, 0.8660254037844387076, 1.000000000000000000, 0.8660254037844387076, 1.000000000000000000, 0.8660254037844387076, 1.000000000000000000, 0.8660254037844387076, 1.000000000000000000, 0.8660254037844387076, 1.000000000000000000, 0.8660254037844387076, 1.000000000000000000, 0.8660254037844387076, 1.000000000000000000, 0.8660254037844387076, 1.000000000000000000, 0.8660254037844387076, 1.000000000000000000, 0.8660254037844387076, 1.000000000000000000, 0.8660254037844387076, 1.000000000000000000, 0.8660254037844387076, 1.000000000000000000, 0.8660254037844387076, 1.000000000000000000, 0.8660254037844387076, 1.000000000000000000, 0.8660254037844387076, 1.000000000000000000, 0.8660254037844387076, 1.000000000000000000, 0.8660254037844387076, 1.000000000000000000, 0.8660254037844387076, 1.000000000000000000, 0.8660254037844387076, 1.000000000000000000, 0.8660254037844387076, 1.000000000000000000, 0.8660254037844387076, 1.000000000000000000, 0.8660254037844387076, 1.000000000000000000, 0.8660254037844387076, 1.000000000000000000, 0.8660254037844387076, 1.000000000000000000, 0.8660254037844387076, 1.000000000000000000, 0.8660254037844387076, 1.000000000000000000, 0.8660254037844387076, 1.000000000000000000, 0.8660254037844387076, 1.000000000000000000, 0.8660254037844387076, 1.000000000000000000, 0.8660254037844387076, 1.000000000000000000, 0.8660254037844387076, 1.000000000000000000, 0.8660254037844387076, 1.000000000000000000, 0.8660254037844387076, 1.000000000000000000, 0.8660254037844387076, 1.000000000000000000, 0.8660254037844387076, 1.000000000000000000, 0.8660254037844387076, 1.000000000000000000, 0.8660254037844387076, 1.000000000000000000, 0.8660254037844387076, 1.000000000000000000, 0.8660254037844387076, 1.000000000000000000, 0.9548847207714155072, 0.9401541335272467492) ) ) 
 REPRESENTATION_ITEM ( '' )  SURFACE ( )  );
#3974=CARTESIAN_POINT ( 'NONE',  ( 26.75643035624999655, 240.0343750006145740, 3.323476615752267715 ) ) ;
#3975=VERTEX_POINT ( 'NONE', #35384 ) ;
#3979=DIRECTION ( 'NONE',  ( -1.000000000000000000, 0.000000000000000000, 0.000000000000000000 ) ) ;
#3985=VERTEX_POINT ( 'NONE', #18734 ) ;
#3987=CARTESIAN_POINT ( 'NONE',  ( 15.24356964374999990, 246.5968750006145171, 0.000000000000000000 ) ) ;
#3992=CARTESIAN_POINT ( 'NONE',  ( 20.99999999999999645, 202.0000000000000000, 0.000000000000000000 ) ) ;
#4001=CARTESIAN_POINT ( 'NONE',  ( 18.12178482187499640, 246.0718750006145115, -4.985214923628404904 ) ) ;
#4008=CARTESIAN_POINT ( 'NONE',  ( 20.99999999999998579, 247.9187500012290002, 5.999999999999998224 ) ) ;
#4012=AXIS2_PLACEMENT_3D ( 'NONE', #34312, #2285, #36776 ) ;
#4014=CARTESIAN_POINT ( 'NONE',  ( 15.00000000000000178, 246.4937500012290172, 3.464101615137757051 ) ) ;
#4021=CYLINDRICAL_SURFACE ( 'NONE', #15775, 5.999999999999999112 ) ;
#4025=CARTESIAN_POINT ( 'NONE',  ( -13.49999999999998401, 196.4750000000000227, 23.38268590217985476 ) ) ;
#4027=EDGE_CURVE ( 'NONE', #32139, #23609, #17530, .T. ) ;
#4031=CARTESIAN_POINT ( 'NONE',  ( 21.00000000000000000, 244.5437500012290286, -6.928203230275506996 ) ) ;
#4034=CARTESIAN_POINT ( 'NONE',  ( -27.24356964375000345, 199.8031250006145285, 0.000000000000000000 ) ) ;
#4038=EDGE_LOOP ( 'NONE', ( #19316, #13265 ) ) ;
#4040=CARTESIAN_POINT ( 'NONE',  ( 15.24356964375000167, 244.8343750006145285, 3.323476615752272600 ) ) ;
#4045=FILL_AREA_STYLE ('',( #824 ) ) ;
#4051=CYLINDRICAL_SURFACE ( 'NONE', #16179, 5.999999999999999112 ) ;
#4067=FACE_OUTER_BOUND ( 'NONE', #24122, .T. ) ;
#4071=CARTESIAN_POINT ( 'NONE',  ( 15.24356964374999990, 249.8593750006145342, 0.000000000000000000 ) ) ;
#4073=CARTESIAN_POINT ( 'NONE',  ( 20.99999999999999645, 244.5718750006145399, 6.646953231504538984 ) ) ;
#4082=CARTESIAN_POINT ( 'NONE',  ( -7.794113622367441430, 220.1661624776399719, 2.888482486952295591 ) ) ;
#4085=ORIENTED_EDGE ( 'NONE', *, *, #18977, .F. ) ;
#4087=CARTESIAN_POINT ( 'NONE',  ( 27.00000000000001421, 196.7000000012290286, 15.58845726811988897 ) ) ;
#4096=CARTESIAN_POINT ( 'NONE',  ( 12.98158921324744774, 213.0069040450338491, 5.206989594055764670 ) ) ;
#4103=CARTESIAN_POINT ( 'NONE',  ( 15.00000000000000178, 241.0374999999999943, 3.464101615137757051 ) ) ;
#4104=CARTESIAN_POINT ( 'NONE',  ( 27.24356964375000700, 197.7406250006145285, 15.72908226750537075 ) ) ;
#4108=EDGE_CURVE ( 'NONE', #37310, #22812, #29896, .T. ) ;
#4111=CARTESIAN_POINT ( 'NONE',  ( 10.49999999999999822, 222.9518338469886203, -2.500000000000000000 ) ) ;
#4122=FACE_OUTER_BOUND ( 'NONE', #31746, .T. ) ;
#4128=ADVANCED_FACE ( 'NONE', ( #24950 ), #21942, .F. ) ;
#4133=CARTESIAN_POINT ( 'NONE',  ( 21.00000000000000000, 246.7375000000000114, -6.928203230275506996 ) ) ;
#4134=CARTESIAN_POINT ( 'NONE',  ( 27.24356964375000700, 195.4906250006145001, 15.72908226750537075 ) ) ;
#4137=ORIENTED_EDGE ( 'NONE', *, *, #29096, .F. ) ;
#4139=CARTESIAN_POINT ( 'NONE',  ( 5.778771075727756162E-15, 196.7656250006145342, 31.45816453501075927 ) ) ;
#4140=CARTESIAN_POINT ( 'NONE',  ( 21.00000000000000000, 240.1843750006145513, -6.646953231504538984 ) ) ;
#4143=CARTESIAN_POINT ( 'NONE',  ( 26.75643035624999655, 244.7218750006145456, -3.323476615752271712 ) ) ;
#4147=EDGE_CURVE ( 'NONE', #30190, #23622, #27268, .T. ) ;
#4151=CARTESIAN_POINT ( 'NONE',  ( 26.75643035624999655, 240.1093750006145342, -3.323476615752271268 ) ) ;
#4161=CARTESIAN_POINT ( 'NONE',  ( 18.00000000000000000, 244.0749999999999886, -5.196152422706630247 ) ) ;
#4163=DIRECTION ( 'NONE',  ( -0.000000000000000000, 1.000000000000000000, -0.000000000000000000 ) ) ;
#4166=CARTESIAN_POINT ( 'NONE',  ( 21.00000000000000000, 240.6343750006145115, -6.646953231504538984 ) ) ;
#4170=CARTESIAN_POINT ( 'NONE',  ( 23.99999999999999645, 242.6500000000000057, -5.196152422706631135 ) ) ;
#4174=CARTESIAN_POINT ( 'NONE',  ( 18.12178482187499640, 243.9343750006145513, -4.985214923628404904 ) ) ;
#4179=CARTESIAN_POINT ( 'NONE',  ( 15.24356964374999990, 247.4593750006145285, -3.323476615752268604 ) ) ;
#4192=CARTESIAN_POINT ( 'NONE',  ( 26.75643035624999655, 247.6843750006145513, 3.323476615752267271 ) ) ;
#4197=( BOUNDED_CURVE ( )  B_SPLINE_CURVE ( 2, ( #248, #11812, #18082, #26779, #26588, #20172, #32464, #12187, #23759 ),
 .UNSPECIFIED., .F., .F. ) 
 B_SPLINE_CURVE_WITH_KNOTS ( ( 3, 2, 2, 2, 3 ),
 ( 0.2934782608695652439, 0.2971014492753623060, 0.3043478260869565410, 0.3115942028985507206, 0.3152173913043477826 ),
 .UNSPECIFIED. ) 
 CURVE ( )  GEOMETRIC_REPRESENTATION_ITEM ( )  RATIONAL_B_SPLINE_CURVE ( ( 0.9330127018922194093, 0.9330127018922198534, 1.000000000000000000, 0.8660254037844387076, 1.000000000000000000, 0.8660254037844387076, 1.000000000000000000, 0.9330127018922198534, 0.9330127018922191873 ) ) 
 REPRESENTATION_ITEM ( '' )  );
#4202=CARTESIAN_POINT ( 'NONE',  ( 15.00000000000000000, 241.4124999999999659, -3.464101615137752610 ) ) ;
#4208=CARTESIAN_POINT ( 'NONE',  ( 20.99999999999997513, 246.7937500012290286, -5.999999999999999112 ) ) ;
#4212=CARTESIAN_POINT ( 'NONE',  ( 27.00000000000000355, 195.7250000000000227, -3.306546357697854128E-15 ) ) ;
#4217=CARTESIAN_POINT ( 'NONE',  ( 24.00000000000000000, 244.8062500012290457, 5.196152422706629359 ) ) ;
#4225=DIRECTION ( 'NONE',  ( 0.000000000000000000, 0.000000000000000000, -1.000000000000000000 ) ) ;
#4226=CARTESIAN_POINT ( 'NONE',  ( 23.87821517812500005, 244.4968750006145228, 4.985214923628404016 ) ) ;
#4241=DIRECTION ( 'NONE',  ( 0.000000000000000000, 0.000000000000000000, 1.000000000000000000 ) ) ;
#4245=CARTESIAN_POINT ( 'NONE',  ( -28.37024444651914123, 204.7169729760873906, -6.013169554073232170 ) ) ;
#4255=CARTESIAN_POINT ( 'NONE',  ( 21.00000000000000000, 249.0718750006145399, 6.646953231504538984 ) ) ;
#4257=CARTESIAN_POINT ( 'NONE',  ( 23.87821517812500005, 244.1593750006145171, 4.985214923628404016 ) ) ;
#4259=ORIENTED_EDGE ( 'NONE', *, *, #9642, .F. ) ;
#4260=DIRECTION ( 'NONE',  ( -0.000000000000000000, 1.000000000000000000, -0.000000000000000000 ) ) ;
#4272=DIRECTION ( 'NONE',  ( -0.000000000000000000, 1.000000000000000000, -0.000000000000000000 ) ) ;
#4273=CARTESIAN_POINT ( 'NONE',  ( 22.60769515458673951, 249.2888461906613884, 5.999999999999998224 ) ) ;
#4278=CARTESIAN_POINT ( 'NONE',  ( 26.99999999999999645, 243.5687500012290343, -3.464101615137755275 ) ) ;
#4279=CARTESIAN_POINT ( 'NONE',  ( 15.00000000000000000, 243.7562500012290627, 0.000000000000000000 ) ) ;
#4289=CARTESIAN_POINT ( 'NONE',  ( -13.62178482187500528, 199.7281250006145399, -23.59362340125807123 ) ) ;
#4294=DIRECTION ( 'NONE',  ( 0.000000000000000000, -1.000000000000000000, 0.000000000000000000 ) ) ;
#4309=CYLINDRICAL_SURFACE ( 'NONE', #32457, 27.00000000000000000 ) ;
#4315=CARTESIAN_POINT ( 'NONE',  ( 26.99999999999999645, 246.6625000000000227, -3.464101615137755275 ) ) ;
#4319=ORIENTED_EDGE ( 'NONE', *, *, #28696, .F. ) ;
#4322=CARTESIAN_POINT ( 'NONE',  ( -27.00000000000000355, 199.1750000012290513, -15.58845726811989429 ) ) ;
#4326=CARTESIAN_POINT ( 'NONE',  ( 18.12178482187499640, 245.7343750006145342, -4.985214923628404904 ) ) ;
#4332=CARTESIAN_POINT ( 'NONE',  ( 23.87821517812499650, 240.1468750006145285, -4.985214923628404904 ) ) ;
#4348=CARTESIAN_POINT ( 'NONE',  ( 15.24356964374999990, 249.8593750006145342, 0.000000000000000000 ) ) ;
#4352=CARTESIAN_POINT ( 'NONE',  ( 5.778771075727756162E-15, 197.2718750006145569, 31.45816453501076637 ) ) ;
#4355=CARTESIAN_POINT ( 'NONE',  ( 18.12178482187499640, 243.4843750006145342, -4.985214923628404904 ) ) ;
#4362=CARTESIAN_POINT ( 'NONE',  ( 18.12178482187499640, 246.5218750006145001, -4.985214923628404904 ) ) ;
#4377=CARTESIAN_POINT ( 'NONE',  ( 18.12178482187499640, 247.4218750006145342, -4.985214923628404904 ) ) ;
#4379=CARTESIAN_POINT ( 'NONE',  ( -7.234628195640307347, 199.1200961906613713, -27.00000000000000711 ) ) ;
#4398=CARTESIAN_POINT ( 'NONE',  ( 13.62178482187501416, 197.7593750006145399, 23.59362340125806767 ) ) ;
#4403=CARTESIAN_POINT ( 'NONE',  ( 18.00000000000000000, 243.6812500012290457, -5.196152422706630247 ) ) ;
#4412=CARTESIAN_POINT ( 'NONE',  ( 23.87821517812499650, 244.6468750006145285, -4.985214923628404904 ) ) ;
#4424=CARTESIAN_POINT ( 'NONE',  ( 0.000000000000000000, 210.0000000000000284, -27.00000000000000000 ) ) ;
#4427=COLOUR_RGB ( '',0.8941176470588234615, 0.8941176470588234615, 0.8941176470588234615 ) ;
#4432=CARTESIAN_POINT ( 'NONE',  ( -28.72461751544321018, 203.0584876166405195, -4.011490837943430421 ) ) ;
#4433=ORIENTED_EDGE ( 'NONE', *, *, #32992, .F. ) ;
#4437=CARTESIAN_POINT ( 'NONE',  ( 24.00000000000000000, 247.4500000000000171, 5.196152422706629359 ) ) ;
#4441=AXIS2_PLACEMENT_3D ( 'NONE', #28119, #30415, #18867 ) ;
#4442=CARTESIAN_POINT ( 'NONE',  ( 21.00000000000000000, 247.4687500012290400, 5.999999999999998224 ) ) ;
#4444=CARTESIAN_POINT ( 'NONE',  ( 18.12178482187500350, 244.0843750006145285, 4.985214923628407568 ) ) ;
#4456=DIRECTION ( 'NONE',  ( 0.000000000000000000, 0.000000000000000000, -1.000000000000000000 ) ) ;
#4458=CARTESIAN_POINT ( 'NONE',  ( 24.00000000000000000, 249.3062500012290457, 5.196152422706629359 ) ) ;
#4475=CARTESIAN_POINT ( 'NONE',  ( 5.778771075727756162E-15, 196.7656250006145342, 31.45816453501075927 ) ) ;
#4478=ORIENTED_EDGE ( 'NONE', *, *, #22111, .T. ) ;
#4485=AXIS2_PLACEMENT_3D ( 'NONE', #6361, #3700, #26630 ) ;
#4495=CARTESIAN_POINT ( 'NONE',  ( 13.49999999999999645, 199.8499999999999943, -23.38268590217984766 ) ) ;
#4496=CARTESIAN_POINT ( 'NONE',  ( 22.60769515458672885, 247.4888461906613770, 5.999999999999997335 ) ) ;
#4504=CARTESIAN_POINT ( 'NONE',  ( 26.99999999999999645, 244.8249999999999886, -7.347880794884117764E-16 ) ) ;
#4506=EDGE_CURVE ( 'NONE', #2146, #12569, #26067, .T. ) ;
#4510=ORIENTED_EDGE ( 'NONE', *, *, #6847, .F. ) ;
#4511=CARTESIAN_POINT ( 'NONE',  ( -27.00000000000000355, 198.3125000012290400, 0.000000000000000000 ) ) ;
#4512=CARTESIAN_POINT ( 'NONE',  ( 19.39230484541326049, 248.6138461906613770, -5.999999999999997335 ) ) ;
#4514=( BOUNDED_CURVE ( )  B_SPLINE_CURVE ( 2, ( #31991, #516, #32364, #23657, #23466, #32548, #35200, #9250, #20823 ),
 .UNSPECIFIED., .F., .F. ) 
 B_SPLINE_CURVE_WITH_KNOTS ( ( 3, 2, 2, 2, 3 ),
 ( 0.02083333333333333565, 0.02777777777777777624, 0.04166666666666666435, 0.05555555555555555247, 0.06250000000000000000 ),
 .UNSPECIFIED. ) 
 CURVE ( )  GEOMETRIC_REPRESENTATION_ITEM ( )  RATIONAL_B_SPLINE_CURVE ( ( 0.9330127018922194093, 0.9330127018922194093, 1.000000000000000000, 0.8660254037844387076, 1.000000000000000000, 0.8660254037844387076, 1.000000000000000000, 0.9330127018922194093, 0.9330127018922194093 ) ) 
 REPRESENTATION_ITEM ( '' )  );
#4517=CARTESIAN_POINT ( 'NONE',  ( 21.00000000000000000, 245.2468750006145228, -6.646953231504538984 ) ) ;
#4523=CARTESIAN_POINT ( 'NONE',  ( -4.694659320240884604E-14, 197.8625000000000114, 27.00000000000000000 ) ) ;
#4531=EDGE_CURVE ( 'NONE', #32891, #23955, #23233, .T. ) ;
#4537=CARTESIAN_POINT ( 'NONE',  ( 21.00000000000000000, 249.2968750006145342, -6.646953231504538984 ) ) ;
#4541=CARTESIAN_POINT ( 'NONE',  ( -27.24356964375000345, 197.5718750006145115, -15.72908226750537786 ) ) ;
#4544=DIRECTION ( 'NONE',  ( -1.000000000000000000, 0.000000000000000000, 0.000000000000000000 ) ) ;
#4545=CARTESIAN_POINT ( 'NONE',  ( 18.12178482187499640, 242.5843750006145285, -4.985214923628404904 ) ) ;
#4552=CARTESIAN_POINT ( 'NONE',  ( 15.24356964375000167, 243.4843750006145058, 3.323476615752272600 ) ) ;
#4553=EDGE_CURVE ( 'NONE', #149, #20414, #27964, .T. ) ;
#4565=CARTESIAN_POINT ( 'NONE',  ( 23.87821517812499650, 245.9968750006145228, -4.985214923628404904 ) ) ;
#4567=CARTESIAN_POINT ( 'NONE',  ( -26.99999999999999645, 197.4500000012290002, 15.58845726811991561 ) ) ;
#4569=CARTESIAN_POINT ( 'NONE',  ( 18.00000000000000000, 245.8750000000000000, -5.196152422706630247 ) ) ;
#4578=CARTESIAN_POINT ( 'NONE',  ( 24.00000000000000000, 242.5562500012290457, 5.196152422706629359 ) ) ;
#4582=DIRECTION ( 'NONE',  ( 1.000000000000000000, 0.000000000000000000, 0.000000000000000000 ) ) ;
#4584=CARTESIAN_POINT ( 'NONE',  ( 23.99999999999999645, 244.0562500012290457, -5.196152422706631135 ) ) ;
#4588=CARTESIAN_POINT ( 'NONE',  ( -27.24356964375000345, 197.1593750006145456, 0.000000000000000000 ) ) ;
#4593=CARTESIAN_POINT ( 'NONE',  ( 26.99999999999999645, 240.4187500012290286, -3.464101615137755275 ) ) ;
#4596=CARTESIAN_POINT ( 'NONE',  ( 27.24356964374999635, 199.6156250006145285, -15.72908226750539029 ) ) ;
#4599=ORIENTED_EDGE ( 'NONE', *, *, #27014, .T. ) ;
#4613=CARTESIAN_POINT ( 'NONE',  ( 7.234628195640322446, 199.6825961894323598, 26.99999999999999645 ) ) ;
#4619=CARTESIAN_POINT ( 'NONE',  ( 20.99999999999999289, 244.0937500012290116, -5.999999999999997335 ) ) ;
#4627=CARTESIAN_POINT ( 'NONE',  ( 15.24356964374999990, 248.4718750006145171, -3.323476615752268604 ) ) ;
#4629=CARTESIAN_POINT ( 'NONE',  ( 18.12178482187500350, 243.6343750006145115, 4.985214923628407568 ) ) ;
#4630=ORIENTED_EDGE ( 'NONE', *, *, #11394, .T. ) ;
#4632=CARTESIAN_POINT ( 'NONE',  ( 20.99999999999999645, 185.0294372515228645, 0.000000000000000000 ) ) ;
#4638=VERTEX_POINT ( 'NONE', #31754 ) ;
#4640=ORIENTED_EDGE ( 'NONE', *, *, #22827, .F. ) ;
#4649=CARTESIAN_POINT ( 'NONE',  ( 14.14550961275805996, 216.8544903872546286, 0.3345106846866886530 ) ) ;
#4651=DIRECTION ( 'NONE',  ( 0.000000000000000000, 0.000000000000000000, 1.000000000000000000 ) ) ;
#4657=CARTESIAN_POINT ( 'NONE',  ( 13.62178482187499640, 197.4031250006145228, -23.59362340125807123 ) ) ;
#4662=CARTESIAN_POINT ( 'NONE',  ( 20.99999999999999645, 185.0294372515228645, 0.000000000000000000 ) ) ;
#4674=ADVANCED_FACE ( 'NONE', ( #14328 ), #14511, .F. ) ;
#4676=CARTESIAN_POINT ( 'NONE',  ( 5.727106289114498080E-15, 199.6625000000000227, 31.17691453623979214 ) ) ;
#4686=CARTESIAN_POINT ( 'NONE',  ( 26.99999999999999645, 246.5874999999999773, 3.464101615137751278 ) ) ;
#4691=ORIENTED_EDGE ( 'NONE', *, *, #13324, .T. ) ;
#4692=CARTESIAN_POINT ( 'NONE',  ( 13.49999999999999645, 198.6125000012290513, -23.38268590217984766 ) ) ;
#4698=CARTESIAN_POINT ( 'NONE',  ( 21.00000000000000000, 244.1218750006145513, 6.646953231504538984 ) ) ;
#4705=CARTESIAN_POINT ( 'NONE',  ( -27.24356964375000345, 198.0593750006145513, 0.000000000000000000 ) ) ;
#4720=CARTESIAN_POINT ( 'NONE',  ( 20.99999999999997513, 246.2874999999999943, -5.999999999999999112 ) ) ;
#4721=CARTESIAN_POINT ( 'NONE',  ( 26.75643035624999655, 249.1468750006145285, 3.323476615752267715 ) ) ;
#4724=AXIS2_PLACEMENT_3D ( 'NONE', #18969, #19161, #22183 ) ;
#4726=CARTESIAN_POINT ( 'NONE',  ( -27.24356964375000345, 198.9593750006145285, 0.000000000000000000 ) ) ;
#4728=( BOUNDED_CURVE ( )  B_SPLINE_CURVE ( 2, ( #21610, #33160, #4899, #16481, #7206 ),
 .UNSPECIFIED., .F., .F. ) 
 B_SPLINE_CURVE_WITH_KNOTS ( ( 3, 2, 3 ),
 ( 0.000000000000000000, 0.01388888888888888985, 0.02083333333333333565 ),
 .UNSPECIFIED. ) 
 CURVE ( )  GEOMETRIC_REPRESENTATION_ITEM ( )  RATIONAL_B_SPLINE_CURVE ( ( 1.000000000000000000, 0.8660254037844387076, 1.000000000000000000, 0.9330127018922192983, 0.9330127018922194093 ) ) 
 REPRESENTATION_ITEM ( '' )  );
#4731=CARTESIAN_POINT ( 'NONE',  ( 23.87821517812500005, 241.9093750006145456, 4.985214923628404016 ) ) ;
#4735=ORIENTED_EDGE ( 'NONE', *, *, #11334, .F. ) ;
#4737=CARTESIAN_POINT ( 'NONE',  ( 15.24356964374999990, 244.7968750006145058, 0.000000000000000000 ) ) ;
#4751=( BOUNDED_CURVE ( )  B_SPLINE_CURVE ( 2, ( #20603, #17756, #9407, #29297, #26835, #864, #12435, #19449, #30628 ),
 .UNSPECIFIED., .F., .F. ) 
 B_SPLINE_CURVE_WITH_KNOTS ( ( 3, 2, 2, 2, 3 ),
 ( 0.8541666666666667407, 0.8611111111111111605, 0.8750000000000000000, 0.8888888888888888395, 0.8958333333333333703 ),
 .UNSPECIFIED. ) 
 CURVE ( )  GEOMETRIC_REPRESENTATION_ITEM ( )  RATIONAL_B_SPLINE_CURVE ( ( 0.9330127018922192983, 0.9330127018922198534, 1.000000000000000000, 0.8660254037844387076, 1.000000000000000000, 0.8660254037844387076, 1.000000000000000000, 0.9330127018922187432, 0.9330127018922192983 ) ) 
 REPRESENTATION_ITEM ( '' )  );
#4753=CARTESIAN_POINT ( 'NONE',  ( 23.87821517812500005, 244.0468750006145058, 4.985214923628404016 ) ) ;
#4761=ADVANCED_FACE ( 'NONE', ( #23602 ), #3877, .F. ) ;
#4773=CARTESIAN_POINT ( 'NONE',  ( 27.24356964375000345, 197.3843750006145399, -3.336375036156643733E-15 ) ) ;
#4774=CARTESIAN_POINT ( 'NONE',  ( 10.89885883991209425, 194.9999999999999432, 24.98405147375524749 ) ) ;
#4777=CYLINDRICAL_SURFACE ( 'NONE', #24854, 27.00000000000000000 ) ;
#4778=VERTEX_POINT ( 'NONE', #12602 ) ;
#4779=CARTESIAN_POINT ( 'NONE',  ( 23.99999999999999645, 241.8062500012290457, -5.196152422706631135 ) ) ;
#4782=CARTESIAN_POINT ( 'NONE',  ( -13.62178482187500528, 199.2781250006145228, -23.59362340125807123 ) ) ;
#4804=CARTESIAN_POINT ( 'NONE',  ( -28.58889042833610361, 203.6434601642691007, -4.885801288223162508 ) ) ;
#4813=CARTESIAN_POINT ( 'NONE',  ( 26.75643035624999655, 248.2468750006145797, 3.323476615752267715 ) ) ;
#4815=CARTESIAN_POINT ( 'NONE',  ( 15.24356964374999990, 243.1093750006145342, 0.000000000000000000 ) ) ;
#4817=CARTESIAN_POINT ( 'NONE',  ( 23.99999999999999645, 248.5562500012290457, -5.196152422706631135 ) ) ;
#4826=ORIENTED_EDGE ( 'NONE', *, *, #19586, .T. ) ;
#4831=CARTESIAN_POINT ( 'NONE',  ( 15.24356964375000167, 249.3343750006145001, 3.323476615752272600 ) ) ;
#4837=CARTESIAN_POINT ( 'NONE',  ( 14.59897497552647394, 216.4010250244744782, -0.7232488345312202416 ) ) ;
#4844=ADVANCED_FACE ( 'NONE', ( #4067 ), #12787, .F. ) ;
#4846=CARTESIAN_POINT ( 'NONE',  ( 27.24356964375000345, 196.4281250006145569, -3.336375036156643733E-15 ) ) ;
#4850=CARTESIAN_POINT ( 'NONE',  ( -29.00000000000002487, 210.0000000000000000, 0.000000000000000000 ) ) ;
#4864=CARTESIAN_POINT ( 'NONE',  ( 26.99999999999999645, 198.4625000000000341, -15.58845726811990495 ) ) ;
#4868=CARTESIAN_POINT ( 'NONE',  ( 27.00000000000000355, 198.5375000012290627, -3.306546357697854128E-15 ) ) ;
#4871=DIRECTION ( 'NONE',  ( 0.000000000000000000, -1.000000000000000000, 0.000000000000000000 ) ) ;
#4875=CARTESIAN_POINT ( 'NONE',  ( 21.00000000000000000, 244.2624999999999886, 6.928203230275506996 ) ) ;
#4876=CARTESIAN_POINT ( 'NONE',  ( 20.99999999999999289, 248.9874999999999829, -5.999999999999997335 ) ) ;
#4880=ORIENTED_EDGE ( 'NONE', *, *, #33340, .T. ) ;
#4881=CARTESIAN_POINT ( 'NONE',  ( 27.00000000000001066, 198.5000000012290400, 15.58845726811988897 ) ) ;
#4885=CARTESIAN_POINT ( 'NONE',  ( 15.24356964374999990, 243.9718750006145456, -3.323476615752268604 ) ) ;
#4887=CARTESIAN_POINT ( 'NONE',  ( 20.00041122355693801, 239.7848985277800864, -5.668978102276318154 ) ) ;
#4891=CARTESIAN_POINT ( 'NONE',  ( -13.62178482187498396, 199.4843750006145626, 23.59362340125808188 ) ) ;
#4897=CARTESIAN_POINT ( 'NONE',  ( 20.99999999999999645, 185.0294372515228645, 0.000000000000000000 ) ) ;
#4899=CARTESIAN_POINT ( 'NONE',  ( -13.50000000000000533, 199.5875000012290457, -23.38268590217984411 ) ) ;
#4909=CARTESIAN_POINT ( 'NONE',  ( -27.24356964374999279, 198.5468750006145342, 15.72908226750539384 ) ) ;
#4912=DIRECTION ( 'NONE',  ( 1.000000000000000000, 0.000000000000000000, 0.000000000000000000 ) ) ;
#4913=CARTESIAN_POINT ( 'NONE',  ( 15.00000000000000000, 249.9625000000000057, -3.464101615137752166 ) ) ;
#4917=ORIENTED_EDGE ( 'NONE', *, *, #414, .F. ) ;
#4919=CARTESIAN_POINT ( 'NONE',  ( 21.00000000000000000, 245.1343750006145115, -6.646953231504538984 ) ) ;
#4931=CARTESIAN_POINT ( 'NONE',  ( 26.75643035624999655, 244.9843750006145342, 3.323476615752267271 ) ) ;
#4932=FACE_OUTER_BOUND ( 'NONE', #16499, .T. ) ;
#4950=CARTESIAN_POINT ( 'NONE',  ( 20.99999999999999645, 185.0294372515228645, 5.999999999999999112 ) ) ;
#4951=CARTESIAN_POINT ( 'NONE',  ( -27.24356964374999990, 198.4718750006145171, -15.72908226750537786 ) ) ;
#4954=EDGE_CURVE ( 'NONE', #3383, #37177, #27189, .T. ) ;
#4956=FACE_OUTER_BOUND ( 'NONE', #26942, .T. ) ;
#4959=CARTESIAN_POINT ( 'NONE',  ( 18.00000000000000000, 241.4312500012290457, -5.196152422706630247 ) ) ;
#4962=CARTESIAN_POINT ( 'NONE',  ( -27.24356964374999990, 198.4156250006145399, -15.72908226750537786 ) ) ;
#4969=EDGE_CURVE ( 'NONE', #24301, #23005, #6540, .T. ) ;
#4993=FACE_OUTER_BOUND ( 'NONE', #11077, .T. ) ;
#4995=CARTESIAN_POINT ( 'NONE',  ( 15.00000000000000000, 247.7125000000000057, -3.464101615137752610 ) ) ;
#4996=ADVANCED_FACE ( 'NONE', ( #21146 ), #18113, .F. ) ;
#4997=CARTESIAN_POINT ( 'NONE',  ( 26.75643035624999655, 247.4218750006145058, -3.323476615752271712 ) ) ;
#4999=CARTESIAN_POINT ( 'NONE',  ( 15.24356964374999990, 241.7218750006145456, -3.323476615752268604 ) ) ;
#5003=CARTESIAN_POINT ( 'NONE',  ( 21.00000000000000000, 248.8187500012290627, 6.928203230275506996 ) ) ;
#5008=CARTESIAN_POINT ( 'NONE',  ( 26.99999999999999645, 240.8687500012290457, -3.464101615137755275 ) ) ;
#5011=ORIENTED_EDGE ( 'NONE', *, *, #586, .T. ) ;
#5014=ORIENTED_EDGE ( 'NONE', *, *, #24856, .T. ) ;
#5019=CARTESIAN_POINT ( 'NONE',  ( 23.87821517812499650, 248.2468750006145228, -4.985214923628404904 ) ) ;
#5023=CARTESIAN_POINT ( 'NONE',  ( 14.34881165084746613, 216.6511883491593835, 0.6450403596531998351 ) ) ;
#5032=CARTESIAN_POINT ( 'NONE',  ( -13.62178482187500528, 195.6781250006145569, -23.59362340125807123 ) ) ;
#5043=EDGE_CURVE ( 'NONE', #32797, #21280, #5072, .T. ) ;
#5046=CARTESIAN_POINT ( 'NONE',  ( 20.99999999999997513, 246.2874999999999943, -5.999999999999999112 ) ) ;
#5049=CARTESIAN_POINT ( 'NONE',  ( 13.49999999999999645, 198.9500000000000171, -23.38268590217984766 ) ) ;
#5053=CARTESIAN_POINT ( 'NONE',  ( 23.87821517812500005, 247.7593750006145399, 4.985214923628404016 ) ) ;
#5061=CARTESIAN_POINT ( 'NONE',  ( 18.00000000000000355, 243.7750000000000057, 5.196152422706632912 ) ) ;
#5067=CARTESIAN_POINT ( 'NONE',  ( -13.49999999999998401, 195.6875000012290400, 23.38268590217985476 ) ) ;
#5071=CARTESIAN_POINT ( 'NONE',  ( 15.24356964375000167, 242.6968750006145399, 3.323476615752272600 ) ) ;
#5072=CIRCLE ( 'NONE', #4441, 28.99999999999999645 ) ;
#5078=CARTESIAN_POINT ( 'NONE',  ( 27.24356964375000700, 199.1468750006145285, 15.72908226750537075 ) ) ;
#5085=CARTESIAN_POINT ( 'NONE',  ( 20.99999999999997868, 245.1625000000000227, 5.999999999999999112 ) ) ;
#5092=EDGE_CURVE ( 'NONE', #13079, #24290, #35304, .T. ) ;
#5095=CARTESIAN_POINT ( 'NONE',  ( 22.60769515458672885, 248.5736538117967314, -5.999999999999998224 ) ) ;
#5099=CARTESIAN_POINT ( 'NONE',  ( -13.62178482187500528, 197.0843750006145285, -23.59362340125807123 ) ) ;
#5103=CARTESIAN_POINT ( 'NONE',  ( 15.24356964374999990, 240.4093750006145456, 0.000000000000000000 ) ) ;
#5109=VECTOR ( 'NONE', #22448, 1000.000000000000000 ) ;
#5110=CARTESIAN_POINT ( 'NONE',  ( 15.24356964374999990, 245.6593750006145171, -3.323476615752268604 ) ) ;
#5121=CARTESIAN_POINT ( 'NONE',  ( 26.75643035624999655, 244.1218750006145228, -7.049594010296217766E-16 ) ) ;
#5137=DIRECTION ( 'NONE',  ( 0.000000000000000000, 0.000000000000000000, 1.000000000000000000 ) ) ;
#5139=CARTESIAN_POINT ( 'NONE',  ( 20.99999999999995381, 242.5187500012290513, 5.999999999999998224 ) ) ;
#5140=CARTESIAN_POINT ( 'NONE',  ( -27.24356964375000345, 198.9593750006145285, 0.000000000000000000 ) ) ;
#5146=CARTESIAN_POINT ( 'NONE',  ( 23.99999999999999645, 242.7062500012290513, -5.196152422706631135 ) ) ;
#5162=( BOUNDED_CURVE ( )  B_SPLINE_CURVE ( 2, ( #22040, #24870, #19017, #15983, #19572, #1927, #13311, #28083, #2115 ),
 .UNSPECIFIED., .F., .F. ) 
 B_SPLINE_CURVE_WITH_KNOTS ( ( 3, 2, 2, 2, 3 ),
 ( 0.7500000000000000000, 0.7536231884057971175, 0.7608695652173913526, 0.7681159420289854767, 0.7717391304347825942 ),
 .UNSPECIFIED. ) 
 CURVE ( )  GEOMETRIC_REPRESENTATION_ITEM ( )  RATIONAL_B_SPLINE_CURVE ( ( 0.9330127018922194093, 0.9330127018922194093, 1.000000000000000000, 0.8660254037844387076, 1.000000000000000000, 0.8660254037844387076, 1.000000000000000000, 0.9330127018922194093, 0.9330127018922194093 ) ) 
 REPRESENTATION_ITEM ( '' )  );
#5164=ORIENTED_EDGE ( 'NONE', *, *, #13324, .F. ) ;
#5166=CARTESIAN_POINT ( 'NONE',  ( 20.99999999999999645, 202.0000000000000000, 0.000000000000000000 ) ) ;
#5185=( BOUNDED_CURVE ( )  B_SPLINE_CURVE ( 2, ( #18949, #12869, #9465, #15722, #27272, #29930, #16098, #36167, #4523 ),
 .UNSPECIFIED., .F., .F. ) 
 B_SPLINE_CURVE_WITH_KNOTS ( ( 3, 2, 2, 2, 3 ),
 ( 0.3541666666666666852, 0.3611111111111111049, 0.3750000000000000000, 0.3888888888888888951, 0.3958333333333333703 ),
 .UNSPECIFIED. ) 
 CURVE ( )  GEOMETRIC_REPRESENTATION_ITEM ( )  RATIONAL_B_SPLINE_CURVE ( ( 0.9330127018922194093, 0.9330127018922196314, 1.000000000000000000, 0.8660254037844387076, 1.000000000000000000, 0.8660254037844387076, 1.000000000000000000, 0.9330127018922190762, 0.9330127018922194093 ) ) 
 REPRESENTATION_ITEM ( '' )  );
#5186=CARTESIAN_POINT ( 'NONE',  ( 15.24356964374999990, 246.7093750006145569, 0.000000000000000000 ) ) ;
#5188=CARTESIAN_POINT ( 'NONE',  ( 15.24356964375000167, 241.3468750006145171, 3.323476615752272600 ) ) ;
#5192=CARTESIAN_POINT ( 'NONE',  ( -7.234628195640313564, 199.9075961894323541, -27.00000000000000355 ) ) ;
#5200=ORIENTED_EDGE ( 'NONE', *, *, #1973, .T. ) ;
#5203=FACE_OUTER_BOUND ( 'NONE', #11385, .T. ) ;
#5208=CARTESIAN_POINT ( 'NONE',  ( 15.20136072254643977, 225.4630380732105550, 1.553813268098316769 ) ) ;
#5210=DIRECTION ( 'NONE',  ( -0.000000000000000000, 1.000000000000000000, -0.000000000000000000 ) ) ;
#5218=CARTESIAN_POINT ( 'NONE',  ( 13.62178482187501416, 196.8031250006145285, 23.59362340125806767 ) ) ;
#5237=CARTESIAN_POINT ( 'NONE',  ( 27.00000000000000355, 197.9750000000000227, -3.306546357697854128E-15 ) ) ;
#5241=CARTESIAN_POINT ( 'NONE',  ( 15.24356964374999990, 248.5093750006145399, 0.000000000000000000 ) ) ;
#5248=CARTESIAN_POINT ( 'NONE',  ( 15.00000000000000000, 244.1124999999999829, -3.464101615137752166 ) ) ;
#5250=EDGE_CURVE ( 'NONE', #29663, #5512, #24613, .T. ) ;
#5254=CARTESIAN_POINT ( 'NONE',  ( -27.00000000000000355, 194.7125000012290172, 0.000000000000000000 ) ) ;
#5258=CARTESIAN_POINT ( 'NONE',  ( 26.75643035624999655, 241.9468750006145683, 3.323476615752267715 ) ) ;
#5267=CARTESIAN_POINT ( 'NONE',  ( 5.778771075727756162E-15, 197.7218750006145456, 31.45816453501075927 ) ) ;
#5271=CARTESIAN_POINT ( 'NONE',  ( 24.00000000000000000, 245.1999999999999886, 5.196152422706629359 ) ) ;
#5280=CARTESIAN_POINT ( 'NONE',  ( 21.00000000000000000, 240.2687500012290513, 5.999999999999998224 ) ) ;
#5281=EDGE_LOOP ( 'NONE', ( #11172, #31588, #18795, #2024 ) ) ;
#5284=CARTESIAN_POINT ( 'NONE',  ( 5.778771075727756162E-15, 196.3718750006145513, 31.45816453501076637 ) ) ;
#5288=CARTESIAN_POINT ( 'NONE',  ( 15.24356964374999990, 240.8218750006145399, -3.323476615752268604 ) ) ;
#5289=CARTESIAN_POINT ( 'NONE',  ( -1.926257025242585782E-15, 199.2406250006145285, -31.45816453501076637 ) ) ;
#5294=CARTESIAN_POINT ( 'NONE',  ( 21.00000000000000000, 244.2343750006145626, -6.646953231504538984 ) ) ;
#5296=EDGE_CURVE ( 'NONE', #23197, #10569, #26255, .T. ) ;
#5309=CARTESIAN_POINT ( 'NONE',  ( 26.75643035624999655, 245.4343750006145228, 3.323476615752267271 ) ) ;
#5326=CARTESIAN_POINT ( 'NONE',  ( -4.500000000000002665, 244.5000000000000000, -2.500000000000000000 ) ) ;
#5329=CARTESIAN_POINT ( 'NONE',  ( 27.24356964375000345, 196.0343750006145456, -3.336375036156643733E-15 ) ) ;
#5330=CARTESIAN_POINT ( 'NONE',  ( 20.99999999999997868, 210.0000000000000000, 0.000000000000000000 ) ) ;
#5335=CARTESIAN_POINT ( 'NONE',  ( 23.99999999999999645, 242.2562500012290627, -5.196152422706631135 ) ) ;
#5351=ORIENTED_EDGE ( 'NONE', *, *, #19209, .T. ) ;
#5366=CARTESIAN_POINT ( 'NONE',  ( 19.39230484541326049, 240.0638461906613941, -5.999999999999997335 ) ) ;
#5367=CARTESIAN_POINT ( 'NONE',  ( 23.87821517812500005, 247.3093750006145228, 4.985214923628404016 ) ) ;
#5369=CARTESIAN_POINT ( 'NONE',  ( 20.99999999999999645, 241.8718750006145228, 6.646953231504538984 ) ) ;
#5372=DIRECTION ( 'NONE',  ( 0.000000000000000000, 0.000000000000000000, 1.000000000000000000 ) ) ;
#5373=CARTESIAN_POINT ( 'NONE',  ( 26.99999999999999645, 248.9687500012290116, -3.464101615137755275 ) ) ;
#5379=ORIENTED_EDGE ( 'NONE', *, *, #31383, .T. ) ;
#5380=ORIENTED_EDGE ( 'NONE', *, *, #8349, .T. ) ;
#5385=CARTESIAN_POINT ( 'NONE',  ( 15.24356964374999990, 248.3593750006145342, -3.323476615752268604 ) ) ;
#5389=CARTESIAN_POINT ( 'NONE',  ( 14.68278727570621633, 216.3172127243001910, 0.6964482669446712126 ) ) ;
#5400=CARTESIAN_POINT ( 'NONE',  ( 21.00000000000000000, 242.0687500012289775, 5.999999999999998224 ) ) ;
#5404=( BOUNDED_SURFACE ( )  B_SPLINE_SURFACE ( 1, 2, ( 
 ( #4034, #27162, #27723, #19023, #30580, #4596, #16173, #1185, #12759, #1753, #18267, #29811, #31816, #28090, #4782, #19214, #25949, #14579, #29151, #26131, #7823, #34658, #14392, #2122, #13699, #3192, #3009, #14768, #20465, #5852, #10469, #16356, #25250, #13503, #163, #36426, #30760, #4962, #22047, #27904, #22234, #1935, #33598, #10655, #34848, #11362, #20088, #25061, #36800, #36614, #8703, #22933, #33785, #32005, #17430, #8886, #19400, #31632, #34478, #5662, #8521, #17242, #30944, #20277, #7637, #6035, #37492, #16544, #28784, #2821, #11543, #11729, #23115, #28969, #23301, #17622, #23482, #6606, #21029, #35402, #6793, #4139, #26313, #718, #14953, #35034, #29916, #9452, #9079, #23672, #15522, #35783, #6997, #9266, #32943, #9825, #26882, #913, #30108, #12482, #35217, #20838, #21403, #24237, #24050, #32381, #29722, #9640, #27076, #26501, #12291, #29536, #26689, #3576, #12098, #32195, #6229, #1102, #18368, #17803, #12670, #6419, #32565, #15136, #11915, #20649, #23863, #350, #531, #29345, #17992, #18567, #35596, #3384, #18181 ),
 ( #21217, #3756, #32757, #15330, #3946, #16087, #27446, #27823, #24969, #27262, #1477, #21592, #30296, #4322, #33883, #13241, #1666, #33696, #16461, #15900, #33140, #10571, #27637, #7366, #22149, #18937, #7184, #35973, #4692, #30856, #7925, #4881, #24607, #13421, #30676, #30490, #4511, #19499, #19318, #31046, #36719, #7735, #1286, #18754, #24790, #13051, #28005, #15711, #10010, #21776, #12857, #36156, #10202, #33326, #24425, #36341, #13616, #10386, #21962, #33507, #7552, #19126, #36528, #16275, #1852, #10759, #2037, #25164, #22331, #37271, #34252, #11318, #17011, #2593, #36897, #25904, #2220, #16648, #5430, #8474, #19867, #37085, #23068, #31410, #28552, #22886, #14164, #34436, #31591, #20046, #5614, #16830, #17199, #25718, #2408, #8845, #31772, #14350, #10945, #28738, #2777, #22519, #11500, #20417, #28191, #5804, #5067, #17386, #13802, #37451, #28372, #34615, #8658, #8114, #25351, #8295, #20228, #13981, #28927, #14531, #23256, #25533, #11682, #26087, #2963, #117, #34065, #34801, #11132, #22710, #19686, #31225, #5254, #3334, #35355 ) ),
 .UNSPECIFIED., .F., .F., .F. ) 
 B_SPLINE_SURFACE_WITH_KNOTS ( ( 2, 2 ),
 ( 3, 2, 2, 2, 2, 2, 2, 2, 2, 2, 2, 2, 2, 2, 2, 2, 2, 2, 2, 2, 2, 2, 2, 2, 2, 2, 2, 2, 2, 2, 2, 2, 2, 2, 2, 2, 2, 2, 2, 2, 2, 2, 2, 2, 2, 2, 2, 2, 2, 2, 2, 2, 2, 2, 2, 2, 2, 2, 2, 2, 2, 2, 2, 2, 2, 2, 2, 3 ),
 ( 0.000000000000000000, 1.000000000000000000 ),
 ( 0.000000000000000000, 0.01388888888888888812, 0.02777777777777777624, 0.04166666666666666435, 0.05555555555555555247, 0.06944444444444444753, 0.08333333333333332871, 0.09722222222222222376, 0.1111111111111111049, 0.1250000000000000000, 0.1388888888888888951, 0.1527777777777777901, 0.1666666666666666574, 0.1805555555555555525, 0.1944444444444444475, 0.2083333333333333426, 0.2222222222222222099, 0.2361111111111111049, 0.2500000000000000000, 0.2638888888888888951, 0.2777777777777777901, 0.2916666666666666852, 0.3055555555555555802, 0.3194444444444444198, 0.3333333333333333148, 0.3472222222222222099, 0.3611111111111111049, 0.3750000000000000000, 0.3888888888888888951, 0.4027777777777777901, 0.4166666666666666852, 0.4305555555555555802, 0.4444444444444444198, 0.4583333333333333148, 0.4722222222222222099, 0.4861111111111111049, 0.5000000000000000000, 0.5138888888888888395, 0.5277777777777777901, 0.5416666666666666297, 0.5555555555555555802, 0.5694444444444444198, 0.5833333333333333703, 0.5972222222222222099, 0.6111111111111111605, 0.6250000000000000000, 0.6388888888888888395, 0.6527777777777777901, 0.6666666666666666297, 0.6805555555555555802, 0.6944444444444444198, 0.7083333333333333703, 0.7222222222222222099, 0.7361111111111111605, 0.7500000000000000000, 0.7638888888888888395, 0.7777777777777777901, 0.7916666666666666297, 0.8055555555555555802, 0.8194444444444444198, 0.8333333333333333703, 0.8472222222222222099, 0.8611111111111111605, 0.8750000000000000000, 0.8888888888888888395, 0.9027777777777777901, 0.9166666666666666297, 0.9258785558287927486 ),
 .UNSPECIFIED. ) 
 GEOMETRIC_REPRESENTATION_ITEM ( )  RATIONAL_B_SPLINE_SURFACE ( (
 ( 1.000000000000000000, 0.8660254037844387076, 1.000000000000000000, 0.8660254037844387076, 1.000000000000000000, 0.8660254037844387076, 1.000000000000000000, 0.8660254037844387076, 1.000000000000000000, 0.8660254037844387076, 1.000000000000000000, 0.8660254037844387076, 1.000000000000000000, 0.8660254037844387076, 1.000000000000000000, 0.8660254037844387076, 1.000000000000000000, 0.8660254037844387076, 1.000000000000000000, 0.8660254037844387076, 1.000000000000000000, 0.8660254037844387076, 1.000000000000000000, 0.8660254037844387076, 1.000000000000000000, 0.8660254037844387076, 1.000000000000000000, 0.8660254037844387076, 1.000000000000000000, 0.8660254037844387076, 1.000000000000000000, 0.8660254037844387076, 1.000000000000000000, 0.8660254037844387076, 1.000000000000000000, 0.8660254037844387076, 1.000000000000000000, 0.8660254037844387076, 1.000000000000000000, 0.8660254037844387076, 1.000000000000000000, 0.8660254037844387076, 1.000000000000000000, 0.8660254037844387076, 1.000000000000000000, 0.8660254037844387076, 1.000000000000000000, 0.8660254037844387076, 1.000000000000000000, 0.8660254037844387076, 1.000000000000000000, 0.8660254037844387076, 1.000000000000000000, 0.8660254037844387076, 1.000000000000000000, 0.8660254037844387076, 1.000000000000000000, 0.8660254037844387076, 1.000000000000000000, 0.8660254037844387076, 1.000000000000000000, 0.8660254037844387076, 1.000000000000000000, 0.8660254037844387076, 1.000000000000000000, 0.8660254037844387076, 1.000000000000000000, 0.8660254037844387076, 1.000000000000000000, 0.8660254037844387076, 1.000000000000000000, 0.8660254037844387076, 1.000000000000000000, 0.8660254037844387076, 1.000000000000000000, 0.8660254037844387076, 1.000000000000000000, 0.8660254037844387076, 1.000000000000000000, 0.8660254037844387076, 1.000000000000000000, 0.8660254037844387076, 1.000000000000000000, 0.8660254037844387076, 1.000000000000000000, 0.8660254037844387076, 1.000000000000000000, 0.8660254037844387076, 1.000000000000000000, 0.8660254037844387076, 1.000000000000000000, 0.8660254037844387076, 1.000000000000000000, 0.8660254037844387076, 1.000000000000000000, 0.8660254037844387076, 1.000000000000000000, 0.8660254037844387076, 1.000000000000000000, 0.8660254037844387076, 1.000000000000000000, 0.8660254037844387076, 1.000000000000000000, 0.8660254037844387076, 1.000000000000000000, 0.8660254037844387076, 1.000000000000000000, 0.8660254037844387076, 1.000000000000000000, 0.8660254037844387076, 1.000000000000000000, 0.8660254037844387076, 1.000000000000000000, 0.8660254037844387076, 1.000000000000000000, 0.8660254037844387076, 1.000000000000000000, 0.8660254037844387076, 1.000000000000000000, 0.8660254037844387076, 1.000000000000000000, 0.8660254037844387076, 1.000000000000000000, 0.8660254037844387076, 1.000000000000000000, 0.8660254037844387076, 1.000000000000000000, 0.8660254037844387076, 1.000000000000000000, 0.8660254037844387076, 1.000000000000000000, 0.8660254037844387076, 1.000000000000000000, 0.9111405425767590271, 0.9401542252352144136),
 ( 1.000000000000000000, 0.8660254037844387076, 1.000000000000000000, 0.8660254037844387076, 1.000000000000000000, 0.8660254037844387076, 1.000000000000000000, 0.8660254037844387076, 1.000000000000000000, 0.8660254037844387076, 1.000000000000000000, 0.8660254037844387076, 1.000000000000000000, 0.8660254037844387076, 1.000000000000000000, 0.8660254037844387076, 1.000000000000000000, 0.8660254037844387076, 1.000000000000000000, 0.8660254037844387076, 1.000000000000000000, 0.8660254037844387076, 1.000000000000000000, 0.8660254037844387076, 1.000000000000000000, 0.8660254037844387076, 1.000000000000000000, 0.8660254037844387076, 1.000000000000000000, 0.8660254037844387076, 1.000000000000000000, 0.8660254037844387076, 1.000000000000000000, 0.8660254037844387076, 1.000000000000000000, 0.8660254037844387076, 1.000000000000000000, 0.8660254037844387076, 1.000000000000000000, 0.8660254037844387076, 1.000000000000000000, 0.8660254037844387076, 1.000000000000000000, 0.8660254037844387076, 1.000000000000000000, 0.8660254037844387076, 1.000000000000000000, 0.8660254037844387076, 1.000000000000000000, 0.8660254037844387076, 1.000000000000000000, 0.8660254037844387076, 1.000000000000000000, 0.8660254037844387076, 1.000000000000000000, 0.8660254037844387076, 1.000000000000000000, 0.8660254037844387076, 1.000000000000000000, 0.8660254037844387076, 1.000000000000000000, 0.8660254037844387076, 1.000000000000000000, 0.8660254037844387076, 1.000000000000000000, 0.8660254037844387076, 1.000000000000000000, 0.8660254037844387076, 1.000000000000000000, 0.8660254037844387076, 1.000000000000000000, 0.8660254037844387076, 1.000000000000000000, 0.8660254037844387076, 1.000000000000000000, 0.8660254037844387076, 1.000000000000000000, 0.8660254037844387076, 1.000000000000000000, 0.8660254037844387076, 1.000000000000000000, 0.8660254037844387076, 1.000000000000000000, 0.8660254037844387076, 1.000000000000000000, 0.8660254037844387076, 1.000000000000000000, 0.8660254037844387076, 1.000000000000000000, 0.8660254037844387076, 1.000000000000000000, 0.8660254037844387076, 1.000000000000000000, 0.8660254037844387076, 1.000000000000000000, 0.8660254037844387076, 1.000000000000000000, 0.8660254037844387076, 1.000000000000000000, 0.8660254037844387076, 1.000000000000000000, 0.8660254037844387076, 1.000000000000000000, 0.8660254037844387076, 1.000000000000000000, 0.8660254037844387076, 1.000000000000000000, 0.8660254037844387076, 1.000000000000000000, 0.8660254037844387076, 1.000000000000000000, 0.8660254037844387076, 1.000000000000000000, 0.8660254037844387076, 1.000000000000000000, 0.8660254037844387076, 1.000000000000000000, 0.8660254037844387076, 1.000000000000000000, 0.8660254037844387076, 1.000000000000000000, 0.8660254037844387076, 1.000000000000000000, 0.8660254037844387076, 1.000000000000000000, 0.8660254037844387076, 1.000000000000000000, 0.8660254037844387076, 1.000000000000000000, 0.8660254037844387076, 1.000000000000000000, 0.8660254037844387076, 1.000000000000000000, 0.9111405425767590271, 0.9401542252352144136) ) ) 
 REPRESENTATION_ITEM ( '' )  SURFACE ( )  );
#5413=CARTESIAN_POINT ( 'NONE',  ( -26.99999999999998934, 197.7875000000000227, 15.58845726811991561 ) ) ;
#5417=CARTESIAN_POINT ( 'NONE',  ( 18.12178482187500350, 249.4843750006145342, 4.985214923628407568 ) ) ;
#5418=ORIENTED_EDGE ( 'NONE', *, *, #32767, .T. ) ;
#5420=CARTESIAN_POINT ( 'NONE',  ( 20.99999999999999289, 243.5874999999999488, -5.999999999999997335 ) ) ;
#5424=CARTESIAN_POINT ( 'NONE',  ( 15.00000000000000000, 244.5625000000000000, -3.464101615137752166 ) ) ;
#5430=CARTESIAN_POINT ( 'NONE',  ( 27.00000000000000355, 196.7375000012290229, -3.306546357697854128E-15 ) ) ;
#5434=CARTESIAN_POINT ( 'NONE',  ( 18.12178482187499640, 243.9343750006145513, -4.985214923628404904 ) ) ;
#5443=CARTESIAN_POINT ( 'NONE',  ( 5.778771075727756162E-15, 197.2718750006145569, 31.45816453501075927 ) ) ;
#5445=( BOUNDED_CURVE ( )  B_SPLINE_CURVE ( 2, ( #11562, #2650, #23135, #20294, #5868, #26149, #25145, #22131, #10739 ),
 .UNSPECIFIED., .F., .F. ) 
 B_SPLINE_CURVE_WITH_KNOTS ( ( 3, 2, 2, 2, 3 ),
 ( 0.1458333333333333426, 0.1527777777777777901, 0.1666666666666666574, 0.1805555555555555525, 0.1875000000000000000 ),
 .UNSPECIFIED. ) 
 CURVE ( )  GEOMETRIC_REPRESENTATION_ITEM ( )  RATIONAL_B_SPLINE_CURVE ( ( 0.9330127018922194093, 0.9330127018922194093, 1.000000000000000000, 0.8660254037844387076, 1.000000000000000000, 0.8660254037844387076, 1.000000000000000000, 0.9330127018922194093, 0.9330127018922194093 ) ) 
 REPRESENTATION_ITEM ( '' )  );
#5458=CARTESIAN_POINT ( 'NONE',  ( 23.99999999999999645, 248.9500000000000171, -5.196152422706631135 ) ) ;
#5463=CARTESIAN_POINT ( 'NONE',  ( 27.24356964375000700, 195.5468750006145342, 15.72908226750537075 ) ) ;
#5468=CARTESIAN_POINT ( 'NONE',  ( 21.00000000000000000, 249.8875000000000171, -6.928203230275506996 ) ) ;
#5469=CARTESIAN_POINT ( 'NONE',  ( -1.926257025242585782E-15, 198.7906250006145399, -31.45816453501076637 ) ) ;
#5474=ORIENTED_EDGE ( 'NONE', *, *, #3801, .T. ) ;
#5475=CARTESIAN_POINT ( 'NONE',  ( 18.12178482187499640, 242.9218750006145058, -4.985214923628404904 ) ) ;
#5483=CARTESIAN_POINT ( 'NONE',  ( 15.24356964374999990, 244.7593750006145115, -3.323476615752268604 ) ) ;
#5495=CARTESIAN_POINT ( 'NONE',  ( 0.000000000000000000, 195.0000000000000000, 0.000000000000000000 ) ) ;
#5500=ORIENTED_EDGE ( 'NONE', *, *, #4969, .T. ) ;
#5506=CARTESIAN_POINT ( 'NONE',  ( 20.99999999999997513, 245.8937500012290798, -5.999999999999999112 ) ) ;
#5507=CARTESIAN_POINT ( 'NONE',  ( 27.24356964375000345, 195.1343750006145399, -3.336375036156643733E-15 ) ) ;
#5512=VERTEX_POINT ( 'NONE', #20349 ) ;
#5513=CARTESIAN_POINT ( 'NONE',  ( 18.12178482187500350, 248.9218750006145342, 4.985214923628407568 ) ) ;
#5519=ORIENTED_EDGE ( 'NONE', *, *, #35989, .T. ) ;
#5547=CARTESIAN_POINT ( 'NONE',  ( 20.99999999999999645, 185.0294372515228645, 0.000000000000000000 ) ) ;
#5548=DIRECTION ( 'NONE',  ( -0.000000000000000000, -1.000000000000000000, -0.000000000000000000 ) ) ;
#5549=CARTESIAN_POINT ( 'NONE',  ( 26.75643035624999655, 245.6218750006145513, -3.323476615752271712 ) ) ;
#5551=CARTESIAN_POINT ( 'NONE',  ( 26.75643035624999655, 242.4343750006145513, -7.049594010296217766E-16 ) ) ;
#5552=VERTEX_POINT ( 'NONE', #799 ) ;
#5555=CARTESIAN_POINT ( 'NONE',  ( 26.99999999999999645, 248.8937500012290229, 3.464101615137751278 ) ) ;
#5569=CARTESIAN_POINT ( 'NONE',  ( 18.12178482187499640, 247.8718750006145228, -4.985214923628404904 ) ) ;
#5572=CARTESIAN_POINT ( 'NONE',  ( 19.95279056986836963, 210.3927035363167022, -5.999999999999998224 ) ) ;
#5583=ORIENTED_EDGE ( 'NONE', *, *, #175, .F. ) ;
#5593=AXIS2_PLACEMENT_3D ( 'NONE', #34978, #26823, #12424 ) ;
#5594=CARTESIAN_POINT ( 'NONE',  ( 15.00000000000000000, 243.3062500012290457, 0.000000000000000000 ) ) ;
#5596=CARTESIAN_POINT ( 'NONE',  ( -27.00000000000000355, 199.0625000000000000, -15.58845726811989429 ) ) ;
#5597=CARTESIAN_POINT ( 'NONE',  ( 18.00000000000000000, 240.0249999999999773, -5.196152422706630247 ) ) ;
#5599=CARTESIAN_POINT ( 'NONE',  ( 20.99999999999999645, 248.3968750006145569, -6.646953231504538984 ) ) ;
#5608=CARTESIAN_POINT ( 'NONE',  ( 21.00000000000000000, 242.4624999999999773, 6.928203230275506996 ) ) ;
#5614=CARTESIAN_POINT ( 'NONE',  ( 27.00000000000000355, 196.2875000012290343, -3.306546357697854128E-15 ) ) ;
#5619=CARTESIAN_POINT ( 'NONE',  ( 18.12178482187500350, 243.6343750006145115, 4.985214923628407568 ) ) ;
#5627=CARTESIAN_POINT ( 'NONE',  ( 27.08132523266538172, 194.9999999999999432, -1.221504123172654444 ) ) ;
#5628=CARTESIAN_POINT ( 'NONE',  ( -27.24356964374999635, 197.1968750006145115, 15.72908226750539384 ) ) ;
#5634=CARTESIAN_POINT ( 'NONE',  ( 20.99999999999999645, 185.0294372515228645, -5.999999999999999112 ) ) ;
#5635=CARTESIAN_POINT ( 'NONE',  ( 21.00000000000001066, 247.4124999999999943, 5.999999999999998224 ) ) ;
#5640=CARTESIAN_POINT ( 'NONE',  ( 27.00000000000000355, 197.1875000012290400, -3.306546357697854128E-15 ) ) ;
#5645=CARTESIAN_POINT ( 'NONE',  ( 26.99999999999999645, 249.7750000000000057, -7.347880794884117764E-16 ) ) ;
#5647=ORIENTED_EDGE ( 'NONE', *, *, #8088, .F. ) ;
#5653=LINE ( 'NONE', #34651, #18679 ) ;
#5654=CARTESIAN_POINT ( 'NONE',  ( 15.24356964374999990, 241.2718750006145569, -3.323476615752268604 ) ) ;
#5655=CARTESIAN_POINT ( 'NONE',  ( 5.778771075727756162E-15, 198.5656250006145456, 31.45816453501076637 ) ) ;
#5662=CARTESIAN_POINT ( 'NONE',  ( -27.24356964374999635, 197.5906250006145228, 15.72908226750539384 ) ) ;
#5663=CARTESIAN_POINT ( 'NONE',  ( 21.00000000000000000, 242.8843750006145399, -6.646953231504538984 ) ) ;
#5664=CARTESIAN_POINT ( 'NONE',  ( 19.39230484541326760, 243.7924038105676630, 5.999999999999999112 ) ) ;
#5672=CARTESIAN_POINT ( 'NONE',  ( 18.12178482187499640, 241.5718750006145399, -4.985214923628404904 ) ) ;
#5682=CARTESIAN_POINT ( 'NONE',  ( 20.99999999999999645, 185.0294372515228645, 5.999999999999999112 ) ) ;
#5683=EDGE_CURVE ( 'NONE', #32891, #37310, #2571, .T. ) ;
#5686=ORIENTED_EDGE ( 'NONE', *, *, #3559, .F. ) ;
#5692=EDGE_CURVE ( 'NONE', #34895, #529, #35482, .T. ) ;
#5697=CARTESIAN_POINT ( 'NONE',  ( -3.656739830522513390, 194.9999999999999716, 27.01108501465073886 ) ) ;
#5700=ORIENTED_EDGE ( 'NONE', *, *, #4108, .F. ) ;
#5702=CARTESIAN_POINT ( 'NONE',  ( 18.12178482187499640, 248.7718750006145001, -4.985214923628404904 ) ) ;
#5714=CARTESIAN_POINT ( 'NONE',  ( -13.08024444877374748, 195.0000000000000000, 23.89571502063673591 ) ) ;
#5720=CARTESIAN_POINT ( 'NONE',  ( -7.234628195640289583, 197.7700961906613770, -27.00000000000001421 ) ) ;
#5728=VERTEX_POINT ( 'NONE', #26767 ) ;
#5735=LINE ( 'NONE', #8965, #3110 ) ;
#5736=FACE_OUTER_BOUND ( 'NONE', #16157, .T. ) ;
#5737=CARTESIAN_POINT ( 'NONE',  ( 15.24356964375000167, 244.9468750006145399, 3.323476615752272600 ) ) ;
#5739=CARTESIAN_POINT ( 'NONE',  ( 18.12178482187500350, 241.8343750006145285, 4.985214923628407568 ) ) ;
#5740=ORIENTED_EDGE ( 'NONE', *, *, #30304, .T. ) ;
#5743=CARTESIAN_POINT ( 'NONE',  ( 23.99999999999999645, 246.3062500012290457, -5.196152422706631135 ) ) ;
#5744=VERTEX_POINT ( 'NONE', #20535 ) ;
#5755=ORIENTED_EDGE ( 'NONE', *, *, #776, .F. ) ;
#5759=CARTESIAN_POINT ( 'NONE',  ( 15.24356964374999990, 247.4593750006145285, -3.323476615752268604 ) ) ;
#5762=CARTESIAN_POINT ( 'NONE',  ( 14.04484906357430773, 216.9551509364345350, -0.1802446458350883129 ) ) ;
#5779=AXIS2_PLACEMENT_3D ( 'NONE', #3845, #13319, #24327 ) ;
#5786=CARTESIAN_POINT ( 'NONE',  ( 18.00000000000000000, 249.0250000000000057, -5.196152422706630247 ) ) ;
#5788=CARTESIAN_POINT ( 'NONE',  ( -1.926257025242585782E-15, 199.7468750006145513, -31.45816453501075927 ) ) ;
#5791=CARTESIAN_POINT ( 'NONE',  ( 20.99999999999999645, 248.1718750006145342, 6.646953231504538984 ) ) ;
#5798=CARTESIAN_POINT ( 'NONE',  ( 23.99999999999999645, 241.3000000000000114, -5.196152422706631135 ) ) ;
#5804=CARTESIAN_POINT ( 'NONE',  ( 5.727106289114498080E-15, 195.7250000012290343, 31.17691453623979214 ) ) ;
#5807=PRODUCT_DEFINITION_CONTEXT ( 'detailed design', #32784, 'design' ) ;
#5810=CIRCLE ( 'NONE', #13102, 6.000000000000005329 ) ;
#5811=CARTESIAN_POINT ( 'NONE',  ( 21.00000000000000000, 241.1968750006145399, -6.646953231504538984 ) ) ;
#5819=CARTESIAN_POINT ( 'NONE',  ( 26.61936306680777875, 195.0000000000000000, 5.364276260378865402 ) ) ;
#5820=CARTESIAN_POINT ( 'NONE',  ( -13.62178482187500528, 196.6343750006145399, -23.59362340125807123 ) ) ;
#5842=CARTESIAN_POINT ( 'NONE',  ( 13.62178482187501416, 196.4093750006145456, 23.59362340125806767 ) ) ;
#5846=CARTESIAN_POINT ( 'NONE',  ( 26.99999999999999645, 248.9125000000000227, -3.464101615137755275 ) ) ;
#5847=CARTESIAN_POINT ( 'NONE',  ( 5.778771075727756162E-15, 199.4656250006145797, 31.45816453501076637 ) ) ;
#5850=ORIENTED_EDGE ( 'NONE', *, *, #27087, .F. ) ;
#5851=ORIENTED_EDGE ( 'NONE', *, *, #11736, .T. ) ;
#5852=CARTESIAN_POINT ( 'NONE',  ( 27.24356964374999635, 198.7156250006145513, -15.72908226750539029 ) ) ;
#5853=CARTESIAN_POINT ( 'NONE',  ( 26.75643035624999655, 241.8343750006145001, 3.323476615752267715 ) ) ;
#5857=CARTESIAN_POINT ( 'NONE',  ( 26.75643035624999655, 246.8968750006145285, 3.323476615752267715 ) ) ;
#5861=CARTESIAN_POINT ( 'NONE',  ( 20.99999999999999645, 242.4343750006145228, -6.646953231504538984 ) ) ;
#5863=CARTESIAN_POINT ( 'NONE',  ( 22.60769515458672529, 246.7736538117967200, -6.000000000000004441 ) ) ;
#5867=CARTESIAN_POINT ( 'NONE',  ( 19.95811700914455500, 239.9653672772770392, -5.908847589363869446 ) ) ;
#5868=CARTESIAN_POINT ( 'NONE',  ( -27.00000000000000355, 198.7625000012290286, 0.000000000000000000 ) ) ;
#5876=CARTESIAN_POINT ( 'NONE',  ( 26.75643035624999655, 242.3218750006145399, -7.049594010296217766E-16 ) ) ;
#5883=CARTESIAN_POINT ( 'NONE',  ( 27.24356964374999635, 196.0718750006145683, -15.72908226750539029 ) ) ;
#5884=CARTESIAN_POINT ( 'NONE',  ( 24.00000000000000000, 246.1000000000000227, 5.196152422706629359 ) ) ;
#5892=CARTESIAN_POINT ( 'NONE',  ( 21.00000000000000000, 248.5093750006144830, 6.646953231504538984 ) ) ;
#5897=ORIENTED_EDGE ( 'NONE', *, *, #34903, .T. ) ;
#5899=CARTESIAN_POINT ( 'NONE',  ( 20.99999999999997513, 245.8937500012290798, -5.999999999999999112 ) ) ;
#5902=CARTESIAN_POINT ( 'NONE',  ( 15.00000000000000178, 245.5937500012290400, 3.464101615137757051 ) ) ;
#5904=CARTESIAN_POINT ( 'NONE',  ( -26.80567346611835333, 195.0000000000000853, 4.049898097028912680 ) ) ;
#5908=VERTEX_POINT ( 'NONE', #30570 ) ;
#5910=CARTESIAN_POINT ( 'NONE',  ( 4.999999999999997335, 216.0000000000000000, 7.347880794884120722E-16 ) ) ;
#5924=CARTESIAN_POINT ( 'NONE',  ( 26.75643035624999655, 245.9968750006145513, 3.323476615752267715 ) ) ;
#5926=CARTESIAN_POINT ( 'NONE',  ( 15.24356964374999990, 239.9218750006145626, -3.323476615752268604 ) ) ;
#5928=ORIENTED_EDGE ( 'NONE', *, *, #6629, .T. ) ;
#5930=CARTESIAN_POINT ( 'NONE',  ( 4.999999999999997335, 216.0000000000000000, 7.347880794884120722E-16 ) ) ;
#5931=CARTESIAN_POINT ( 'NONE',  ( 21.00000000000000000, 247.0187500012290513, 6.928203230275506996 ) ) ;
#5941=ORIENTED_EDGE ( 'NONE', *, *, #9197, .F. ) ;
#5945=CARTESIAN_POINT ( 'NONE',  ( 23.87821517812499650, 247.3468750006144887, -4.985214923628404904 ) ) ;
#5970=CARTESIAN_POINT ( 'NONE',  ( 20.99999999999999645, 210.0000000000000284, 0.000000000000000000 ) ) ;
#5972=CARTESIAN_POINT ( 'NONE',  ( 26.99999999999999645, 241.2812500012290400, -7.347880794884117764E-16 ) ) ;
#5974=CARTESIAN_POINT ( 'NONE',  ( -27.00000000000000355, 195.5000000000000000, 0.000000000000000000 ) ) ;
#5977=CARTESIAN_POINT ( 'NONE',  ( 20.99999999999999645, 246.8218750006145399, 6.646953231504538984 ) ) ;
#5985=CARTESIAN_POINT ( 'NONE',  ( 21.00000000000000000, 240.4375000000000000, -6.928203230275506996 ) ) ;
#5992=DIRECTION ( 'NONE',  ( -0.000000000000000000, 1.000000000000000000, -0.000000000000000000 ) ) ;
#5993=CARTESIAN_POINT ( 'NONE',  ( 1.120210788295102201E-13, 196.4000000012290741, -27.00000000000000711 ) ) ;
#5997=EDGE_CURVE ( 'NONE', #12534, #11333, #16163, .T. ) ;
#5998=CARTESIAN_POINT ( 'NONE',  ( 21.00000000000000000, 240.7468750006145228, -6.646953231504538984 ) ) ;
#6005=CARTESIAN_POINT ( 'NONE',  ( 0.000000000000000000, 210.0000000000000284, 0.000000000000000000 ) ) ;
#6006=CARTESIAN_POINT ( 'NONE',  ( -20.86978604919638869, 194.8588513911398081, -17.51182792271053046 ) ) ;
#6008=VERTEX_POINT ( 'NONE', #18829 ) ;
#6017=CARTESIAN_POINT ( 'NONE',  ( 15.00000000000000178, 249.5875000000000341, 3.464101615137757051 ) ) ;
#6021=CARTESIAN_POINT ( 'NONE',  ( -27.00000000000000355, 195.0266196731382706, -9.719019365307174141 ) ) ;
#6025=CARTESIAN_POINT ( 'NONE',  ( -13.62178482187500528, 196.1843750006145228, -23.59362340125807123 ) ) ;
#6029=CARTESIAN_POINT ( 'NONE',  ( 18.00000000000000000, 248.1250000000000000, -5.196152422706630247 ) ) ;
#6030=CARTESIAN_POINT ( 'NONE',  ( -13.62178482187500528, 199.2781250006145228, -23.59362340125807123 ) ) ;
#6033=VERTEX_POINT ( 'NONE', #1553 ) ;
#6035=CARTESIAN_POINT ( 'NONE',  ( 27.24356964374999635, 197.3656250006145285, -15.72908226750539029 ) ) ;
#6036=CARTESIAN_POINT ( 'NONE',  ( 23.87821517812500005, 242.2468750006145228, 4.985214923628404016 ) ) ;
#6039=CARTESIAN_POINT ( 'NONE',  ( 26.75643035624999655, 247.4218750006145058, -3.323476615752271712 ) ) ;
#6044=CARTESIAN_POINT ( 'NONE',  ( 26.75643035624999655, 242.3593750006145342, -3.323476615752271268 ) ) ;
#6054=DIRECTION ( 'NONE',  ( -0.000000000000000000, 1.000000000000000000, -0.000000000000000000 ) ) ;
#6057=CARTESIAN_POINT ( 'NONE',  ( 19.39230484541326405, 247.8986538117967200, 5.999999999999995559 ) ) ;
#6059=CARTESIAN_POINT ( 'NONE',  ( 18.12178482187499640, 242.4718750006145171, -4.985214923628404904 ) ) ;
#6064=DIRECTION ( 'NONE',  ( -0.000000000000000000, -1.000000000000000000, -0.000000000000000000 ) ) ;
#6065=FACE_OUTER_BOUND ( 'NONE', #35895, .T. ) ;
#6068=DIRECTION ( 'NONE',  ( -1.000000000000000000, 0.000000000000000000, 0.000000000000000000 ) ) ;
#6073=CARTESIAN_POINT ( 'NONE',  ( 26.75643035624999655, 248.6218750006145228, -7.049594010296217766E-16 ) ) ;
#6080=ORIENTED_EDGE ( 'NONE', *, *, #2517, .T. ) ;
#6087=CARTESIAN_POINT ( 'NONE',  ( 15.24356964375000167, 249.3343750006145001, 3.323476615752272600 ) ) ;
#6091=EDGE_CURVE ( 'NONE', #25480, #21774, #23611, .T. ) ;
#6093=ORIENTED_EDGE ( 'NONE', *, *, #10076, .F. ) ;
#6103=CARTESIAN_POINT ( 'NONE',  ( 18.00000000000000000, 242.2749999999999773, -5.196152422706630247 ) ) ;
#6108=DIRECTION ( 'NONE',  ( -0.000000000000000000, -1.000000000000000000, -0.000000000000000000 ) ) ;
#6109=EDGE_CURVE ( 'NONE', #14431, #19996, #15875, .T. ) ;
#6111=CARTESIAN_POINT ( 'NONE',  ( 26.75643035624999655, 246.0718750006145115, -3.323476615752271712 ) ) ;
#6113=CARTESIAN_POINT ( 'NONE',  ( 18.12178482187499640, 239.8843750006145115, -4.985214923628404904 ) ) ;
#6116=ORIENTED_EDGE ( 'NONE', *, *, #34481, .F. ) ;
#6118=ADVANCED_FACE ( 'NONE', ( #19762 ), #25791, .F. ) ;
#6119=CARTESIAN_POINT ( 'NONE',  ( 21.00000000000000000, 246.7937500012290570, -6.928203230275506996 ) ) ;
#6131=CARTESIAN_POINT ( 'NONE',  ( 15.24356964374999990, 247.4968750006145228, 0.000000000000000000 ) ) ;
#6134=CARTESIAN_POINT ( 'NONE',  ( 15.90209636607630195, 223.5944096904683818, -3.170162721593450694 ) ) ;
#6138=AXIS2_PLACEMENT_3D ( 'NONE', #2891, #23188, #6309 ) ;
#6164=CARTESIAN_POINT ( 'NONE',  ( -27.00000000000000355, 195.0263594417697846, -9.827195513778322677 ) ) ;
#6165=CARTESIAN_POINT ( 'NONE',  ( 21.00000000000000000, 240.2125000000000057, 5.999999999999998224 ) ) ;
#6167=CARTESIAN_POINT ( 'NONE',  ( 26.75643035624999655, 246.4468750006144830, 3.323476615752267271 ) ) ;
#6171=CARTESIAN_POINT ( 'NONE',  ( 15.24356964374999990, 249.7468750006145228, 0.000000000000000000 ) ) ;
#6176=CARTESIAN_POINT ( 'NONE',  ( 18.00000000000000000, 240.0249999999999773, -5.196152422706630247 ) ) ;
#6188=CARTESIAN_POINT ( 'NONE',  ( 23.87821517812499650, 241.6093750006145342, -4.985214923628404904 ) ) ;
#6197=CARTESIAN_POINT ( 'NONE',  ( 13.62178482187499640, 195.6593750006145456, -23.59362340125807123 ) ) ;
#6201=ORIENTED_EDGE ( 'NONE', *, *, #4531, .F. ) ;
#6203=DIRECTION ( 'NONE',  ( 0.000000000000000000, 0.000000000000000000, -1.000000000000000000 ) ) ;
#6211=CARTESIAN_POINT ( 'NONE',  ( 18.00000000000000000, 249.4749999999999943, -5.196152422706630247 ) ) ;
#6215=CARTESIAN_POINT ( 'NONE',  ( -13.49999999999998401, 195.2375000012290229, 23.38268590217985476 ) ) ;
#6219=LINE ( 'NONE', #29907, #13849 ) ;
#6223=CARTESIAN_POINT ( 'NONE',  ( 15.00000000000000178, 248.6875000000000284, 3.464101615137757051 ) ) ;
#6224=CARTESIAN_POINT ( 'NONE',  ( 27.24356964375000345, 195.9781250006145399, -3.336375036156643733E-15 ) ) ;
#6227=ORIENTED_EDGE ( 'NONE', *, *, #3340, .F. ) ;
#6229=CARTESIAN_POINT ( 'NONE',  ( 13.62178482187501416, 195.4531250006145342, 23.59362340125806767 ) ) ;
#6230=CARTESIAN_POINT ( 'NONE',  ( 15.24356964374999990, 242.0593750006145513, -3.323476615752268604 ) ) ;
#6234=CARTESIAN_POINT ( 'NONE',  ( 15.24356964374999990, 247.1593750006145171, 0.000000000000000000 ) ) ;
#6241=CARTESIAN_POINT ( 'NONE',  ( 18.12178482187499640, 241.1218750006145228, -4.985214923628404904 ) ) ;
#6247=EDGE_CURVE ( 'NONE', #26373, #1047, #32351, .T. ) ;
#6250=CARTESIAN_POINT ( 'NONE',  ( 15.00000000000000000, 241.0187500012290229, -3.464101615137752610 ) ) ;
#6255=CARTESIAN_POINT ( 'NONE',  ( 20.99999999999995381, 244.3187500012290627, 5.999999999999998224 ) ) ;
#6260=CARTESIAN_POINT ( 'NONE',  ( 15.24356964375000167, 241.6843750006144944, 3.323476615752272600 ) ) ;
#6271=ORIENTED_EDGE ( 'NONE', *, *, #889, .F. ) ;
#6272=CARTESIAN_POINT ( 'NONE',  ( 18.00000000000000000, 240.0812500012290513, -5.196152422706630247 ) ) ;
#6284=CARTESIAN_POINT ( 'NONE',  ( 23.87821517812499650, 249.1468750006145285, -4.985214923628404904 ) ) ;
#6296=VECTOR ( 'NONE', #8068, 1000.000000000000000 ) ;
#6301=VERTEX_POINT ( 'NONE', #5506 ) ;
#6309=DIRECTION ( 'NONE',  ( 0.000000000000000000, 0.000000000000000000, 1.000000000000000000 ) ) ;
#6310=CARTESIAN_POINT ( 'NONE',  ( 18.12178482187500350, 244.5343750006145456, 4.985214923628407568 ) ) ;
#6315=CARTESIAN_POINT ( 'NONE',  ( 18.00000000000000355, 246.5312500012290400, 5.196152422706632912 ) ) ;
#6323=VERTEX_POINT ( 'NONE', #29186 ) ;
#6324=ADVANCED_FACE ( 'NONE', ( #3228 ), #6826, .T. ) ;
#6328=CARTESIAN_POINT ( 'NONE',  ( 21.00000000000000000, 246.9343750006145228, -6.646953231504538984 ) ) ;
#6331=CARTESIAN_POINT ( 'NONE',  ( 10.42677199038734592, 213.9649605036083528, -4.520320870630215815 ) ) ;
#6352=AXIS2_PLACEMENT_3D ( 'NONE', #36755, #36564, #10981 ) ;
#6353=CARTESIAN_POINT ( 'NONE',  ( 20.99999999999999645, 185.0294372515228645, -5.999999999999999112 ) ) ;
#6358=CARTESIAN_POINT ( 'NONE',  ( 20.99999999999999645, 246.1468750006145285, -6.646953231504538984 ) ) ;
#6361=CARTESIAN_POINT ( 'NONE',  ( -14.50000000000000000, 210.0000000000000000, 0.000000000000000000 ) ) ;
#6365=CARTESIAN_POINT ( 'NONE',  ( 26.99999999999999645, 240.3625000000000114, -3.464101615137755275 ) ) ;
#6368=VERTEX_POINT ( 'NONE', #6456 ) ;
#6371=CARTESIAN_POINT ( 'NONE',  ( 22.60769515458672885, 246.5325961894323541, 5.999999999999997335 ) ) ;
#6375=CARTESIAN_POINT ( 'NONE',  ( 21.00000000000000000, 249.4375000000000568, -5.999999999999998224 ) ) ;
#6376=CARTESIAN_POINT ( 'NONE',  ( 15.24356964374999990, 240.3718750006145228, -3.323476615752268604 ) ) ;
#6378=CARTESIAN_POINT ( 'NONE',  ( -5.530181890562601232, 223.3271220116375275, 2.500000000000000000 ) ) ;
#6383=AXIS2_PLACEMENT_3D ( 'NONE', #15313, #26866, #24035 ) ;
#6386=CARTESIAN_POINT ( 'NONE',  ( -27.24356964374999990, 196.2218750006145456, -15.72908226750537786 ) ) ;
#6391=( BOUNDED_CURVE ( )  B_SPLINE_CURVE ( 2, ( #34672, #5863, #28606, #22945, #176, #9091, #11373, #8532, #11743 ),
 .UNSPECIFIED., .F., .F. ) 
 B_SPLINE_CURVE_WITH_KNOTS ( ( 3, 2, 2, 2, 3 ),
 ( 0.2717391304347825942, 0.2753623188405797118, 0.2826086956521738913, 0.2898550724637681264, 0.2934782608695652439 ),
 .UNSPECIFIED. ) 
 CURVE ( )  GEOMETRIC_REPRESENTATION_ITEM ( )  RATIONAL_B_SPLINE_CURVE ( ( 0.9330127018922191873, 0.9330127018922187432, 1.000000000000000000, 0.8660254037844387076, 1.000000000000000000, 0.8660254037844387076, 1.000000000000000000, 0.9330127018922188542, 0.9330127018922194093 ) ) 
 REPRESENTATION_ITEM ( '' )  );
#6393=CARTESIAN_POINT ( 'NONE',  ( -4.526655657482483441, 226.9744801578922022, -2.499999999999999556 ) ) ;
#6394=CARTESIAN_POINT ( 'NONE',  ( 1.069080835302379631E-14, 198.7624999999999886, 27.00000000000000000 ) ) ;
#6404=DIRECTION ( 'NONE',  ( -1.000000000000000000, -6.123233995736766036E-17, 0.000000000000000000 ) ) ;
#6408=FACE_OUTER_BOUND ( 'NONE', #12127, .T. ) ;
#6412=CARTESIAN_POINT ( 'NONE',  ( 21.00000000000000000, 249.4375000000000000, -6.928203230275506996 ) ) ;
#6413=CARTESIAN_POINT ( 'NONE',  ( -13.62178482187500528, 197.0281250006145228, -23.59362340125807123 ) ) ;
#6419=CARTESIAN_POINT ( 'NONE',  ( -27.24356964374999990, 195.2656250006145342, -15.72908226750537786 ) ) ;
#6420=CARTESIAN_POINT ( 'NONE',  ( 20.99999999999999289, 248.8187500012290911, 5.999999999999999112 ) ) ;
#6421=ADVANCED_FACE ( 'NONE', ( #18028 ), #11949, .F. ) ;
#6424=CARTESIAN_POINT ( 'NONE',  ( 26.75643035624999655, 248.7718750006145569, -3.323476615752271712 ) ) ;
#6430=CARTESIAN_POINT ( 'NONE',  ( 26.75643035624999655, 242.7343750006145058, 3.323476615752267271 ) ) ;
#6432=CARTESIAN_POINT ( 'NONE',  ( 20.99999999999999645, 249.6625000000000512, 5.999999999999998224 ) ) ;
#6435=VECTOR ( 'NONE', #22137, 1000.000000000000000 ) ;
#6443=CARTESIAN_POINT ( 'NONE',  ( 10.49999999999999645, 244.5000000000000000, 2.500000000000000000 ) ) ;
#6448=CARTESIAN_POINT ( 'NONE',  ( 15.24356964374999990, 242.9968750006145228, 0.000000000000000000 ) ) ;
#6449=ORIENTED_EDGE ( 'NONE', *, *, #8485, .F. ) ;
#6454=CARTESIAN_POINT ( 'NONE',  ( 5.778771075727756162E-15, 199.0718750006145399, 31.45816453501076637 ) ) ;
#6455=ADVANCED_FACE ( 'NONE', ( #17843 ), #15175, .F. ) ;
#6456=CARTESIAN_POINT ( 'NONE',  ( 15.24356964374999990, 249.7468750006145228, 0.000000000000000000 ) ) ;
#6464=CARTESIAN_POINT ( 'NONE',  ( 26.75643035624999655, 247.6843750006145513, 3.323476615752267715 ) ) ;
#6477=CARTESIAN_POINT ( 'NONE',  ( 15.24356964374999990, 248.3593750006145342, -3.323476615752268604 ) ) ;
#6484=CARTESIAN_POINT ( 'NONE',  ( -27.87471972953271049, 209.7345472881551984, 8.000000000000001776 ) ) ;
#6500=CARTESIAN_POINT ( 'NONE',  ( 21.00000000000001066, 247.0187500012290513, 5.999999999999998224 ) ) ;
#6502=DIRECTION ( 'NONE',  ( -4.130293990420971855E-17, 1.000000000000000000, 0.000000000000000000 ) ) ;
#6504=CARTESIAN_POINT ( 'NONE',  ( 26.99999999999999645, 247.1312500012290343, -7.347880794884117764E-16 ) ) ;
#6507=CARTESIAN_POINT ( 'NONE',  ( 20.99999999999999645, 185.0294372515228645, 5.999999999999999112 ) ) ;
#6516=CARTESIAN_POINT ( 'NONE',  ( 15.24356964375000167, 246.1843750006145513, 3.323476615752272600 ) ) ;
#6535=CARTESIAN_POINT ( 'NONE',  ( 20.99999999999998579, 248.1437500012290229, -5.999999999999997335 ) ) ;
#6536=VECTOR ( 'NONE', #3458, 1000.000000000000000 ) ;
#6540=LINE ( 'NONE', #6353, #14037 ) ;
#6542=CARTESIAN_POINT ( 'NONE',  ( 13.49999999999999645, 195.8000000000000114, -23.38268590217984766 ) ) ;
#6544=FACE_OUTER_BOUND ( 'NONE', #26441, .T. ) ;
#6546=CARTESIAN_POINT ( 'NONE',  ( 26.75643035624999655, 246.8968750006145285, 3.323476615752267271 ) ) ;
#6549=CARTESIAN_POINT ( 'NONE',  ( 18.00000000000000000, 245.0312500012290400, -5.196152422706630247 ) ) ;
#6553=CARTESIAN_POINT ( 'NONE',  ( 26.99999999999999645, 242.1250000000000000, -7.347880794884117764E-16 ) ) ;
#6557=ORIENTED_EDGE ( 'NONE', *, *, #34278, .F. ) ;
#6560=CARTESIAN_POINT ( 'NONE',  ( 20.99999999999998579, 248.3124999999999716, 5.999999999999998224 ) ) ;
#6565=CARTESIAN_POINT ( 'NONE',  ( 21.00000000000000000, 240.9718750006145456, 6.646953231504538984 ) ) ;
#6568=CARTESIAN_POINT ( 'NONE',  ( 18.00000000000000355, 245.5749999999999886, 5.196152422706632912 ) ) ;
#6573=CARTESIAN_POINT ( 'NONE',  ( 19.39230484541326049, 240.9075961894323541, -5.999999999999997335 ) ) ;
#6574=CARTESIAN_POINT ( 'NONE',  ( 5.778771075727756162E-15, 199.4656250006145797, 31.45816453501075927 ) ) ;
#6579=CARTESIAN_POINT ( 'NONE',  ( 20.99999999999999645, 210.0000000000000284, 0.000000000000000000 ) ) ;
#6589=ADVANCED_FACE ( 'NONE', ( #6065 ), #14985, .F. ) ;
#6593=VERTEX_POINT ( 'NONE', #26535 ) ;
#6596=CARTESIAN_POINT ( 'NONE',  ( 20.99999999999999645, 185.0294372515228645, 0.000000000000000000 ) ) ;
#6601=CARTESIAN_POINT ( 'NONE',  ( 21.00000000000000000, 248.5374999999999943, -6.928203230275506996 ) ) ;
#6602=CARTESIAN_POINT ( 'NONE',  ( -1.926257025242585782E-15, 196.5406250006145399, -31.45816453501076637 ) ) ;
#6606=CARTESIAN_POINT ( 'NONE',  ( 27.24356964374999635, 196.9156250006145399, -15.72908226750539029 ) ) ;
#6607=CARTESIAN_POINT ( 'NONE',  ( 26.75643035624999655, 240.0343750006145740, 3.323476615752267715 ) ) ;
#6611=CARTESIAN_POINT ( 'NONE',  ( 26.75643035624999655, 247.3843750006145399, -7.049594010296217766E-16 ) ) ;
#6618=CARTESIAN_POINT ( 'NONE',  ( 27.24356964375000345, 199.6343750006145399, -3.336375036156643733E-15 ) ) ;
#6629=EDGE_CURVE ( 'NONE', #30804, #6033, #7015, .T. ) ;
#6632=DIRECTION ( 'NONE',  ( 0.000000000000000000, 0.000000000000000000, 1.000000000000000000 ) ) ;
#6633=( BOUNDED_CURVE ( )  B_SPLINE_CURVE ( 2, ( #27773, #1803, #13370, #13936, #25484, #8060, #37404, #20181, #28880 ),
 .UNSPECIFIED., .F., .F. ) 
 B_SPLINE_CURVE_WITH_KNOTS ( ( 3, 2, 2, 2, 3 ),
 ( 0.7282608695652174058, 0.7318840579710145233, 0.7391304347826086474, 0.7463768115942028825, 0.7500000000000000000 ),
 .UNSPECIFIED. ) 
 CURVE ( )  GEOMETRIC_REPRESENTATION_ITEM ( )  RATIONAL_B_SPLINE_CURVE ( ( 0.9330127018922194093, 0.9330127018922194093, 1.000000000000000000, 0.8660254037844387076, 1.000000000000000000, 0.8660254037844387076, 1.000000000000000000, 0.9330127018922194093, 0.9330127018922194093 ) ) 
 REPRESENTATION_ITEM ( '' )  );
#6636=CARTESIAN_POINT ( 'NONE',  ( 26.75643035624999655, 241.9093750006145171, -3.323476615752271712 ) ) ;
#6640=CARTESIAN_POINT ( 'NONE',  ( 24.00000000000000000, 242.5000000000000000, 5.196152422706629359 ) ) ;
#6643=LINE ( 'NONE', #9303, #32432 ) ;
#6649=CARTESIAN_POINT ( 'NONE',  ( 21.00000000000000000, 246.0343750006144887, -6.646953231504538984 ) ) ;
#6657=VERTEX_POINT ( 'NONE', #19309 ) ;
#6659=AXIS2_PLACEMENT_3D ( 'NONE', #28128, #33129, #2712 ) ;
#6662=CARTESIAN_POINT ( 'NONE',  ( 20.99999999999999645, 248.9593750006145285, 6.646953231504538984 ) ) ;
#6668=CARTESIAN_POINT ( 'NONE',  ( -27.94841835328498902, 207.9074690653111475, 7.739347195566303128 ) ) ;
#6672=( BOUNDED_CURVE ( )  B_SPLINE_CURVE ( 2, ( #5420, #2951, #2584, #20217, #23059, #23425, #29095, #20590, #26443 ),
 .UNSPECIFIED., .F., .F. ) 
 B_SPLINE_CURVE_WITH_KNOTS ( ( 3, 2, 2, 2, 3 ),
 ( 0.6195652173913043237, 0.6231884057971014412, 0.6304347826086956763, 0.6376811594202898004, 0.6413043478260869179 ),
 .UNSPECIFIED. ) 
 CURVE ( )  GEOMETRIC_REPRESENTATION_ITEM ( )  RATIONAL_B_SPLINE_CURVE ( ( 0.9330127018922194093, 0.9330127018922194093, 1.000000000000000000, 0.8660254037844387076, 1.000000000000000000, 0.8660254037844387076, 1.000000000000000000, 0.9330127018922194093, 0.9330127018922194093 ) ) 
 REPRESENTATION_ITEM ( '' )  );
#6674=EDGE_CURVE ( 'NONE', #3075, #31515, #36643, .T. ) ;
#6675=CARTESIAN_POINT ( 'NONE',  ( 19.39230484541326760, 249.2486538117967427, 5.999999999999999112 ) ) ;
#6679=EDGE_CURVE ( 'NONE', #2746, #7301, #20797, .T. ) ;
#6684=AXIS2_PLACEMENT_3D ( 'NONE', #4897, #13820, #8134 ) ;
#6691=CARTESIAN_POINT ( 'NONE',  ( 0.000000000000000000, 210.0000000000000284, 0.000000000000000000 ) ) ;
#6693=CARTESIAN_POINT ( 'NONE',  ( 15.00000000000000000, 245.1062500012290286, 0.000000000000000000 ) ) ;
#6696=CARTESIAN_POINT ( 'NONE',  ( 18.00000000000000000, 242.7249999999999943, -5.196152422706630247 ) ) ;
#6703=CARTESIAN_POINT ( 'NONE',  ( 26.75643035624999655, 243.6718750006145058, -7.049594010296217766E-16 ) ) ;
#6724=VECTOR ( 'NONE', #35653, 1000.000000000000000 ) ;
#6727=LINE ( 'NONE', #12980, #1112 ) ;
#6734=CARTESIAN_POINT ( 'NONE',  ( 20.99999999999999645, 247.0468750006145058, -6.646953231504538984 ) ) ;
#6735=EDGE_LOOP ( 'NONE', ( #29915, #16615, #5200, #31531 ) ) ;
#6745=CARTESIAN_POINT ( 'NONE',  ( 0.000000000000000000, 195.0000000000000000, 0.000000000000000000 ) ) ;
#6746=CARTESIAN_POINT ( 'NONE',  ( -27.24356964375000345, 199.8312500006145171, 0.000000000000000000 ) ) ;
#6748=CARTESIAN_POINT ( 'NONE',  ( 26.99999999999999645, 243.0249999999999773, -7.347880794884117764E-16 ) ) ;
#6753=CARTESIAN_POINT ( 'NONE',  ( 19.95279056986857569, 210.3927035363166169, 5.999999999999996447 ) ) ;
#6755=FACE_OUTER_BOUND ( 'NONE', #29597, .T. ) ;
#6761=CARTESIAN_POINT ( 'NONE',  ( -27.24356964374999990, 197.9656250006145228, -15.72908226750537786 ) ) ;
#6764=ORIENTED_EDGE ( 'NONE', *, *, #35521, .T. ) ;
#6767=CARTESIAN_POINT ( 'NONE',  ( -26.99999999999999645, 197.7874999999999943, 15.58845726811991561 ) ) ;
#6778=CYLINDRICAL_SURFACE ( 'NONE', #14750, 5.999999999999999112 ) ;
#6781=CARTESIAN_POINT ( 'NONE',  ( 22.60769515458672174, 244.7888461906613600, 6.000000000000004441 ) ) ;
#6782=AXIS2_PLACEMENT_3D ( 'NONE', #30033, #1030, #35711 ) ;
#6784=CARTESIAN_POINT ( 'NONE',  ( -27.00000000000000355, 198.3125000012290400, 0.000000000000000000 ) ) ;
#6787=CARTESIAN_POINT ( 'NONE',  ( 26.99999999999999645, 245.3124999999999716, -3.464101615137755275 ) ) ;
#6788=CARTESIAN_POINT ( 'NONE',  ( 27.24356964375000345, 195.5281250006145228, -3.336375036156643733E-15 ) ) ;
#6791=EDGE_LOOP ( 'NONE', ( #14276, #11914, #34935, #8057 ) ) ;
#6793=CARTESIAN_POINT ( 'NONE',  ( 13.62178482187501416, 196.8031250006145285, 23.59362340125806767 ) ) ;
#6794=CARTESIAN_POINT ( 'NONE',  ( 15.24356964374999990, 240.7468750006144944, 0.000000000000000000 ) ) ;
#6798=CARTESIAN_POINT ( 'NONE',  ( 23.87821517812499650, 246.1093750006145342, -4.985214923628404904 ) ) ;
#6804=CARTESIAN_POINT ( 'NONE',  ( 15.24356964375000167, 239.8843750006145115, 3.323476615752272600 ) ) ;
#6810=LINE ( 'NONE', #7201, #35876 ) ;
#6818=EDGE_CURVE ( 'NONE', #10561, #6368, #14952, .T. ) ;
#6821=CARTESIAN_POINT ( 'NONE',  ( 15.24356964374999990, 239.8093750006145228, -3.323476615752268604 ) ) ;
#6825=CARTESIAN_POINT ( 'NONE',  ( -13.62178482187500528, 199.7843750006145456, -23.59362340125807123 ) ) ;
#6826=CYLINDRICAL_SURFACE ( 'NONE', #2745, 7.500000000000000000 ) ;
#6827=DIRECTION ( 'NONE',  ( -0.000000000000000000, 1.000000000000000000, -0.000000000000000000 ) ) ;
#6829=VECTOR ( 'NONE', #4272, 1000.000000000000000 ) ;
#6835=CARTESIAN_POINT ( 'NONE',  ( 15.24356964374999990, 246.1093750006145342, -3.323476615752268604 ) ) ;
#6841=AXIS2_PLACEMENT_3D ( 'NONE', #36089, #12604, #35901 ) ;
#6847=EDGE_CURVE ( 'NONE', #27888, #17896, #14521, .T. ) ;
#6849=VECTOR ( 'NONE', #13997, 1000.000000000000000 ) ;
#6852=CARTESIAN_POINT ( 'NONE',  ( 15.24356964374999990, 246.5593750006144944, -3.323476615752268604 ) ) ;
#6857=CARTESIAN_POINT ( 'NONE',  ( 15.00000000000000178, 245.9875000000000398, 3.464101615137757051 ) ) ;
#6861=CARTESIAN_POINT ( 'NONE',  ( 15.00000000000000178, 248.6875000000000000, 3.464101615137757051 ) ) ;
#6866=CARTESIAN_POINT ( 'NONE',  ( 19.39230484541324984, 246.5486538117966973, 5.999999999999991118 ) ) ;
#6877=CARTESIAN_POINT ( 'NONE',  ( 26.99999999999999645, 196.6625000000000227, -15.58845726811990495 ) ) ;
#6882=CYLINDRICAL_SURFACE ( 'NONE', #7660, 28.99999999999999645 ) ;
#6884=CARTESIAN_POINT ( 'NONE',  ( 18.00000000000000355, 242.9312500012290457, 5.196152422706632912 ) ) ;
#6894=CARTESIAN_POINT ( 'NONE',  ( 23.87821517812500005, 243.5968750006145171, 4.985214923628404016 ) ) ;
#6899=VECTOR ( 'NONE', #22643, 1000.000000000000000 ) ;
#6901=( BOUNDED_CURVE ( )  B_SPLINE_CURVE ( 2, ( #16334, #14044, #25228, #16150, #33577, #7802, #24855, #10822, #27882 ),
 .UNSPECIFIED., .F., .F. ) 
 B_SPLINE_CURVE_WITH_KNOTS ( ( 3, 2, 2, 2, 3 ),
 ( 0.5108695652173913526, 0.5144927536231883591, 0.5217391304347825942, 0.5289855072463768293, 0.5326086956521739468 ),
 .UNSPECIFIED. ) 
 CURVE ( )  GEOMETRIC_REPRESENTATION_ITEM ( )  RATIONAL_B_SPLINE_CURVE ( ( 0.9330127018922192983, 0.9330127018922202975, 1.000000000000000000, 0.8660254037844387076, 1.000000000000000000, 0.8660254037844387076, 1.000000000000000000, 0.9330127018922194093, 0.9330127018922194093 ) ) 
 REPRESENTATION_ITEM ( '' )  );
#6909=DIRECTION ( 'NONE',  ( 0.000000000000000000, 0.000000000000000000, 1.000000000000000000 ) ) ;
#6911=EDGE_CURVE ( 'NONE', #24301, #29694, #6672, .T. ) ;
#6918=ORIENTED_EDGE ( 'NONE', *, *, #9691, .T. ) ;
#6922=CARTESIAN_POINT ( 'NONE',  ( 0.000000000000000000, 210.0000000000000284, -27.00000000000000000 ) ) ;
#6926=CARTESIAN_POINT ( 'NONE',  ( 18.00000000000000355, 247.4312500012290457, 5.196152422706632912 ) ) ;
#6928=CARTESIAN_POINT ( 'NONE',  ( 26.75643035624999655, 244.6843750006145228, -7.049594010296217766E-16 ) ) ;
#6930=ORIENTED_EDGE ( 'NONE', *, *, #10076, .T. ) ;
#6940=CARTESIAN_POINT ( 'NONE',  ( -8.147263093523481103, 219.8189111151660029, 2.997147438070004721 ) ) ;
#6944=ORIENTED_EDGE ( 'NONE', *, *, #28448, .T. ) ;
#6954=CARTESIAN_POINT ( 'NONE',  ( 16.47967912936645263, 222.0541889883434976, 3.964960503605021280 ) ) ;
#6964=CARTESIAN_POINT ( 'NONE',  ( 5.778771075727756162E-15, 198.5656250006145171, 31.45816453501075927 ) ) ;
#6967=ORIENTED_EDGE ( 'NONE', *, *, #22705, .F. ) ;
#6981=CARTESIAN_POINT ( 'NONE',  ( -27.00000000000000355, 200.0000000000000000, 0.000000000000000000 ) ) ;
#6991=CARTESIAN_POINT ( 'NONE',  ( 15.00000000000000000, 245.4625000000000057, -3.464101615137752166 ) ) ;
#6992=CARTESIAN_POINT ( 'NONE',  ( -27.24356964375000345, 197.1031250006145399, 0.000000000000000000 ) ) ;
#6996=EDGE_LOOP ( 'NONE', ( #26128, #7212, #24838, #35940 ) ) ;
#6997=CARTESIAN_POINT ( 'NONE',  ( 13.62178482187501416, 196.3531250006145115, 23.59362340125806767 ) ) ;
#6998=CARTESIAN_POINT ( 'NONE',  ( 18.12178482187500350, 240.8218750006145399, 4.985214923628407568 ) ) ;
#7002=CARTESIAN_POINT ( 'NONE',  ( 18.12178482187500350, 244.5343750006145456, 4.985214923628407568 ) ) ;
#7004=CARTESIAN_POINT ( 'NONE',  ( 21.00000000000000000, 242.9687500012290684, 5.999999999999998224 ) ) ;
#7013=FACE_OUTER_BOUND ( 'NONE', #22463, .T. ) ;
#7015=CIRCLE ( 'NONE', #12443, 8.000000000000007105 ) ;
#7021=CARTESIAN_POINT ( 'NONE',  ( 1.069080835302379631E-14, 198.4250000012290229, 27.00000000000000000 ) ) ;
#7024=CARTESIAN_POINT ( 'NONE',  ( 11.62741699796950989, 213.5147186257614180, 5.999999999999998224 ) ) ;
#7025=CARTESIAN_POINT ( 'NONE',  ( 26.75643035624999655, 249.2218750006144887, -3.323476615752271712 ) ) ;
#7026=B_SPLINE_CURVE_WITH_KNOTS ( 'NONE', 3,
 ( #31147, #24706, #36258, #16744, #33614, #30594, #10860, #10301, #7280, #36818, #1769, #21872, #28291, #22433, #8023, #13520 ),
 .UNSPECIFIED., .F., .F.,
 ( 4, 2, 2, 2, 2, 2, 2, 4 ),
 ( 0.000000000000000000, 0.002989157573830781168, 0.004483736360746172836, 0.005978315147661564938, 0.008967472721492300569, 0.01046205150840768747, 0.01120934090186539826, 0.01195663029532311079 ),
 .UNSPECIFIED. ) ;
#7027=ORIENTED_EDGE ( 'NONE', *, *, #14956, .T. ) ;
#7030=CARTESIAN_POINT ( 'NONE',  ( 26.99999999999999645, 242.5750000000000171, -7.347880794884117764E-16 ) ) ;
#7032=CYLINDRICAL_SURFACE ( 'NONE', #29400, 5.999999999999999112 ) ;
#7033=CARTESIAN_POINT ( 'NONE',  ( 14.99999999999999289, 204.0000000000000000, 0.000000000000000000 ) ) ;
#7034=CARTESIAN_POINT ( 'NONE',  ( 18.12178482187500350, 243.6343750006145115, 4.985214923628407568 ) ) ;
#7040=CARTESIAN_POINT ( 'NONE',  ( 26.75643035624999655, 246.3343750006145285, 3.323476615752267715 ) ) ;
#7046=ORIENTED_EDGE ( 'NONE', *, *, #18000, .T. ) ;
#7053=CARTESIAN_POINT ( 'NONE',  ( 15.24356964374999990, 247.0093750006145115, -3.323476615752268604 ) ) ;
#7056=CARTESIAN_POINT ( 'NONE',  ( 15.00000000000000000, 245.9499999999999886, 0.000000000000000000 ) ) ;
#7058=VERTEX_POINT ( 'NONE', #20407 ) ;
#7064=DIRECTION ( 'NONE',  ( 0.000000000000000000, 1.000000000000000000, 0.000000000000000000 ) ) ;
#7068=UNCERTAINTY_MEASURE_WITH_UNIT (LENGTH_MEASURE( 1.000000000000000082E-05 ), #1195, 'distance_accuracy_value', 'NONE');
#7069=EDGE_LOOP ( 'NONE', ( #11306, #3431, #23205, #19972 ) ) ;
#7070=CARTESIAN_POINT ( 'NONE',  ( 27.00000000000000355, 197.6375000012290286, -3.306546357697854128E-15 ) ) ;
#7077=CARTESIAN_POINT ( 'NONE',  ( -1.909035429704832693E-15, 195.8375000000000057, -31.17691453623979214 ) ) ;
#7082=CARTESIAN_POINT ( 'NONE',  ( 18.00000000000000355, 243.8312500012290513, 5.196152422706632912 ) ) ;
#7089=CARTESIAN_POINT ( 'NONE',  ( 0.000000000000000000, 210.0000000000000284, 0.000000000000000000 ) ) ;
#7090=CARTESIAN_POINT ( 'NONE',  ( 18.12178482187500350, 243.9718750006145171, 4.985214923628407568 ) ) ;
#7094=( BOUNDED_CURVE ( )  B_SPLINE_CURVE ( 2, ( #24018, #35369, #1441, #4103, #878, #15106, #29502, #6573, #9421 ),
 .UNSPECIFIED., .F., .F. ) 
 B_SPLINE_CURVE_WITH_KNOTS ( ( 3, 2, 2, 2, 3 ),
 ( 0.8586956521739130821, 0.8623188405797101996, 0.8695652173913043237, 0.8768115942028985588, 0.8804347826086956763 ),
 .UNSPECIFIED. ) 
 CURVE ( )  GEOMETRIC_REPRESENTATION_ITEM ( )  RATIONAL_B_SPLINE_CURVE ( ( 0.9330127018922194093, 0.9330127018922194093, 1.000000000000000000, 0.8660254037844387076, 1.000000000000000000, 0.8660254037844387076, 1.000000000000000000, 0.9330127018922194093, 0.9330127018922194093 ) ) 
 REPRESENTATION_ITEM ( '' )  );
#7104=CARTESIAN_POINT ( 'NONE',  ( 3.253724281355069334E-15, 199.8875000000000455, -27.00000000000000000 ) ) ;
#7117=CARTESIAN_POINT ( 'NONE',  ( 23.87821517812500005, 249.1093750006145342, 4.985214923628404016 ) ) ;
#7119=CARTESIAN_POINT ( 'NONE',  ( 15.24356964375000167, 244.9468750006144830, 3.323476615752272600 ) ) ;
#7121=CARTESIAN_POINT ( 'NONE',  ( 20.00041297495057080, 239.8598985277379256, -5.668978411116884608 ) ) ;
#7127=ORIENTED_EDGE ( 'NONE', *, *, #1948, .F. ) ;
#7130=VERTEX_POINT ( 'NONE', #31401 ) ;
#7131=CARTESIAN_POINT ( 'NONE',  ( -27.00000000000000355, 195.9125000000000796, -15.58845726811989429 ) ) ;
#7133=CARTESIAN_POINT ( 'NONE',  ( 20.99999999999999289, 249.2125000000000057, 5.999999999999999112 ) ) ;
#7134=( BOUNDED_CURVE ( )  B_SPLINE_CURVE ( 2, ( #2379, #13954, #34774, #14876, #32676, #26803, #20389, #14686, #3305 ),
 .UNSPECIFIED., .F., .F. ) 
 B_SPLINE_CURVE_WITH_KNOTS ( ( 3, 2, 2, 2, 3 ),
 ( 0.8804347826086956763, 0.8840579710144927938, 0.8913043478260869179, 0.8985507246376811530, 0.9021739130434782705 ),
 .UNSPECIFIED. ) 
 CURVE ( )  GEOMETRIC_REPRESENTATION_ITEM ( )  RATIONAL_B_SPLINE_CURVE ( ( 0.9330127018922194093, 0.9330127018922194093, 1.000000000000000000, 0.8660254037844387076, 1.000000000000000000, 0.8660254037844387076, 1.000000000000000000, 0.9330127018922194093, 0.9330127018922194093 ) ) 
 REPRESENTATION_ITEM ( '' )  );
#7141=CARTESIAN_POINT ( 'NONE',  ( 19.39230484541326760, 245.5924038105676743, 5.999999999999999112 ) ) ;
#7148=CARTESIAN_POINT ( 'NONE',  ( -13.62178482187500528, 197.4781250006145399, -23.59362340125807123 ) ) ;
#7152=ORIENTED_EDGE ( 'NONE', *, *, #35270, .F. ) ;
#7154=CARTESIAN_POINT ( 'NONE',  ( -29.00000000000002487, 210.0000000000000284, 8.000000000000000000 ) ) ;
#7170=ORIENTED_EDGE ( 'NONE', *, *, #30917, .F. ) ;
#7175=CARTESIAN_POINT ( 'NONE',  ( 18.00000000000000355, 245.5749999999999886, 5.196152422706632912 ) ) ;
#7183=ORIENTED_EDGE ( 'NONE', *, *, #2992, .T. ) ;
#7184=CARTESIAN_POINT ( 'NONE',  ( -13.50000000000000533, 198.6875000012290400, -23.38268590217984411 ) ) ;
#7187=( BOUNDED_CURVE ( )  B_SPLINE_CURVE ( 2, ( #37111, #11159, #8324, #22732, #10969 ),
 .UNSPECIFIED., .F., .F. ) 
 B_SPLINE_CURVE_WITH_KNOTS ( ( 3, 2, 3 ),
 ( 0.8541666666666667407, 0.8611111111111111605, 0.8636088982343050890 ),
 .UNSPECIFIED. ) 
 CURVE ( )  GEOMETRIC_REPRESENTATION_ITEM ( )  RATIONAL_B_SPLINE_CURVE ( ( 0.9330127018922192983, 0.9330127018922198534, 1.000000000000000000, 0.9759059184691117883, 0.9604780286076208817 ) ) 
 REPRESENTATION_ITEM ( '' )  );
#7189=CARTESIAN_POINT ( 'NONE',  ( 15.24356964375000167, 244.4968750006145228, 3.323476615752272600 ) ) ;
#7196=CARTESIAN_POINT ( 'NONE',  ( 19.00081547855239350, 239.7604221912915534, -5.492723509887032840 ) ) ;
#7200=( BOUNDED_CURVE ( )  B_SPLINE_CURVE ( 2, ( #27530, #19015, #22596, #22409, #19204 ),
 .UNSPECIFIED., .F., .F. ) 
 B_SPLINE_CURVE_WITH_KNOTS ( ( 3, 2, 3 ),
 ( 0.000000000000000000, 0.007246376811594202987, 0.01086956521739129711 ),
 .UNSPECIFIED. ) 
 CURVE ( )  GEOMETRIC_REPRESENTATION_ITEM ( )  RATIONAL_B_SPLINE_CURVE ( ( 1.000000000000000000, 0.8660254037844387076, 1.000000000000000000, 0.9330127018922194093, 0.9330127018922192983 ) ) 
 REPRESENTATION_ITEM ( '' )  );
#7201=CARTESIAN_POINT ( 'NONE',  ( 15.24356964374999990, 249.8031250006145285, 0.000000000000000000 ) ) ;
#7206=CARTESIAN_POINT ( 'NONE',  ( 3.253724281355069334E-15, 199.5500000012290513, -27.00000000000000000 ) ) ;
#7211=CARTESIAN_POINT ( 'NONE',  ( 15.24356964374999990, 249.4093750006145171, 0.000000000000000000 ) ) ;
#7212=ORIENTED_EDGE ( 'NONE', *, *, #27619, .T. ) ;
#7217=CARTESIAN_POINT ( 'NONE',  ( 18.91622474583366653, 239.6197971919061160, -5.725135026351895640 ) ) ;
#7218=CARTESIAN_POINT ( 'NONE',  ( 26.75643035624999655, 243.8218750006145399, -3.323476615752271712 ) ) ;
#7224=CARTESIAN_POINT ( 'NONE',  ( 26.75643035624999655, 246.8593750006145342, -3.323476615752271712 ) ) ;
#7236=CARTESIAN_POINT ( 'NONE',  ( 18.12178482187500350, 245.7718750006145001, 4.985214923628407568 ) ) ;
#7237=CARTESIAN_POINT ( 'NONE',  ( 27.00000000000001421, 196.5875000000000341, 15.58845726811988897 ) ) ;
#7246=CARTESIAN_POINT ( 'NONE',  ( 0.000000000000000000, 202.0000000000000000, -27.00000000000000000 ) ) ;
#7256=CARTESIAN_POINT ( 'NONE',  ( 5.778771075727756162E-15, 198.1718750006145342, 31.45816453501075927 ) ) ;
#7260=ORIENTED_EDGE ( 'NONE', *, *, #13066, .T. ) ;
#7261=CARTESIAN_POINT ( 'NONE',  ( 24.00000000000000000, 244.3562500012290286, 5.196152422706629359 ) ) ;
#7269=CARTESIAN_POINT ( 'NONE',  ( 26.75643035624999655, 245.0218750006145001, -7.049594010296217766E-16 ) ) ;
#7271=EDGE_CURVE ( 'NONE', #24534, #25338, #34015, .T. ) ;
#7280=CARTESIAN_POINT ( 'NONE',  ( -11.18923628784230573, 217.4947066899765389, -4.100298858792801759 ) ) ;
#7283=CYLINDRICAL_SURFACE ( 'NONE', #25014, 5.999999999999999112 ) ;
#7286=EDGE_CURVE ( 'NONE', #33968, #5728, #34834, .T. ) ;
#7293=CARTESIAN_POINT ( 'NONE',  ( 26.99999999999999645, 247.5250000000000057, -7.347880794884117764E-16 ) ) ;
#7295=ADVANCED_FACE ( 'NONE', ( #33077, #24176 ), #35341, .T. ) ;
#7297=DIRECTION ( 'NONE',  ( 0.000000000000000000, 1.000000000000000000, 0.000000000000000000 ) ) ;
#7299=CARTESIAN_POINT ( 'NONE',  ( 26.75643035624999655, 243.8218750006145399, -3.323476615752271268 ) ) ;
#7301=VERTEX_POINT ( 'NONE', #7121 ) ;
#7321=CARTESIAN_POINT ( 'NONE',  ( 13.90958069845249767, 212.6589072380734251, 5.392997762652351312 ) ) ;
#7326=ADVANCED_FACE ( 'NONE', ( #18692 ), #12422, .F. ) ;
#7332=CARTESIAN_POINT ( 'NONE',  ( 13.62178482187499640, 199.6531250006145228, -23.59362340125807123 ) ) ;
#7336=ORIENTED_EDGE ( 'NONE', *, *, #1487, .F. ) ;
#7351=FACE_OUTER_BOUND ( 'NONE', #26023, .T. ) ;
#7355=VERTEX_POINT ( 'NONE', #29850 ) ;
#7359=CARTESIAN_POINT ( 'NONE',  ( 21.00000000000000000, 246.2874999999999659, -6.928203230275506996 ) ) ;
#7365=ORIENTED_EDGE ( 'NONE', *, *, #4969, .F. ) ;
#7366=CARTESIAN_POINT ( 'NONE',  ( -26.99999999999998934, 198.8000000012290513, 15.58845726811991561 ) ) ;
#7367=CARTESIAN_POINT ( 'NONE',  ( 20.99999999999999289, 248.5937500012290400, -5.999999999999997335 ) ) ;
#7370=CARTESIAN_POINT ( 'NONE',  ( 18.12178482187499640, 244.8343750006145285, -4.985214923628404904 ) ) ;
#7372=DIRECTION ( 'NONE',  ( 0.000000000000000000, 0.000000000000000000, -1.000000000000000000 ) ) ;
#7377=CARTESIAN_POINT ( 'NONE',  ( 26.75643035624999655, 240.5218750006145001, -7.049594010296217766E-16 ) ) ;
#7390=CARTESIAN_POINT ( 'NONE',  ( 15.24356964375000167, 240.3343750006145001, 3.323476615752272600 ) ) ;
#7394=CARTESIAN_POINT ( 'NONE',  ( -13.62178482187500528, 197.5343750006145456, -23.59362340125807123 ) ) ;
#7398=CARTESIAN_POINT ( 'NONE',  ( 15.24356964375000167, 242.6968750006145399, 3.323476615752272600 ) ) ;
#7401=ORIENTED_EDGE ( 'NONE', *, *, #23703, .F. ) ;
#7402=ORIENTED_EDGE ( 'NONE', *, *, #33282, .T. ) ;
#7403=CIRCLE ( 'NONE', #29156, 27.00000000000000000 ) ;
#7404=CARTESIAN_POINT ( 'NONE',  ( 26.75643035624999655, 245.5093750006145115, -3.323476615752271712 ) ) ;
#7420=( BOUNDED_CURVE ( )  B_SPLINE_CURVE ( 2, ( #26297, #2807, #6215, #32549, #29331, #23100, #148, #8688, #23850 ),
 .UNSPECIFIED., .F., .F. ) 
 B_SPLINE_CURVE_WITH_KNOTS ( ( 3, 2, 2, 2, 3 ),
 ( 0.8125000000000000000, 0.8194444444444444198, 0.8333333333333333703, 0.8472222222222222099, 0.8541666666666667407 ),
 .UNSPECIFIED. ) 
 CURVE ( )  GEOMETRIC_REPRESENTATION_ITEM ( )  RATIONAL_B_SPLINE_CURVE ( ( 0.9330127018922194093, 0.9330127018922194093, 1.000000000000000000, 0.8660254037844387076, 1.000000000000000000, 0.8660254037844387076, 1.000000000000000000, 0.9330127018922187432, 0.9330127018922192983 ) ) 
 REPRESENTATION_ITEM ( '' )  );
#7422=CARTESIAN_POINT ( 'NONE',  ( 15.24356964375000167, 246.1843750006145513, 3.323476615752272600 ) ) ;
#7424=CARTESIAN_POINT ( 'NONE',  ( -1.045839947578415010E-13, 196.5125000000000455, 27.00000000000000355 ) ) ;
#7434=AXIS2_PLACEMENT_3D ( 'NONE', #27806, #30088, #15882 ) ;
#7441=CARTESIAN_POINT ( 'NONE',  ( 13.62178482187499640, 198.8093750006145513, -23.59362340125807123 ) ) ;
#7442=DIRECTION ( 'NONE',  ( -1.000000000000000000, 0.000000000000000000, 0.000000000000000000 ) ) ;
#7446=CARTESIAN_POINT ( 'NONE',  ( 15.00000000000000178, 241.9937500012290457, 3.464101615137757051 ) ) ;
#7468=CARTESIAN_POINT ( 'NONE',  ( 26.99999999999999645, 199.8125000000000000, -15.58845726811990495 ) ) ;
#7472=CARTESIAN_POINT ( 'NONE',  ( 20.99999999999999645, 192.3000000000000398, -8.000000000000000000 ) ) ;
#7477=CARTESIAN_POINT ( 'NONE',  ( 21.00000000000001066, 247.4124999999999943, 5.999999999999998224 ) ) ;
#7479=CARTESIAN_POINT ( 'NONE',  ( -7.234628195640302017, 195.5924038105676743, 27.00000000000000711 ) ) ;
#7481=CARTESIAN_POINT ( 'NONE',  ( 21.00000000000000000, 246.8218750006145399, 6.646953231504538984 ) ) ;
#7483=CARTESIAN_POINT ( 'NONE',  ( 15.24356964374999990, 244.0093750006145399, 0.000000000000000000 ) ) ;
#7485=ORIENTED_EDGE ( 'NONE', *, *, #24532, .T. ) ;
#7499=CARTESIAN_POINT ( 'NONE',  ( 20.99999999999997513, 247.1875000000000284, -5.999999999999999112 ) ) ;
#7507=CARTESIAN_POINT ( 'NONE',  ( 20.99999999999999645, 210.0000000000000000, 5.999999999999996447 ) ) ;
#7509=CARTESIAN_POINT ( 'NONE',  ( 13.49999999999999645, 197.1500000000000057, -23.38268590217984766 ) ) ;
#7517=CARTESIAN_POINT ( 'NONE',  ( -13.62178482187498396, 195.3781250006145171, 23.59362340125808188 ) ) ;
#7532=DIRECTION ( 'NONE',  ( -0.000000000000000000, -1.000000000000000000, -0.000000000000000000 ) ) ;
#7534=EDGE_CURVE ( 'NONE', #10561, #23659, #9331, .T. ) ;
#7537=CARTESIAN_POINT ( 'NONE',  ( -13.50000000000000533, 199.9250000000000114, -23.38268590217984411 ) ) ;
#7546=CARTESIAN_POINT ( 'NONE',  ( 15.00000000000000178, 245.9874999999999829, 3.464101615137757051 ) ) ;
#7547=LINE ( 'NONE', #10194, #28748 ) ;
#7552=CARTESIAN_POINT ( 'NONE',  ( -27.00000000000000355, 197.4125000012290343, 0.000000000000000000 ) ) ;
#7553=CARTESIAN_POINT ( 'NONE',  ( 15.00000000000000178, 248.7437500012290457, 3.464101615137757051 ) ) ;
#7556=CARTESIAN_POINT ( 'NONE',  ( 26.75643035624999655, 244.6843750006145228, -7.049594010296217766E-16 ) ) ;
#7563=CARTESIAN_POINT ( 'NONE',  ( 13.62178482187501416, 198.2093750006145285, 23.59362340125806767 ) ) ;
#7567=DIRECTION ( 'NONE',  ( 0.000000000000000000, 0.000000000000000000, -1.000000000000000000 ) ) ;
#7576=CARTESIAN_POINT ( 'NONE',  ( 4.999999999999998224, 216.0000000000000000, 3.514718625761427795 ) ) ;
#7577=CARTESIAN_POINT ( 'NONE',  ( 15.24356964375000167, 249.4468750006145399, 3.323476615752272600 ) ) ;
#7581=CARTESIAN_POINT ( 'NONE',  ( 27.24356964375000345, 196.9343750006145228, -3.336375036156643733E-15 ) ) ;
#7583=AXIS2_PLACEMENT_3D ( 'NONE', #6691, #32084, #14654 ) ;
#7586=CARTESIAN_POINT ( 'NONE',  ( 23.87821517812499650, 243.4093750006145171, -4.985214923628404904 ) ) ;
#7592=EDGE_LOOP ( 'NONE', ( #1256, #9796, #27771, #14858 ) ) ;
#7593=CARTESIAN_POINT ( 'NONE',  ( 26.75643035624999655, 245.0593750006144944, -3.323476615752271712 ) ) ;
#7594=LINE ( 'NONE', #22193, #32849 ) ;
#7605=CARTESIAN_POINT ( 'NONE',  ( 15.24356964374999990, 247.4593750006145285, -3.323476615752268604 ) ) ;
#7611=ORIENTED_EDGE ( 'NONE', *, *, #34267, .F. ) ;
#7616=( BOUNDED_CURVE ( )  B_SPLINE_CURVE ( 2, ( #1048, #12240, #9776, #35353, #862, #4087, #32513, #12621, #24185 ),
 .UNSPECIFIED., .F., .F. ) 
 B_SPLINE_CURVE_WITH_KNOTS ( ( 3, 2, 2, 2, 3 ),
 ( 0.5208333333333333703, 0.5277777777777777901, 0.5416666666666666297, 0.5555555555555555802, 0.5625000000000000000 ),
 .UNSPECIFIED. ) 
 CURVE ( )  GEOMETRIC_REPRESENTATION_ITEM ( )  RATIONAL_B_SPLINE_CURVE ( ( 0.9330127018922192983, 0.9330127018922198534, 1.000000000000000000, 0.8660254037844387076, 1.000000000000000000, 0.8660254037844387076, 1.000000000000000000, 0.9330127018922194093, 0.9330127018922194093 ) ) 
 REPRESENTATION_ITEM ( '' )  );
#7620=ORIENTED_EDGE ( 'NONE', *, *, #29790, .T. ) ;
#7627=CARTESIAN_POINT ( 'NONE',  ( 15.00000000000000000, 245.0499999999999829, 0.000000000000000000 ) ) ;
#7628=CARTESIAN_POINT ( 'NONE',  ( 27.24356964375000345, 197.8343750006145569, -3.336375036156643733E-15 ) ) ;
#7629=CARTESIAN_POINT ( 'NONE',  ( 11.70272374968897289, 194.9999999999999432, 24.61780419312783863 ) ) ;
#7630=EDGE_CURVE ( 'NONE', #16688, #23609, #14103, .T. ) ;
#7632=CARTESIAN_POINT ( 'NONE',  ( 0.000000000000000000, 210.0000000000000284, 0.000000000000000000 ) ) ;
#7634=CARTESIAN_POINT ( 'NONE',  ( 26.99999999999999645, 241.6937500012290343, 3.464101615137751278 ) ) ;
#7637=CARTESIAN_POINT ( 'NONE',  ( 13.62178482187499640, 197.4031250006145228, -23.59362340125807123 ) ) ;
#7642=ORIENTED_EDGE ( 'NONE', *, *, #35638, .T. ) ;
#7644=DIRECTION ( 'NONE',  ( 1.000000000000000000, 0.000000000000000000, 0.000000000000000000 ) ) ;
#7647=VECTOR ( 'NONE', #34495, 1000.000000000000000 ) ;
#7657=DIRECTION ( 'NONE',  ( -1.000000000000000000, -6.123233995736766036E-17, -0.000000000000000000 ) ) ;
#7660=AXIS2_PLACEMENT_3D ( 'NONE', #18457, #19723, #2259 ) ;
#7662=CARTESIAN_POINT ( 'NONE',  ( -27.95091016768448000, 207.9223924231847604, -7.730003002181515370 ) ) ;
#7663=ORIENTED_EDGE ( 'NONE', *, *, #24850, .T. ) ;
#7670=CARTESIAN_POINT ( 'NONE',  ( 15.00000000000000178, 247.7874999999999943, 3.464101615137757051 ) ) ;
#7671=CARTESIAN_POINT ( 'NONE',  ( 21.00000000000000000, 246.5968750006145456, -6.646953231504538984 ) ) ;
#7673=CARTESIAN_POINT ( 'NONE',  ( 18.12178482187500350, 244.5343750006145456, 4.985214923628407568 ) ) ;
#7675=CARTESIAN_POINT ( 'NONE',  ( 26.99999999999999645, 249.3812500012290343, -7.347880794884117764E-16 ) ) ;
#7683=ORIENTED_EDGE ( 'NONE', *, *, #10580, .T. ) ;
#7687=CARTESIAN_POINT ( 'NONE',  ( 20.99999999999999289, 241.8437500012290400, -5.999999999999997335 ) ) ;
#7688=CARTESIAN_POINT ( 'NONE',  ( 23.87821517812499650, 249.1468750006145285, -4.985214923628404904 ) ) ;
#7692=CARTESIAN_POINT ( 'NONE',  ( 5.025722718613374163, 215.9903539805198420, -0.3926987779611901819 ) ) ;
#7701=CARTESIAN_POINT ( 'NONE',  ( -13.62178482187498396, 196.7281250006145399, 23.59362340125808188 ) ) ;
#7704=VECTOR ( 'NONE', #16006, 1000.000000000000000 ) ;
#7705=VERTEX_POINT ( 'NONE', #5930 ) ;
#7715=CARTESIAN_POINT ( 'NONE',  ( 19.39230484541326760, 246.4924038105676516, 5.999999999999999112 ) ) ;
#7717=CARTESIAN_POINT ( 'NONE',  ( 15.00000000000000000, 243.2687500012290513, -3.464101615137752610 ) ) ;
#7719=CARTESIAN_POINT ( 'NONE',  ( 5.727106289114498080E-15, 198.3125000000000000, 31.17691453623979214 ) ) ;
#7726=DIRECTION ( 'NONE',  ( -1.000000000000000000, -4.130293990420971855E-17, 0.000000000000000000 ) ) ;
#7729=CARTESIAN_POINT ( 'NONE',  ( 24.00000000000000000, 242.9499999999999886, 5.196152422706629359 ) ) ;
#7735=CARTESIAN_POINT ( 'NONE',  ( 26.99999999999999645, 198.1250000012290400, -15.58845726811990495 ) ) ;
#7739=CARTESIAN_POINT ( 'NONE',  ( 21.00000000000000000, 243.8968750006145001, -6.646953231504538984 ) ) ;
#7746=CARTESIAN_POINT ( 'NONE',  ( 5.778771075727756162E-15, 199.5218750006145854, 31.45816453501075927 ) ) ;
#7760=EDGE_CURVE ( 'NONE', #14209, #3896, #848, .T. ) ;
#7766=AXIS2_PLACEMENT_3D ( 'NONE', #31079, #4912, #36933 ) ;
#7769=CARTESIAN_POINT ( 'NONE',  ( -27.24356964375000345, 198.5093750006145399, 0.000000000000000000 ) ) ;
#7772=FACE_OUTER_BOUND ( 'NONE', #770, .T. ) ;
#7773=CARTESIAN_POINT ( 'NONE',  ( 23.87821517812500005, 241.0093750006145399, 4.985214923628404016 ) ) ;
#7778=ORIENTED_EDGE ( 'NONE', *, *, #32767, .F. ) ;
#7779=CARTESIAN_POINT ( 'NONE',  ( 26.75643035624999655, 244.9843750006145058, 3.323476615752267715 ) ) ;
#7787=VERTEX_POINT ( 'NONE', #25840 ) ;
#7792=CARTESIAN_POINT ( 'NONE',  ( 23.87821517812500005, 245.3968750006145285, 4.985214923628404016 ) ) ;
#7798=EDGE_LOOP ( 'NONE', ( #24788, #3254, #29673, #18802, #27135 ) ) ;
#7802=CARTESIAN_POINT ( 'NONE',  ( 15.00000000000000000, 244.5625000000000000, -3.464101615137752610 ) ) ;
#7814=CARTESIAN_POINT ( 'NONE',  ( 19.39230484541324984, 245.1424038105676857, 5.999999999999991118 ) ) ;
#7815=CARTESIAN_POINT ( 'NONE',  ( 27.24356964375000700, 197.3468750006145740, 15.72908226750537075 ) ) ;
#7816=CARTESIAN_POINT ( 'NONE',  ( -1.045839947578415010E-13, 195.1625000000000512, 27.00000000000000355 ) ) ;
#7820=CARTESIAN_POINT ( 'NONE',  ( 15.00000000000000178, 242.4437500012290343, 3.464101615137757051 ) ) ;
#7823=CARTESIAN_POINT ( 'NONE',  ( 13.62178482187501416, 199.0531250006145285, 23.59362340125806767 ) ) ;
#7826=ORIENTED_EDGE ( 'NONE', *, *, #30917, .T. ) ;
#7827=UNCERTAINTY_MEASURE_WITH_UNIT (LENGTH_MEASURE( 1.000000000000000082E-05 ), #25280, 'distance_accuracy_value', 'NONE');
#7834=EDGE_CURVE ( 'NONE', #1338, #33602, #6901, .T. ) ;
#7847=CARTESIAN_POINT ( 'NONE',  ( 19.39230484541326049, 244.1138461906614054, -5.999999999999997335 ) ) ;
#7848=ORIENTED_EDGE ( 'NONE', *, *, #15755, .T. ) ;
#7854=DIRECTION ( 'NONE',  ( -0.000000000000000000, 1.000000000000000000, -0.000000000000000000 ) ) ;
#7857=CARTESIAN_POINT ( 'NONE',  ( 23.87821517812500005, 248.2093750006145285, 4.985214923628404016 ) ) ;
#7859=CARTESIAN_POINT ( 'NONE',  ( 18.12178482187500350, 240.9343750006145513, 4.985214923628407568 ) ) ;
#7862=CARTESIAN_POINT ( 'NONE',  ( 18.00000000000000000, 248.6312500012290343, -5.196152422706630247 ) ) ;
#7870=EDGE_LOOP ( 'NONE', ( #17169, #11442, #33548, #35305, #29193, #8556, #27146 ) ) ;
#7872=VERTEX_POINT ( 'NONE', #1912 ) ;
#7876=CARTESIAN_POINT ( 'NONE',  ( 15.24356964375000167, 248.4343750006145228, 3.323476615752272600 ) ) ;
#7880=CARTESIAN_POINT ( 'NONE',  ( 15.00964601948014021, 225.9742772813838769, 0.3926987779608852036 ) ) ;
#7890=CARTESIAN_POINT ( 'NONE',  ( 13.62178482187499640, 196.0531250006145285, -23.59362340125807123 ) ) ;
#7894=CARTESIAN_POINT ( 'NONE',  ( 22.60769515458673595, 248.8388461906613998, 5.999999999999999112 ) ) ;
#7908=CARTESIAN_POINT ( 'NONE',  ( -27.00000000000000355, 198.2000000000000171, 0.000000000000000000 ) ) ;
#7919=CARTESIAN_POINT ( 'NONE',  ( 21.00000000000000000, 244.0374999999999943, -6.928203230275506996 ) ) ;
#7923=ORIENTED_EDGE ( 'NONE', *, *, #24856, .F. ) ;
#7925=CARTESIAN_POINT ( 'NONE',  ( 27.00000000000000355, 198.5375000012290627, -3.306546357697854128E-15 ) ) ;
#7929=CARTESIAN_POINT ( 'NONE',  ( 15.24356964375000167, 242.2468750006145228, 3.323476615752272600 ) ) ;
#7930=AXIS2_PLACEMENT_3D ( 'NONE', #31281, #1906, #30550 ) ;
#7935=CARTESIAN_POINT ( 'NONE',  ( 13.62178482187501416, 198.6593750006145456, 23.59362340125806767 ) ) ;
#7939=CARTESIAN_POINT ( 'NONE',  ( 22.60769515458672529, 245.3674038105676800, -6.000000000000004441 ) ) ;
#7943=CARTESIAN_POINT ( 'NONE',  ( 27.00000000000001421, 197.1500000012290172, 15.58845726811988897 ) ) ;
#7950=CIRCLE ( 'NONE', #27315, 8.000000000000000000 ) ;
#7954=CARTESIAN_POINT ( 'NONE',  ( -27.24356964375000345, 197.1593750006145456, 0.000000000000000000 ) ) ;
#7958=CARTESIAN_POINT ( 'NONE',  ( 23.87821517812499650, 240.7093750006145285, -4.985214923628404904 ) ) ;
#7959=CYLINDRICAL_SURFACE ( 'NONE', #35405, 6.000000000000005329 ) ;
#7960=EDGE_CURVE ( 'NONE', #23722, #5552, #2792, .T. ) ;
#7965=CARTESIAN_POINT ( 'NONE',  ( 15.24356964374999990, 243.8968750006145285, 0.000000000000000000 ) ) ;
#7978=CARTESIAN_POINT ( 'NONE',  ( 23.87821517812499650, 244.1968750006145115, -4.985214923628404904 ) ) ;
#7979=CARTESIAN_POINT ( 'NONE',  ( -4.500000000000000888, 210.0000000000000284, 2.500000000000000000 ) ) ;
#7990=CARTESIAN_POINT ( 'NONE',  ( 22.60769515458672529, 245.8736538117967143, -6.000000000000004441 ) ) ;
#7992=FACE_OUTER_BOUND ( 'NONE', #6735, .T. ) ;
#7998=CARTESIAN_POINT ( 'NONE',  ( -13.62178482187500528, 197.0843750006145285, -23.59362340125807123 ) ) ;
#7999=DIRECTION ( 'NONE',  ( 0.000000000000000000, 0.000000000000000000, -1.000000000000000000 ) ) ;
#8004=CARTESIAN_POINT ( 'NONE',  ( 18.00000000000000000, 240.9812500012290570, -5.196152422706630247 ) ) ;
#8009=ORIENTED_EDGE ( 'NONE', *, *, #25166, .F. ) ;
#8016=ADVANCED_FACE ( 'NONE', ( #31652 ), #28613, .F. ) ;
#8023=CARTESIAN_POINT ( 'NONE',  ( -14.29273924364230908, 215.8523247127875493, -5.456133016108021927 ) ) ;
#8031=EDGE_CURVE ( 'NONE', #26868, #30804, #17810, .T. ) ;
#8033=VERTEX_POINT ( 'NONE', #34496 ) ;
#8038=CARTESIAN_POINT ( 'NONE',  ( 20.99999999999999645, 210.0000000000000284, -8.000000000000000000 ) ) ;
#8039=CYLINDRICAL_SURFACE ( 'NONE', #14032, 8.000000000000000000 ) ;
#8041=CARTESIAN_POINT ( 'NONE',  ( 21.00000000000000000, 248.3968750006145285, -6.646953231504538984 ) ) ;
#8043=CARTESIAN_POINT ( 'NONE',  ( 23.87821517812500005, 241.9093750006145456, 4.985214923628404016 ) ) ;
#8047=CARTESIAN_POINT ( 'NONE',  ( -27.00000000000000355, 200.0000000000000000, 0.000000000000000000 ) ) ;
#8056=VERTEX_POINT ( 'NONE', #25965 ) ;
#8057=ORIENTED_EDGE ( 'NONE', *, *, #11411, .T. ) ;
#8060=CARTESIAN_POINT ( 'NONE',  ( 15.00000000000000000, 241.9187500012290570, -3.464101615137752610 ) ) ;
#8062=CARTESIAN_POINT ( 'NONE',  ( 23.87821517812499650, 248.6968750006145115, -4.985214923628404904 ) ) ;
#8064=( BOUNDED_CURVE ( )  B_SPLINE_CURVE ( 2, ( #30609, #16945, #14651, #17133, #26391, #14097, #28669, #5366, #37202 ),
 .UNSPECIFIED., .F., .F. ) 
 B_SPLINE_CURVE_WITH_KNOTS ( ( 3, 2, 2, 2, 3 ),
 ( 0.9021739130434782705, 0.9057971014492753881, 0.9130434782608695121, 0.9202898550724637472, 0.9239130434782608647 ),
 .UNSPECIFIED. ) 
 CURVE ( )  GEOMETRIC_REPRESENTATION_ITEM ( )  RATIONAL_B_SPLINE_CURVE ( ( 0.9330127018922194093, 0.9330127018922194093, 1.000000000000000000, 0.8660254037844387076, 1.000000000000000000, 0.8660254037844387076, 1.000000000000000000, 0.9330127018922194093, 0.9330127018922194093 ) ) 
 REPRESENTATION_ITEM ( '' )  );
#8066=CARTESIAN_POINT ( 'NONE',  ( 15.38158308873937585, 224.9824450966943061, 2.114697272284774776 ) ) ;
#8068=DIRECTION ( 'NONE',  ( -0.000000000000000000, 1.000000000000000000, -0.000000000000000000 ) ) ;
#8073=CIRCLE ( 'NONE', #177, 8.000000000000000000 ) ;
#8076=CARTESIAN_POINT ( 'NONE',  ( -27.24356964375000345, 195.7531250006145456, 0.000000000000000000 ) ) ;
#8084=( BOUNDED_CURVE ( )  B_SPLINE_CURVE ( 2, ( #27537, #21116, #997, #33225, #24140, #13134, #6696, #35682, #15606 ),
 .UNSPECIFIED., .F., .F. ) 
 B_SPLINE_CURVE_WITH_KNOTS ( ( 3, 2, 2, 2, 3 ),
 ( 0.6847826086956522174, 0.6884057971014492239, 0.6956521739130434590, 0.7028985507246376940, 0.7065217391304348116 ),
 .UNSPECIFIED. ) 
 CURVE ( )  GEOMETRIC_REPRESENTATION_ITEM ( )  RATIONAL_B_SPLINE_CURVE ( ( 0.9330127018922192983, 0.9330127018922202975, 1.000000000000000000, 0.8660254037844387076, 1.000000000000000000, 0.8660254037844387076, 1.000000000000000000, 0.9330127018922194093, 0.9330127018922194093 ) ) 
 REPRESENTATION_ITEM ( '' )  );
#8088=EDGE_CURVE ( 'NONE', #24310, #17657, #14639, .T. ) ;
#8092=DIRECTION ( 'NONE',  ( 0.000000000000000000, 0.000000000000000000, -1.000000000000000000 ) ) ;
#8096=CARTESIAN_POINT ( 'NONE',  ( -13.49999999999998401, 197.3750000000000284, 23.38268590217985476 ) ) ;
#8099=CARTESIAN_POINT ( 'NONE',  ( 23.87821517812500005, 248.6593750006145171, 4.985214923628404016 ) ) ;
#8106=CARTESIAN_POINT ( 'NONE',  ( 26.99999999999999645, 243.9625000000000057, -3.464101615137755275 ) ) ;
#8107=CARTESIAN_POINT ( 'NONE',  ( -13.50000000000000533, 198.5749999999999886, -23.38268590217984411 ) ) ;
#8111=ORIENTED_EDGE ( 'NONE', *, *, #36354, .F. ) ;
#8114=CARTESIAN_POINT ( 'NONE',  ( 26.99999999999999645, 195.4250000012290229, -15.58845726811990495 ) ) ;
#8118=CARTESIAN_POINT ( 'NONE',  ( 26.75643035624999655, 242.3968750006145001, 3.323476615752267715 ) ) ;
#8126=CARTESIAN_POINT ( 'NONE',  ( 27.24356964375000345, 197.8343750006145569, -3.336375036156643733E-15 ) ) ;
#8128=( BOUNDED_CURVE ( )  B_SPLINE_CURVE ( 2, ( #29843, #7479, #35530, #10133, #1597, #843, #21338, #23986, #15828 ),
 .UNSPECIFIED., .F., .F. ) 
 B_SPLINE_CURVE_WITH_KNOTS ( ( 3, 2, 2, 2, 3 ),
 ( 0.8125000000000000000, 0.8194444444444444198, 0.8333333333333333703, 0.8472222222222222099, 0.8541666666666667407 ),
 .UNSPECIFIED. ) 
 CURVE ( )  GEOMETRIC_REPRESENTATION_ITEM ( )  RATIONAL_B_SPLINE_CURVE ( ( 0.9330127018922194093, 0.9330127018922194093, 1.000000000000000000, 0.8660254037844387076, 1.000000000000000000, 0.8660254037844387076, 1.000000000000000000, 0.9330127018922187432, 0.9330127018922192983 ) ) 
 REPRESENTATION_ITEM ( '' )  );
#8129=CARTESIAN_POINT ( 'NONE',  ( 22.60769515458672885, 239.8388461906613429, 5.999999999999997335 ) ) ;
#8131=CARTESIAN_POINT ( 'NONE',  ( 0.000000000000000000, 222.9518338469886203, -2.500000000000000000 ) ) ;
#8134=DIRECTION ( 'NONE',  ( 0.000000000000000000, 0.000000000000000000, 1.000000000000000000 ) ) ;
#8142=CARTESIAN_POINT ( 'NONE',  ( 22.60769515458672885, 240.2888461906613884, 5.999999999999997335 ) ) ;
#8146=CARTESIAN_POINT ( 'NONE',  ( -27.24356964375000345, 198.0218750006145569, -15.72908226750537786 ) ) ;
#8149=DIRECTION ( 'NONE',  ( -0.000000000000000000, 1.000000000000000000, -0.000000000000000000 ) ) ;
#8150=CARTESIAN_POINT ( 'NONE',  ( 21.00000000000000000, 241.6468750006145285, -6.646953231504538984 ) ) ;
#8157=CARTESIAN_POINT ( 'NONE',  ( 15.24356964374999990, 245.2093750006145285, -3.323476615752268604 ) ) ;
#8168=CARTESIAN_POINT ( 'NONE',  ( 15.24356964374999990, 243.8968750006145285, 0.000000000000000000 ) ) ;
#8188=CARTESIAN_POINT ( 'NONE',  ( -27.24356964375000345, 195.8093750006145513, 0.000000000000000000 ) ) ;
#8194=CARTESIAN_POINT ( 'NONE',  ( 15.00000000000000000, 242.3687500012290457, -3.464101615137752166 ) ) ;
#8201=CARTESIAN_POINT ( 'NONE',  ( 19.39230484541326760, 246.0986538117967086, 5.999999999999999112 ) ) ;
#8211=VERTEX_POINT ( 'NONE', #17074 ) ;
#8227=( NAMED_UNIT ( * ) PLANE_ANGLE_UNIT ( ) SI_UNIT ( $, .RADIAN. ) );
#8230=CARTESIAN_POINT ( 'NONE',  ( 18.12178482187499640, 248.4343750006145228, -4.985214923628404904 ) ) ;
#8232=CARTESIAN_POINT ( 'NONE',  ( 15.24356964375000167, 241.7968750006145342, 3.323476615752272600 ) ) ;
#8236=EDGE_CURVE ( 'NONE', #3985, #11470, #5445, .T. ) ;
#8237=CARTESIAN_POINT ( 'NONE',  ( 21.00000000000000000, 248.3687500012290457, 6.928203230275506996 ) ) ;
#8244=ORIENTED_EDGE ( 'NONE', *, *, #7271, .F. ) ;
#8249=DIRECTION ( 'NONE',  ( 1.000000000000000000, 0.000000000000000000, 0.000000000000000000 ) ) ;
#8250=CARTESIAN_POINT ( 'NONE',  ( 18.12178482187500350, 249.3718750006145228, 4.985214923628407568 ) ) ;
#8253=CARTESIAN_POINT ( 'NONE',  ( 14.20575797955546626, 216.7942420204377925, 0.4629122958924736242 ) ) ;
#8262=CARTESIAN_POINT ( 'NONE',  ( 13.62178482187499640, 196.9531250006145342, -23.59362340125807123 ) ) ;
#8265=ORIENTED_EDGE ( 'NONE', *, *, #8947, .F. ) ;
#8278=CARTESIAN_POINT ( 'NONE',  ( 5.727106289114498080E-15, 198.7625000000000455, 31.17691453623979214 ) ) ;
#8282=CARTESIAN_POINT ( 'NONE',  ( 26.75643035624999655, 248.7343750006145342, -7.049594010296217766E-16 ) ) ;
#8289=( BOUNDED_CURVE ( )  B_SPLINE_CURVE ( 2, ( #14465, #47, #22819, #25648, #34368, #11614, #8779, #239, #19980 ),
 .UNSPECIFIED., .F., .F. ) 
 B_SPLINE_CURVE_WITH_KNOTS ( ( 3, 2, 2, 2, 3 ),
 ( 0.3152173913043477826, 0.3188405797101449002, 0.3260869565217391353, 0.3333333333333333148, 0.3369565217391304324 ),
 .UNSPECIFIED. ) 
 CURVE ( )  GEOMETRIC_REPRESENTATION_ITEM ( )  RATIONAL_B_SPLINE_CURVE ( ( 0.9330127018922191873, 0.9330127018922187432, 1.000000000000000000, 0.8660254037844387076, 1.000000000000000000, 0.8660254037844387076, 1.000000000000000000, 0.9330127018922194093, 0.9330127018922194093 ) ) 
 REPRESENTATION_ITEM ( '' )  );
#8290=CARTESIAN_POINT ( 'NONE',  ( 26.99999999999999645, 242.5750000000000171, -7.347880794884117764E-16 ) ) ;
#8295=CARTESIAN_POINT ( 'NONE',  ( 27.00000000000001066, 195.3500000012290343, 15.58845726811988897 ) ) ;
#8300=CARTESIAN_POINT ( 'NONE',  ( 18.12178482187499640, 241.6843750006145513, -4.985214923628404904 ) ) ;
#8303=CARTESIAN_POINT ( 'NONE',  ( 20.99999999999999289, 240.8874999999999886, -5.999999999999997335 ) ) ;
#8309=CARTESIAN_POINT ( 'NONE',  ( 27.24356964374999635, 197.4218750006145342, -15.72908226750539029 ) ) ;
#8313=CARTESIAN_POINT ( 'NONE',  ( 19.39230484541326760, 240.6424038105676573, 5.999999999999999112 ) ) ;
#8324=CARTESIAN_POINT ( 'NONE',  ( 13.49999999999999645, 195.0125000012290570, -23.38268590217984766 ) ) ;
#8325=CARTESIAN_POINT ( 'NONE',  ( 24.00000000000000000, 248.4062500012290400, 5.196152422706629359 ) ) ;
#8330=CARTESIAN_POINT ( 'NONE',  ( -27.24356964374999279, 195.8468750006145740, 15.72908226750539384 ) ) ;
#8333=CARTESIAN_POINT ( 'NONE',  ( 20.99999999999997868, 246.5687500012290343, 5.999999999999999112 ) ) ;
#8334=CARTESIAN_POINT ( 'NONE',  ( 15.24356964375000167, 239.9968750006145513, 3.323476615752272600 ) ) ;
#8335=CARTESIAN_POINT ( 'NONE',  ( -27.24356964374999279, 198.4906250006145569, 15.72908226750539384 ) ) ;
#8340=CARTESIAN_POINT ( 'NONE',  ( 23.87821517812499650, 241.9468750006145115, -4.985214923628404904 ) ) ;
#8345=( BOUNDED_CURVE ( )  B_SPLINE_CURVE ( 2, ( #26112, #8869, #9060, #6017, #14748, #25743, #6211, #31434, #17601 ),
 .UNSPECIFIED., .F., .F. ) 
 B_SPLINE_CURVE_WITH_KNOTS ( ( 3, 2, 2, 2, 3 ),
 ( 0.03260869565217391908, 0.03623188405797101580, 0.04347826086956521618, 0.05072463768115942351, 0.05434782608695652023 ),
 .UNSPECIFIED. ) 
 CURVE ( )  GEOMETRIC_REPRESENTATION_ITEM ( )  RATIONAL_B_SPLINE_CURVE ( ( 0.9330127018922192983, 0.9330127018922194093, 1.000000000000000000, 0.8660254037844387076, 1.000000000000000000, 0.8660254037844387076, 1.000000000000000000, 0.9330127018922194093, 0.9330127018922191873 ) ) 
 REPRESENTATION_ITEM ( '' )  );
#8349=EDGE_CURVE ( 'NONE', #36021, #9298, #17086, .T. ) ;
#8350=CARTESIAN_POINT ( 'NONE',  ( 23.87821517812499650, 245.5468750006145058, -4.985214923628404904 ) ) ;
#8372=CARTESIAN_POINT ( 'NONE',  ( 13.62178482187501416, 195.9593750006145569, 23.59362340125806767 ) ) ;
#8377=ORIENTED_EDGE ( 'NONE', *, *, #5296, .F. ) ;
#8378=CARTESIAN_POINT ( 'NONE',  ( 26.75643035624999655, 249.1093750006145058, -3.323476615752271712 ) ) ;
#8384=AXIS2_PLACEMENT_3D ( 'NONE', #14201, #25752, #15323 ) ;
#8387=( BOUNDED_CURVE ( )  B_SPLINE_CURVE ( 2, ( #28360, #25337, #28912, #11305, #11118, #22695, #36885, #19673, #22506, #10931, #5417, #2396, #25519, #16636, #37257, #14518, #17185, #31576, #31761, #16998, #34053, #34239, #20212, #2208, #28538, #13970, #37438, #23240, #31398, #2581, #8282, #28725, #8099, #19855, #11487, #31212, #5241, #23056, #22873, #5599, #14151, #11666, #34424, #8461, #20031, #5791, #34602, #2763, #14335, #8644, #2948, #31032, #26074, #102, #34788, #8832, #5053, #35336, #3321, #12227, #32690, #12607, #17929, #9393, #26440, #15265, #20404, #32500, #26818, #1036, #21153, #23607, #20967, #14892, #23799, #6734, #17741, #31945, #20773, #6546, #35153, #5977, #26252, #9204, #34973, #23990, #17557, #18307, #3883, #15077, #9016, #6167, #3135, #24173, #32129, #29847, #32317, #3509, #20586, #6358, #14703, #847, #35717, #29092, #9579, #287, #15457, #11853, #29473, #29281, #26626, #656, #23422, #472, #18119, #29661, #12040, #27009, #12419, #3697, #35534, #22082, #25096, #36093, #1411, #30039, #27381, #18873, #16023, #33442, #12987, #7119, #36275, #15645, #21529, #10137, #9765, #30422, #6928, #9948, #13169, #4073, #7673, #27572, #24544, #15833, #27195, #35905, #1220, #12793, #21710, #33075, #4257, #32881, #4444, #30792, #7483, #10320, #10504, #33260, #24362, #7299, #36462, #18500, #1601, #18690, #4629, #1970, #24724, #21893, #19061, #30613, #30232, #16209, #27757, #1787, #13355, #24910, #33634, #19252, #4815, #27940, #16395, #13543, #21342, #11437, #31525, #10879, #34553, #11066, #19807, #13737, #25470, #19431, #34371, #2348, #2156, #31712, #5551, #8593, #25285, #13920, #22452, #31342, #37020, #36836, #14468, #22640, #34187, #33999, #25837, #17136, #8043, #5369, #5739, #8232, #16948, #4999, #31165, #28490, #19983, #2534, #22822, #28309, #19619, #25652, #16581, #5188, #14100, #36653, #37205, #33821, #16762, #11252, #30981, #8414, #28672, #2710, #7859, #23004, #14286, #28126, #37385, #20164, #17319, #28861, #22268, #2895, #10690, #12180, #26582, #26773, #11993, #8783, #23565, #11806, #3839, #14847, #31897, #9349, #9158, #26395, #428, #20541, #23754, #5926, #6113, #20920, #20355 ),
 .UNSPECIFIED., .F., .F. ) 
 B_SPLINE_CURVE_WITH_KNOTS ( ( 3, 2, 2, 2, 2, 2, 2, 2, 2, 2, 2, 2, 2, 2, 2, 2, 2, 2, 2, 2, 2, 2, 2, 2, 2, 2, 2, 2, 2, 2, 2, 2, 2, 2, 2, 2, 2, 2, 2, 2, 2, 2, 2, 2, 2, 2, 2, 2, 2, 2, 2, 2, 2, 2, 2, 2, 2, 2, 2, 2, 2, 2, 2, 2, 2, 2, 2, 2, 2, 2, 2, 2, 2, 2, 2, 2, 2, 2, 2, 2, 2, 2, 2, 2, 2, 2, 2, 2, 2, 2, 2, 2, 2, 2, 2, 2, 2, 2, 2, 2, 2, 2, 2, 2, 2, 2, 2, 2, 2, 2, 2, 2, 2, 2, 2, 2, 2, 2, 2, 2, 2, 2, 2, 2, 2, 2, 2, 2, 2, 2, 2, 2, 2, 2, 3 ),
 ( 0.000000000000000000, 0.007246376811594202987, 0.01449275362318840597, 0.02173913043478260809, 0.02898550724637681195, 0.03623188405797101580, 0.04347826086956521618, 0.05072463768115942351, 0.05797101449275362389, 0.06521739130434782428, 0.07246376811594203160, 0.07971014492753622505, 0.08695652173913043237, 0.09420289855072463969, 0.1014492753623188470, 0.1086956521739130405, 0.1159420289855072478, 0.1231884057971014412, 0.1304347826086956486, 0.1376811594202898559, 0.1449275362318840632, 0.1521739130434782705, 0.1594202898550724501, 0.1666666666666666574, 0.1739130434782608647, 0.1811594202898550721, 0.1884057971014492794, 0.1956521739130434867, 0.2028985507246376940, 0.2101449275362318736, 0.2173913043478260809, 0.2246376811594202882, 0.2318840579710144956, 0.2391304347826087306, 0.2463768115942028825, 0.2536231884057971175, 0.2608695652173912971, 0.2681159420289855322, 0.2753623188405797118, 0.2826086956521738913, 0.2898550724637681264, 0.2971014492753623060, 0.3043478260869565410, 0.3115942028985507206, 0.3188405797101449002, 0.3260869565217391353, 0.3333333333333333148, 0.3405797101449275499, 0.3478260869565217295, 0.3550724637681159646, 0.3623188405797101441, 0.3695652173913043237, 0.3768115942028985588, 0.3840579710144927383, 0.3913043478260869734, 0.3985507246376811530, 0.4057971014492753881, 0.4130434782608695676, 0.4202898550724637472, 0.4275362318840579823, 0.4347826086956521618, 0.4420289855072463969, 0.4492753623188405765, 0.4565217391304347561, 0.4637681159420289911, 0.4710144927536231707, 0.4782608695652174613, 0.4855072463768115854, 0.4927536231884057649, 0.5000000000000000000, 0.5072463768115942351, 0.5144927536231883591, 0.5217391304347825942, 0.5289855072463768293, 0.5362318840579710644, 0.5434782608695651884, 0.5507246376811594235, 0.5579710144927536586, 0.5652173913043477826, 0.5724637681159420177, 0.5797101449275362528, 0.5869565217391304879, 0.5942028985507246119, 0.6014492753623188470, 0.6086956521739130821, 0.6159420289855072062, 0.6231884057971014412, 0.6304347826086956763, 0.6376811594202898004, 0.6449275362318840354, 0.6521739130434782705, 0.6594202898550725056, 0.6666666666666666297, 0.6739130434782608647, 0.6811594202898550998, 0.6884057971014492239, 0.6956521739130434590, 0.7028985507246376940, 0.7101449275362319291, 0.7173913043478260532, 0.7246376811594202882, 0.7318840579710145233, 0.7391304347826086474, 0.7463768115942028825, 0.7536231884057971175, 0.7608695652173913526, 0.7681159420289854767, 0.7753623188405797118, 0.7826086956521739468, 0.7898550724637680709, 0.7971014492753623060, 0.8043478260869565410, 0.8115942028985507761, 0.8188405797101449002, 0.8260869565217391353, 0.8333333333333333703, 0.8405797101449274944, 0.8478260869565217295, 0.8550724637681159646, 0.8623188405797101996, 0.8695652173913043237, 0.8768115942028985588, 0.8840579710144927938, 0.8913043478260869179, 0.8985507246376811530, 0.9057971014492753881, 0.9130434782608695121, 0.9202898550724637472, 0.9275362318840579823, 0.9347826086956522174, 0.9420289855072463414, 0.9492753623188405765, 0.9565217391304349226, 0.9637681159420289356, 0.9662082973083875315 ),
 .UNSPECIFIED. ) 
 CURVE ( )  GEOMETRIC_REPRESENTATION_ITEM ( )  RATIONAL_B_SPLINE_CURVE ( ( 1.000000000000000000, 0.8660254037844387076, 1.000000000000000000, 0.8660254037844387076, 1.000000000000000000, 0.8660254037844387076, 1.000000000000000000, 0.8660254037844387076, 1.000000000000000000, 0.8660254037844387076, 1.000000000000000000, 0.8660254037844387076, 1.000000000000000000, 0.8660254037844387076, 1.000000000000000000, 0.8660254037844387076, 1.000000000000000000, 0.8660254037844387076, 1.000000000000000000, 0.8660254037844387076, 1.000000000000000000, 0.8660254037844387076, 1.000000000000000000, 0.8660254037844387076, 1.000000000000000000, 0.8660254037844387076, 1.000000000000000000, 0.8660254037844387076, 1.000000000000000000, 0.8660254037844387076, 1.000000000000000000, 0.8660254037844387076, 1.000000000000000000, 0.8660254037844387076, 1.000000000000000000, 0.8660254037844387076, 1.000000000000000000, 0.8660254037844387076, 1.000000000000000000, 0.8660254037844387076, 1.000000000000000000, 0.8660254037844387076, 1.000000000000000000, 0.8660254037844387076, 1.000000000000000000, 0.8660254037844387076, 1.000000000000000000, 0.8660254037844387076, 1.000000000000000000, 0.8660254037844387076, 1.000000000000000000, 0.8660254037844387076, 1.000000000000000000, 0.8660254037844387076, 1.000000000000000000, 0.8660254037844387076, 1.000000000000000000, 0.8660254037844387076, 1.000000000000000000, 0.8660254037844387076, 1.000000000000000000, 0.8660254037844387076, 1.000000000000000000, 0.8660254037844387076, 1.000000000000000000, 0.8660254037844387076, 1.000000000000000000, 0.8660254037844387076, 1.000000000000000000, 0.8660254037844387076, 1.000000000000000000, 0.8660254037844387076, 1.000000000000000000, 0.8660254037844387076, 1.000000000000000000, 0.8660254037844387076, 1.000000000000000000, 0.8660254037844387076, 1.000000000000000000, 0.8660254037844387076, 1.000000000000000000, 0.8660254037844387076, 1.000000000000000000, 0.8660254037844387076, 1.000000000000000000, 0.8660254037844387076, 1.000000000000000000, 0.8660254037844387076, 1.000000000000000000, 0.8660254037844387076, 1.000000000000000000, 0.8660254037844387076, 1.000000000000000000, 0.8660254037844387076, 1.000000000000000000, 0.8660254037844387076, 1.000000000000000000, 0.8660254037844387076, 1.000000000000000000, 0.8660254037844387076, 1.000000000000000000, 0.8660254037844387076, 1.000000000000000000, 0.8660254037844387076, 1.000000000000000000, 0.8660254037844387076, 1.000000000000000000, 0.8660254037844387076, 1.000000000000000000, 0.8660254037844387076, 1.000000000000000000, 0.8660254037844387076, 1.000000000000000000, 0.8660254037844387076, 1.000000000000000000, 0.8660254037844387076, 1.000000000000000000, 0.8660254037844387076, 1.000000000000000000, 0.8660254037844387076, 1.000000000000000000, 0.8660254037844387076, 1.000000000000000000, 0.8660254037844387076, 1.000000000000000000, 0.8660254037844387076, 1.000000000000000000, 0.8660254037844387076, 1.000000000000000000, 0.8660254037844387076, 1.000000000000000000, 0.8660254037844387076, 1.000000000000000000, 0.8660254037844387076, 1.000000000000000000, 0.8660254037844387076, 1.000000000000000000, 0.8660254037844387076, 1.000000000000000000, 0.8660254037844387076, 1.000000000000000000, 0.8660254037844387076, 1.000000000000000000, 0.8660254037844387076, 1.000000000000000000, 0.8660254037844387076, 1.000000000000000000, 0.8660254037844387076, 1.000000000000000000, 0.8660254037844387076, 1.000000000000000000, 0.8660254037844387076, 1.000000000000000000, 0.8660254037844387076, 1.000000000000000000, 0.8660254037844387076, 1.000000000000000000, 0.8660254037844387076, 1.000000000000000000, 0.8660254037844387076, 1.000000000000000000, 0.8660254037844387076, 1.000000000000000000, 0.8660254037844387076, 1.000000000000000000, 0.8660254037844387076, 1.000000000000000000, 0.8660254037844387076, 1.000000000000000000, 0.8660254037844387076, 1.000000000000000000, 0.8660254037844387076, 1.000000000000000000, 0.8660254037844387076, 1.000000000000000000, 0.8660254037844387076, 1.000000000000000000, 0.8660254037844387076, 1.000000000000000000, 0.8660254037844387076, 1.000000000000000000, 0.8660254037844387076, 1.000000000000000000, 0.8660254037844387076, 1.000000000000000000, 0.8660254037844387076, 1.000000000000000000, 0.8660254037844387076, 1.000000000000000000, 0.8660254037844387076, 1.000000000000000000, 0.8660254037844387076, 1.000000000000000000, 0.8660254037844387076, 1.000000000000000000, 0.8660254037844387076, 1.000000000000000000, 0.8660254037844387076, 1.000000000000000000, 0.8660254037844387076, 1.000000000000000000, 0.8660254037844387076, 1.000000000000000000, 0.8660254037844387076, 1.000000000000000000, 0.8660254037844387076, 1.000000000000000000, 0.8660254037844387076, 1.000000000000000000, 0.8660254037844387076, 1.000000000000000000, 0.8660254037844387076, 1.000000000000000000, 0.8660254037844387076, 1.000000000000000000, 0.8660254037844387076, 1.000000000000000000, 0.8660254037844387076, 1.000000000000000000, 0.8660254037844387076, 1.000000000000000000, 0.8660254037844387076, 1.000000000000000000, 0.8660254037844387076, 1.000000000000000000, 0.8660254037844387076, 1.000000000000000000, 0.8660254037844387076, 1.000000000000000000, 0.8660254037844387076, 1.000000000000000000, 0.8660254037844387076, 1.000000000000000000, 0.8660254037844387076, 1.000000000000000000, 0.8660254037844387076, 1.000000000000000000, 0.8660254037844387076, 1.000000000000000000, 0.8660254037844387076, 1.000000000000000000, 0.8660254037844387076, 1.000000000000000000, 0.8660254037844387076, 1.000000000000000000, 0.8660254037844387076, 1.000000000000000000, 0.8660254037844387076, 1.000000000000000000, 0.8660254037844387076, 1.000000000000000000, 0.8660254037844387076, 1.000000000000000000, 0.8660254037844387076, 1.000000000000000000, 0.8660254037844387076, 1.000000000000000000, 0.8660254037844387076, 1.000000000000000000, 0.8660254037844387076, 1.000000000000000000, 0.8660254037844387076, 1.000000000000000000, 0.8660254037844387076, 1.000000000000000000, 0.8660254037844387076, 1.000000000000000000, 0.9548847207714133978, 0.9401541335272454170 ) ) 
 REPRESENTATION_ITEM ( '' )  );
#8391=CARTESIAN_POINT ( 'NONE',  ( -1.045839947578415010E-13, 196.5125000000000455, 27.00000000000000355 ) ) ;
#8396=VECTOR ( 'NONE', #24396, 1000.000000000000000 ) ;
#8407=CARTESIAN_POINT ( 'NONE',  ( -27.00000000000000355, 196.0625000012290400, 0.000000000000000000 ) ) ;
#8409=CARTESIAN_POINT ( 'NONE',  ( -27.00000000000000355, 199.0625000000000000, -15.58845726811989429 ) ) ;
#8412=CARTESIAN_POINT ( 'NONE',  ( 26.75643035624999655, 244.1968750006145399, 3.323476615752267715 ) ) ;
#8414=CARTESIAN_POINT ( 'NONE',  ( 26.75643035624999655, 241.0468750006145342, 3.323476615752267271 ) ) ;
#8417=CARTESIAN_POINT ( 'NONE',  ( 23.99999999999999645, 249.0062500012290627, -5.196152422706631135 ) ) ;
#8430=CARTESIAN_POINT ( 'NONE',  ( 20.99999999999999645, 185.0294372515228645, 0.000000000000000000 ) ) ;
#8434=CARTESIAN_POINT ( 'NONE',  ( 6.642437016335149380, 215.3840861188750750, -2.655215585727014993 ) ) ;
#8442=CARTESIAN_POINT ( 'NONE',  ( -13.62178482187498396, 194.9281250006145569, 23.59362340125808188 ) ) ;
#8445=VERTEX_POINT ( 'NONE', #36879 ) ;
#8449=EDGE_CURVE ( 'NONE', #25376, #23017, #10323, .T. ) ;
#8450=CARTESIAN_POINT ( 'NONE',  ( 15.00000000000000178, 243.2874999999999943, 3.464101615137757051 ) ) ;
#8454=DIRECTION ( 'NONE',  ( -0.000000000000000000, -1.000000000000000000, -0.000000000000000000 ) ) ;
#8458=CARTESIAN_POINT ( 'NONE',  ( -13.49999999999998401, 198.2750000000000057, 23.38268590217985476 ) ) ;
#8461=CARTESIAN_POINT ( 'NONE',  ( 26.75643035624999655, 248.2468750006145797, 3.323476615752267271 ) ) ;
#8468=CARTESIAN_POINT ( 'NONE',  ( 18.00000000000000355, 244.2249999999999943, 5.196152422706632912 ) ) ;
#8472=ORIENTED_EDGE ( 'NONE', *, *, #19639, .T. ) ;
#8474=CARTESIAN_POINT ( 'NONE',  ( 27.00000000000001066, 196.7000000012290286, 15.58845726811988897 ) ) ;
#8475=CARTESIAN_POINT ( 'NONE',  ( 1.069080835302379631E-14, 196.6250000012290400, 27.00000000000000000 ) ) ;
#8480=CARTESIAN_POINT ( 'NONE',  ( 26.75643035624999655, 243.2968750006145342, 3.323476615752267715 ) ) ;
#8485=EDGE_CURVE ( 'NONE', #18678, #24310, #356, .T. ) ;
#8489=CARTESIAN_POINT ( 'NONE',  ( 26.23080272481033148, 195.0000000000000568, 6.985708249719166041 ) ) ;
#8490=CARTESIAN_POINT ( 'NONE',  ( -27.24356964374999990, 195.3218750006145399, -15.72908226750537786 ) ) ;
#8502=( BOUNDED_CURVE ( )  B_SPLINE_CURVE ( 2, ( #37494, #5664, #3525, #31635, #29487, #8523, #15090, #34660, #12433 ),
 .UNSPECIFIED., .F., .F. ) 
 B_SPLINE_CURVE_WITH_KNOTS ( ( 3, 2, 2, 2, 3 ),
 ( 0.5978260869565217295, 0.6014492753623188470, 0.6086956521739130821, 0.6159420289855072062, 0.6195652173913043237 ),
 .UNSPECIFIED. ) 
 CURVE ( )  GEOMETRIC_REPRESENTATION_ITEM ( )  RATIONAL_B_SPLINE_CURVE ( ( 0.9330127018922194093, 0.9330127018922194093, 1.000000000000000000, 0.8660254037844387076, 1.000000000000000000, 0.8660254037844387076, 1.000000000000000000, 0.9330127018922194093, 0.9330127018922194093 ) ) 
 REPRESENTATION_ITEM ( '' )  );
#8504=DIRECTION ( 'NONE',  ( 0.000000000000000000, 0.000000000000000000, -1.000000000000000000 ) ) ;
#8505=EDGE_CURVE ( 'NONE', #23955, #22812, #12990, .T. ) ;
#8511=CARTESIAN_POINT ( 'NONE',  ( -27.24356964375000345, 196.2593750006145399, 0.000000000000000000 ) ) ;
#8514=CARTESIAN_POINT ( 'NONE',  ( 20.99999999999999645, 185.0294372515228645, 0.000000000000000000 ) ) ;
#8515=CARTESIAN_POINT ( 'NONE',  ( 26.75643035624999655, 240.1843750006145513, -7.049594010296217766E-16 ) ) ;
#8516=CARTESIAN_POINT ( 'NONE',  ( 13.62178482187499640, 198.3031250006145285, -23.59362340125807123 ) ) ;
#8521=CARTESIAN_POINT ( 'NONE',  ( -27.24356964375000345, 197.5531250006145285, 0.000000000000000000 ) ) ;
#8522=CARTESIAN_POINT ( 'NONE',  ( 15.24356964375000167, 241.6843750006144944, 3.323476615752272600 ) ) ;
#8523=CARTESIAN_POINT ( 'NONE',  ( 15.00000000000000000, 243.6625000000000227, -3.464101615137752610 ) ) ;
#8524=EDGE_CURVE ( 'NONE', #30424, #23066, #282, .T. ) ;
#8531=CARTESIAN_POINT ( 'NONE',  ( 18.12178482187500350, 242.6218750006145228, 4.985214923628407568 ) ) ;
#8532=CARTESIAN_POINT ( 'NONE',  ( 22.60769515458672174, 246.5888461906613998, 6.000000000000004441 ) ) ;
#8538=CARTESIAN_POINT ( 'NONE',  ( 18.00000000000000000, 240.9812500012290570, -5.196152422706630247 ) ) ;
#8541=CARTESIAN_POINT ( 'NONE',  ( -20.72401335767156638, 195.0000000000000000, -17.30627455141886983 ) ) ;
#8542=CARTESIAN_POINT ( 'NONE',  ( 22.60769515458671108, 244.3388461906613429, 6.000000000000010658 ) ) ;
#8549=LINE ( 'NONE', #17274, #3522 ) ;
#8551=CARTESIAN_POINT ( 'NONE',  ( -27.24356964374999635, 194.9468750006145399, 15.72908226750539384 ) ) ;
#8556=ORIENTED_EDGE ( 'NONE', *, *, #29518, .T. ) ;
#8557=EDGE_LOOP ( 'NONE', ( #35033, #7027, #19253, #14070 ) ) ;
#8559=CARTESIAN_POINT ( 'NONE',  ( 15.00000000000000178, 240.1937500012290627, 3.464101615137757051 ) ) ;
#8565=VERTEX_POINT ( 'NONE', #26434 ) ;
#8571=CARTESIAN_POINT ( 'NONE',  ( -20.01834529145943620, 195.0000000000000000, 18.41905743281650132 ) ) ;
#8584=VECTOR ( 'NONE', #11480, 1000.000000000000000 ) ;
#8588=CARTESIAN_POINT ( 'NONE',  ( 13.49999999999999645, 196.3625000012290513, -23.38268590217984766 ) ) ;
#8590=CARTESIAN_POINT ( 'NONE',  ( 0.000000000000000000, 210.0000000000000284, 0.000000000000000000 ) ) ;
#8591=CARTESIAN_POINT ( 'NONE',  ( 26.75643035624999655, 245.0968750006145456, 3.323476615752267715 ) ) ;
#8593=CARTESIAN_POINT ( 'NONE',  ( 26.75643035624999655, 242.3968750006145285, 3.323476615752267271 ) ) ;
#8597=CARTESIAN_POINT ( 'NONE',  ( 21.00000000000000000, 245.2187500012290400, 6.928203230275506996 ) ) ;
#8598=VERTEX_POINT ( 'NONE', #30418 ) ;
#8606=ORIENTED_EDGE ( 'NONE', *, *, #35270, .T. ) ;
#8612=CARTESIAN_POINT ( 'NONE',  ( 15.24356964375000167, 247.0843750006145285, 3.323476615752272600 ) ) ;
#8616=CARTESIAN_POINT ( 'NONE',  ( 8.945811011643066024, 214.5203208706302291, -3.964960503608339959 ) ) ;
#8625=CARTESIAN_POINT ( 'NONE',  ( 20.99999999999998579, 247.6374999999999886, -5.999999999999997335 ) ) ;
#8628=ORIENTED_EDGE ( 'NONE', *, *, #33294, .T. ) ;
#8629=CARTESIAN_POINT ( 'NONE',  ( 22.60769515458672885, 249.0236538117967200, -5.999999999999997335 ) ) ;
#8639=CARTESIAN_POINT ( 'NONE',  ( 7.234628195640322446, 195.6325961894323484, 26.99999999999999645 ) ) ;
#8641=CARTESIAN_POINT ( 'NONE',  ( -13.49999999999998401, 196.0250000000000057, 23.38268590217985476 ) ) ;
#8644=CARTESIAN_POINT ( 'NONE',  ( 15.24356964374999990, 248.0218750006145285, -3.323476615752268604 ) ) ;
#8645=ORIENTED_EDGE ( 'NONE', *, *, #20704, .T. ) ;
#8652=CARTESIAN_POINT ( 'NONE',  ( 15.00000000000000000, 242.3500000000000227, 0.000000000000000000 ) ) ;
#8658=CARTESIAN_POINT ( 'NONE',  ( 13.49999999999999645, 195.4625000012290172, -23.38268590217984766 ) ) ;
#8659=AXIS2_PLACEMENT_3D ( 'NONE', #17413, #8870, #31989 ) ;
#8660=CARTESIAN_POINT ( 'NONE',  ( 20.99999999999999645, 250.0000000000000000, -8.000000000000000000 ) ) ;
#8663=ADVANCED_FACE ( 'NONE', ( #33438 ), #35713, .F. ) ;
#8664=CARTESIAN_POINT ( 'NONE',  ( 23.87821517812500005, 241.4593750006145285, 4.985214923628404016 ) ) ;
#8671=CARTESIAN_POINT ( 'NONE',  ( 24.06985121900113000, 194.9999999999999432, -12.35451244266598181 ) ) ;
#8672=CARTESIAN_POINT ( 'NONE',  ( 27.24356964375000700, 195.0968750006145456, 15.72908226750537075 ) ) ;
#8688=CARTESIAN_POINT ( 'NONE',  ( -7.234628195640263826, 195.0700961906613600, -27.00000000000003553 ) ) ;
#8692=CARTESIAN_POINT ( 'NONE',  ( -27.24356964375000345, 195.7718750006145569, -15.72908226750537786 ) ) ;
#8695=CARTESIAN_POINT ( 'NONE',  ( -7.234628195640302017, 198.2924038105676630, 27.00000000000000711 ) ) ;
#8696=CARTESIAN_POINT ( 'NONE',  ( 18.00000000000000355, 247.3750000000000000, 5.196152422706632912 ) ) ;
#8697=CARTESIAN_POINT ( 'NONE',  ( -27.24356964375000345, 199.7656250006145342, -15.72908226750537786 ) ) ;
#8703=CARTESIAN_POINT ( 'NONE',  ( -13.62178482187500528, 197.9281250006145569, -23.59362340125807123 ) ) ;
#8704=CARTESIAN_POINT ( 'NONE',  ( 18.12178482187500350, 242.1718750006145058, 4.985214923628407568 ) ) ;
#8715=CARTESIAN_POINT ( 'NONE',  ( 26.75643035624999655, 241.4593750006145001, -3.323476615752271268 ) ) ;
#8726=CARTESIAN_POINT ( 'NONE',  ( 15.00000000000000000, 241.5062500012290627, 0.000000000000000000 ) ) ;
#8729=CARTESIAN_POINT ( 'NONE',  ( 18.12178482187499640, 242.9218750006145058, -4.985214923628404904 ) ) ;
#8736=CARTESIAN_POINT ( 'NONE',  ( 26.99999999999999645, 241.1875000000000000, 3.464101615137751278 ) ) ;
#8737=AXIS2_PLACEMENT_3D ( 'NONE', #24286, #35831, #32616 ) ;
#8738=CARTESIAN_POINT ( 'NONE',  ( 15.00000000000000178, 242.4437500012290343, 3.464101615137757051 ) ) ;
#8739=CARTESIAN_POINT ( 'NONE',  ( -28.99999999999999645, 201.9999999999999716, -1.007612034238798379E-23 ) ) ;
#8746=CARTESIAN_POINT ( 'NONE',  ( 26.99999999999999645, 239.9312500012290457, -7.347880794884117764E-16 ) ) ;
#8751=ORIENTED_EDGE ( 'NONE', *, *, #26547, .T. ) ;
#8756=CARTESIAN_POINT ( 'NONE',  ( 20.99999999999999645, 248.0593750006144944, 6.646953231504538984 ) ) ;
#8758=CARTESIAN_POINT ( 'NONE',  ( -22.24010127653566471, 195.0000000000001421, -15.49061856779472279 ) ) ;
#8768=EDGE_CURVE ( 'NONE', #22812, #22517, #8128, .T. ) ;
#8777=LINE ( 'NONE', #15027, #1692 ) ;
#8779=CARTESIAN_POINT ( 'NONE',  ( 24.00000000000000000, 246.1562500012290400, 5.196152422706629359 ) ) ;
#8781=CARTESIAN_POINT ( 'NONE',  ( 26.75643035624999655, 246.5218750006145285, -3.323476615752271712 ) ) ;
#8783=CARTESIAN_POINT ( 'NONE',  ( 15.24356964374999990, 240.3718750006145228, -3.323476615752268604 ) ) ;
#8787=CARTESIAN_POINT ( 'NONE',  ( 18.00000000000000000, 245.9312500012290457, -5.196152422706630247 ) ) ;
#8798=ORIENTED_EDGE ( 'NONE', *, *, #17995, .F. ) ;
#8801=CARTESIAN_POINT ( 'NONE',  ( 21.00000000000000000, 246.0343750006144887, -6.646953231504538984 ) ) ;
#8804=CARTESIAN_POINT ( 'NONE',  ( 11.24016333012526836, 213.6599387512111434, -4.770645753568232728 ) ) ;
#8815=ORIENTED_EDGE ( 'NONE', *, *, #32108, .T. ) ;
#8829=CARTESIAN_POINT ( 'NONE',  ( -27.24356964374999635, 199.4468750006145399, 15.72908226750539384 ) ) ;
#8832=CARTESIAN_POINT ( 'NONE',  ( 26.75643035624999655, 247.7968750006145342, 3.323476615752267271 ) ) ;
#8839=CARTESIAN_POINT ( 'NONE',  ( 26.99999999999999645, 240.8125000000000000, -3.464101615137755275 ) ) ;
#8843=ORIENTED_EDGE ( 'NONE', *, *, #32287, .F. ) ;
#8845=CARTESIAN_POINT ( 'NONE',  ( -26.99999999999998934, 196.1000000012290627, 15.58845726811991561 ) ) ;
#8846=CARTESIAN_POINT ( 'NONE',  ( -27.00000000000000355, 196.4750000012289775, -15.58845726811989429 ) ) ;
#8849=CARTESIAN_POINT ( 'NONE',  ( 18.12178482187499640, 240.3343750006145285, -4.985214923628404904 ) ) ;
#8850=( BOUNDED_CURVE ( )  B_SPLINE_CURVE ( 3, ( #8038, #19426, #16204, #10685 ),
 .UNSPECIFIED., .F., .F. ) 
 B_SPLINE_CURVE_WITH_KNOTS ( ( 4, 4 ),
 ( 1.570796326794900555, 4.712388980384686121 ),
 .UNSPECIFIED. ) 
 CURVE ( )  GEOMETRIC_REPRESENTATION_ITEM ( )  RATIONAL_B_SPLINE_CURVE ( ( 1.000000000000000000, 0.3333333333333359239, 0.3333333333333359239, 1.000000000000000000 ) ) 
 REPRESENTATION_ITEM ( '' )  );
#8858=CARTESIAN_POINT ( 'NONE',  ( 13.62178482187499640, 195.2093750006145569, -23.59362340125807123 ) ) ;
#8863=CARTESIAN_POINT ( 'NONE',  ( 13.49999999999999645, 198.9500000000000171, -23.38268590217984766 ) ) ;
#8869=CARTESIAN_POINT ( 'NONE',  ( 19.39230484541326760, 249.6424038105677141, 5.999999999999999112 ) ) ;
#8870=DIRECTION ( 'NONE',  ( -0.000000000000000000, -1.000000000000000000, -0.000000000000000000 ) ) ;
#8876=FACE_OUTER_BOUND ( 'NONE', #35769, .T. ) ;
#8880=CARTESIAN_POINT ( 'NONE',  ( 26.99999999999999645, 247.5250000000000057, -7.347880794884117764E-16 ) ) ;
#8881=CARTESIAN_POINT ( 'NONE',  ( 5.778771075727756162E-15, 197.6656250006145399, 31.45816453501076637 ) ) ;
#8884=ORIENTED_EDGE ( 'NONE', *, *, #36115, .T. ) ;
#8886=CARTESIAN_POINT ( 'NONE',  ( 27.24356964375000700, 197.7406250006145285, 15.72908226750537075 ) ) ;
#8887=CARTESIAN_POINT ( 'NONE',  ( 23.87821517812499650, 242.8468750006145171, -4.985214923628404904 ) ) ;
#8888=AXIS2_PLACEMENT_3D ( 'NONE', #37356, #25258, #7644 ) ;
#8892=CARTESIAN_POINT ( 'NONE',  ( 26.75643035624999655, 247.7968750006145342, 3.323476615752267715 ) ) ;
#8897=CARTESIAN_POINT ( 'NONE',  ( 15.24356964374999990, 241.1593750006145171, -3.323476615752268604 ) ) ;
#8910=CARTESIAN_POINT ( 'NONE',  ( -20.76482629054277496, 195.0000000000000000, -17.25728419020853366 ) ) ;
#8913=CARTESIAN_POINT ( 'NONE',  ( 15.00000000000000178, 247.8437500012290400, 3.464101615137757051 ) ) ;
#8915=CARTESIAN_POINT ( 'NONE',  ( 15.24356964374999990, 241.6468750006145285, 0.000000000000000000 ) ) ;
#8916=VERTEX_POINT ( 'NONE', #19427 ) ;
#8919=CARTESIAN_POINT ( 'NONE',  ( 24.00000000000000000, 243.9062500012290400, 5.196152422706629359 ) ) ;
#8922=CARTESIAN_POINT ( 'NONE',  ( -20.86978606573367045, 194.8588513912095550, -17.51182790300216752 ) ) ;
#8924=DIRECTION ( 'NONE',  ( 0.000000000000000000, 0.000000000000000000, 1.000000000000000000 ) ) ;
#8929=CARTESIAN_POINT ( 'NONE',  ( 18.12178482187499640, 249.6718750006145342, -4.985214923628404904 ) ) ;
#8935=ORIENTED_EDGE ( 'NONE', *, *, #8505, .T. ) ;
#8944=CARTESIAN_POINT ( 'NONE',  ( 23.87821517812500005, 248.9968750006145228, 4.985214923628404016 ) ) ;
#8947=EDGE_CURVE ( 'NONE', #9483, #18816, #27936, .T. ) ;
#8965=CARTESIAN_POINT ( 'NONE',  ( 0.000000000000000000, 210.0000000000000284, -27.00000000000000000 ) ) ;
#8967=CARTESIAN_POINT ( 'NONE',  ( 21.00000000000000000, 244.3468750006145171, -6.646953231504538984 ) ) ;
#8973=CARTESIAN_POINT ( 'NONE',  ( 21.00000000000000000, 245.8937500012290229, -6.928203230275506996 ) ) ;
#8976=CARTESIAN_POINT ( 'NONE',  ( 27.00000000000000355, 198.0875000012290457, -3.306546357697854128E-15 ) ) ;
#8981=ORIENTED_EDGE ( 'NONE', *, *, #2452, .T. ) ;
#8983=CARTESIAN_POINT ( 'NONE',  ( 20.99999999999999645, 241.6187500012290457, 5.999999999999998224 ) ) ;
#8984=CARTESIAN_POINT ( 'NONE',  ( 26.75643035624999655, 246.8593750006145342, -3.323476615752271712 ) ) ;
#8997=CARTESIAN_POINT ( 'NONE',  ( -27.24356964375000345, 194.8531250006145115, 0.000000000000000000 ) ) ;
#9005=DIRECTION ( 'NONE',  ( 0.000000000000000000, 0.000000000000000000, 1.000000000000000000 ) ) ;
#9009=CARTESIAN_POINT ( 'NONE',  ( 0.000000000000000000, 210.0000000000000284, -27.00000000000000000 ) ) ;
#9013=CARTESIAN_POINT ( 'NONE',  ( -26.99999999999998934, 195.0875000000000341, 15.58845726811991561 ) ) ;
#9016=CARTESIAN_POINT ( 'NONE',  ( 26.75643035624999655, 246.4843750006145342, -7.049594010296217766E-16 ) ) ;
#9017=ORIENTED_EDGE ( 'NONE', *, *, #6091, .T. ) ;
#9023=CARTESIAN_POINT ( 'NONE',  ( 15.00000000000000000, 240.0625000000000000, -3.464101615137752166 ) ) ;
#9031=CARTESIAN_POINT ( 'NONE',  ( 20.99999999999999645, 185.0294372515228645, 0.000000000000000000 ) ) ;
#9032=CARTESIAN_POINT ( 'NONE',  ( 26.99999999999999645, 242.9874999999999829, 3.464101615137751278 ) ) ;
#9035=ADVANCED_FACE ( 'NONE', ( #25647 ), #16944, .F. ) ;
#9036=CARTESIAN_POINT ( 'NONE',  ( 26.99999999999999645, 249.3249999999999886, -7.347880794884117764E-16 ) ) ;
#9037=CARTESIAN_POINT ( 'NONE',  ( 23.87821517812500005, 240.5593750006145228, 4.985214923628404016 ) ) ;
#9039=FACE_OUTER_BOUND ( 'NONE', #33452, .T. ) ;
#9045=CARTESIAN_POINT ( 'NONE',  ( 22.97035613655870989, 195.0000000000000568, 14.56992986484456587 ) ) ;
#9046=CARTESIAN_POINT ( 'NONE',  ( 27.24356964374999635, 196.9718750006145456, -15.72908226750539029 ) ) ;
#9053=CARTESIAN_POINT ( 'NONE',  ( 27.00000000000001421, 198.8374999999999773, 15.58845726811988897 ) ) ;
#9060=CARTESIAN_POINT ( 'NONE',  ( 18.00000000000000355, 249.6250000000000000, 5.196152422706632912 ) ) ;
#9061=CARTESIAN_POINT ( 'NONE',  ( 26.99999999999999645, 245.7624999999999886, -3.464101615137755275 ) ) ;
#9065=VERTEX_POINT ( 'NONE', #16576 ) ;
#9068=DIRECTION ( 'NONE',  ( -0.000000000000000000, 1.000000000000000000, -0.000000000000000000 ) ) ;
#9072=CARTESIAN_POINT ( 'NONE',  ( 26.99999999999999645, 247.9749999999999943, -7.347880794884117764E-16 ) ) ;
#9073=CARTESIAN_POINT ( 'NONE',  ( 13.62178482187499640, 199.6531250006145228, -23.59362340125807123 ) ) ;
#9077=ORIENTED_EDGE ( 'NONE', *, *, #11409, .F. ) ;
#9079=CARTESIAN_POINT ( 'NONE',  ( 13.62178482187499640, 196.5031250006145456, -23.59362340125807123 ) ) ;
#9080=CARTESIAN_POINT ( 'NONE',  ( 23.87821517812500005, 241.7968750006145342, 4.985214923628404016 ) ) ;
#9083=CARTESIAN_POINT ( 'NONE',  ( 26.75643035624999655, 248.6968750006145115, 3.323476615752267715 ) ) ;
#9089=CARTESIAN_POINT ( 'NONE',  ( 26.75643035624999655, 241.3843750006145115, 3.323476615752267271 ) ) ;
#9091=CARTESIAN_POINT ( 'NONE',  ( 26.99999999999999645, 246.6437500012290513, 3.464101615137751278 ) ) ;
#9099=DIRECTION ( 'NONE',  ( -0.8660254037844613562, -0.4999999999999605871, 0.000000000000000000 ) ) ;
#9100=CARTESIAN_POINT ( 'NONE',  ( 26.99999999999999645, 244.4687500012290684, -3.464101615137755275 ) ) ;
#9106=CARTESIAN_POINT ( 'NONE',  ( 26.75643035624999655, 242.3593750006145342, -3.323476615752271712 ) ) ;
#9113=CARTESIAN_POINT ( 'NONE',  ( 20.99999999999995381, 241.5625000000000000, 5.999999999999998224 ) ) ;
#9116=CARTESIAN_POINT ( 'NONE',  ( 20.99999999999997868, 246.0625000000000284, 5.999999999999999112 ) ) ;
#9121=CARTESIAN_POINT ( 'NONE',  ( 21.00000000000000000, 240.2687500012290513, 6.928203230275506996 ) ) ;
#9125=ADVANCED_FACE ( 'NONE', ( #22078 ), #8039, .T. ) ;
#9126=CARTESIAN_POINT ( 'NONE',  ( 23.99999999999999645, 248.0499999999999829, -5.196152422706631135 ) ) ;
#9127=ORIENTED_EDGE ( 'NONE', *, *, #34611, .T. ) ;
#9129=ORIENTED_EDGE ( 'NONE', *, *, #1321, .F. ) ;
#9135=CARTESIAN_POINT ( 'NONE',  ( 18.00000000000000000, 245.4812500012290570, -5.196152422706630247 ) ) ;
#9136=CARTESIAN_POINT ( 'NONE',  ( -26.30981681325194899, 195.0000000000000853, -6.417592593584456218 ) ) ;
#9140=EDGE_LOOP ( 'NONE', ( #29627, #25716, #26194, #20810 ) ) ;
#9141=CARTESIAN_POINT ( 'NONE',  ( 26.99999999999999645, 241.6937500012290343, 3.464101615137751278 ) ) ;
#9156=CARTESIAN_POINT ( 'NONE',  ( 26.75643035624999655, 245.5468750006145342, 3.323476615752267715 ) ) ;
#9158=CARTESIAN_POINT ( 'NONE',  ( 23.87821517812500005, 240.1093750006145342, 4.985214923628404016 ) ) ;
#9161=CARTESIAN_POINT ( 'NONE',  ( 18.00000000000000355, 247.4312500012290457, 5.196152422706632912 ) ) ;
#9163=EDGE_CURVE ( 'NONE', #16244, #17027, #5735, .T. ) ;
#9173=CARTESIAN_POINT ( 'NONE',  ( 15.24356964375000167, 246.6343750006145115, 3.323476615752272600 ) ) ;
#9194=DIRECTION ( 'NONE',  ( -0.000000000000000000, 1.000000000000000000, -0.000000000000000000 ) ) ;
#9196=CARTESIAN_POINT ( 'NONE',  ( 26.99999999999999645, 247.0937500012290400, 3.464101615137751278 ) ) ;
#9197=EDGE_CURVE ( 'NONE', #8211, #13498, #33794, .T. ) ;
#9204=CARTESIAN_POINT ( 'NONE',  ( 15.24356964375000167, 246.7468750006145797, 3.323476615752272600 ) ) ;
#9207=CARTESIAN_POINT ( 'NONE',  ( 19.39230484541326760, 245.1986538117967029, 5.999999999999999112 ) ) ;
#9211=CARTESIAN_POINT ( 'NONE',  ( 26.99999999999999645, 241.2624999999999886, -3.464101615137755275 ) ) ;
#9215=ORIENTED_EDGE ( 'NONE', *, *, #12423, .T. ) ;
#9222=CARTESIAN_POINT ( 'NONE',  ( 21.00000000000000000, 240.2968750006145342, -6.646953231504538984 ) ) ;
#9231=CARTESIAN_POINT ( 'NONE',  ( -13.62178482187498396, 196.7843750006145456, 23.59362340125808188 ) ) ;
#9235=ORIENTED_EDGE ( 'NONE', *, *, #33533, .F. ) ;
#9238=CARTESIAN_POINT ( 'NONE',  ( 23.99999999999999645, 245.4062500012290400, -5.196152422706631135 ) ) ;
#9239=CIRCLE ( 'NONE', #36471, 5.999999999999999112 ) ;
#9247=CARTESIAN_POINT ( 'NONE',  ( 20.99999999999999289, 245.8374999999999773, -5.999999999999997335 ) ) ;
#9248=ADVANCED_FACE ( 'NONE', ( #32079 ), #3081, .F. ) ;
#9250=CARTESIAN_POINT ( 'NONE',  ( 7.234628195640322446, 199.3450961906613657, 26.99999999999999645 ) ) ;
#9260=CARTESIAN_POINT ( 'NONE',  ( 15.00000000000000000, 249.5125000000000171, -3.464101615137752166 ) ) ;
#9261=CARTESIAN_POINT ( 'NONE',  ( 27.24356964375000700, 196.3906250006145342, 15.72908226750537075 ) ) ;
#9266=CARTESIAN_POINT ( 'NONE',  ( 5.778771075727756162E-15, 196.3156250006145171, 31.45816453501075927 ) ) ;
#9269=CIRCLE ( 'NONE', #7434, 2.649999999999990585 ) ;
#9271=CARTESIAN_POINT ( 'NONE',  ( 21.00000000000000000, 246.8218750006145399, 6.646953231504538984 ) ) ;
#9278=CARTESIAN_POINT ( 'NONE',  ( 15.24356964374999990, 241.6468750006145285, 0.000000000000000000 ) ) ;
#9297=CARTESIAN_POINT ( 'NONE',  ( 15.24356964374999990, 241.1968750006145115, 0.000000000000000000 ) ) ;
#9298=VERTEX_POINT ( 'NONE', #15028 ) ;
#9301=CARTESIAN_POINT ( 'NONE',  ( 27.24356964374999279, 199.6718750006145058, -15.72908226750539207 ) ) ;
#9302=DIRECTION ( 'NONE',  ( 0.000000000000000000, 0.000000000000000000, 1.000000000000000000 ) ) ;
#9303=CARTESIAN_POINT ( 'NONE',  ( 20.99999999999999645, 185.0294372515228645, -5.999999999999999112 ) ) ;
#9308=EDGE_LOOP ( 'NONE', ( #29771, #19654, #22675, #36227 ) ) ;
#9310=CARTESIAN_POINT ( 'NONE',  ( 21.00000000000000000, 246.7093750006145285, 6.646953231504538984 ) ) ;
#9315=CARTESIAN_POINT ( 'NONE',  ( 22.60769515458672885, 247.8825961894323484, 5.999999999999997335 ) ) ;
#9316=EDGE_LOOP ( 'NONE', ( #2845, #1422, #28655, #10247 ) ) ;
#9322=CARTESIAN_POINT ( 'NONE',  ( 19.39230484541324984, 245.6486538117966916, 5.999999999999991118 ) ) ;
#9323=CARTESIAN_POINT ( 'NONE',  ( -13.50000000000000533, 199.1375000012290286, -23.38268590217984411 ) ) ;
#9328=CARTESIAN_POINT ( 'NONE',  ( 19.39230484541326405, 248.7424038105677084, 5.999999999999995559 ) ) ;
#9331=( BOUNDED_CURVE ( )  B_SPLINE_CURVE ( 2, ( #36839, #21712, #33262, #22085, #19254 ),
 .UNSPECIFIED., .F., .F. ) 
 B_SPLINE_CURVE_WITH_KNOTS ( ( 3, 2, 3 ),
 ( 0.000000000000000000, 0.007246376811594202987, 0.01086956521739129364 ),
 .UNSPECIFIED. ) 
 CURVE ( )  GEOMETRIC_REPRESENTATION_ITEM ( )  RATIONAL_B_SPLINE_CURVE ( ( 1.000000000000000000, 0.8660254037844387076, 1.000000000000000000, 0.9330127018922196314, 0.9330127018922194093 ) ) 
 REPRESENTATION_ITEM ( '' )  );
#9341=CARTESIAN_POINT ( 'NONE',  ( 15.00000000000000000, 242.3125000000000000, -3.464101615137752610 ) ) ;
#9347=CARTESIAN_POINT ( 'NONE',  ( 23.87821517812499650, 242.5093750006145399, -4.985214923628404904 ) ) ;
#9349=CARTESIAN_POINT ( 'NONE',  ( 26.75643035624999655, 240.1468750006145569, 3.323476615752267271 ) ) ;
#9351=CARTESIAN_POINT ( 'NONE',  ( 23.99999999999999645, 245.4062500012290400, -5.196152422706631135 ) ) ;
#9354=LINE ( 'NONE', #6507, #22153 ) ;
#9362=CARTESIAN_POINT ( 'NONE',  ( 21.00000000000000000, 245.5843750006145569, -6.646953231504538984 ) ) ;
#9366=CARTESIAN_POINT ( 'NONE',  ( 20.21461154673354699, 212.0943692086927399, -5.961323472698028425 ) ) ;
#9377=LINE ( 'NONE', #3683, #25906 ) ;
#9391=CARTESIAN_POINT ( 'NONE',  ( 9.000000000000003553, 242.0000000000000000, 6.000000000000000888 ) ) ;
#9393=CARTESIAN_POINT ( 'NONE',  ( 20.99999999999999645, 247.4968750006145513, -6.646953231504538984 ) ) ;
#9396=DIRECTION ( 'NONE',  ( 1.000000000000000000, 0.000000000000000000, 0.000000000000000000 ) ) ;
#9397=CARTESIAN_POINT ( 'NONE',  ( 0.000000000000000000, 195.0000000000000000, 0.000000000000000000 ) ) ;
#9400=CARTESIAN_POINT ( 'NONE',  ( 15.00000000000000000, 240.9624999999999773, -3.464101615137752166 ) ) ;
#9401=CARTESIAN_POINT ( 'NONE',  ( -8.871188430189180352, 219.1704066634408434, 3.236079657462661796 ) ) ;
#9407=CARTESIAN_POINT ( 'NONE',  ( 13.49999999999999645, 195.3500000000000227, -23.38268590217984766 ) ) ;
#9412=CARTESIAN_POINT ( 'NONE',  ( 18.12178482187499640, 241.2343750006145342, -4.985214923628404904 ) ) ;
#9414=CARTESIAN_POINT ( 'NONE',  ( -5.352125845617103472, 223.7130433768494129, 2.500000000000000000 ) ) ;
#9421=CARTESIAN_POINT ( 'NONE',  ( 20.99999999999999289, 240.8874999999999886, -5.999999999999997335 ) ) ;
#9422=CARTESIAN_POINT ( 'NONE',  ( -27.24356964374999635, 198.4906250006145569, 15.72908226750539384 ) ) ;
#9433=CARTESIAN_POINT ( 'NONE',  ( 19.39230484541326049, 240.5138461906613827, -5.999999999999997335 ) ) ;
#9445=CARTESIAN_POINT ( 'NONE',  ( 15.00000000000000000, 247.7125000000000057, -3.464101615137752166 ) ) ;
#9446=CARTESIAN_POINT ( 'NONE',  ( 13.62178482187499640, 196.0531250006145285, -23.59362340125807123 ) ) ;
#9452=CARTESIAN_POINT ( 'NONE',  ( -1.926257025242585782E-15, 196.5406250006145399, -31.45816453501075927 ) ) ;
#9453=FACE_OUTER_BOUND ( 'NONE', #12945, .T. ) ;
#9456=CARTESIAN_POINT ( 'NONE',  ( 21.00000000000000000, 247.9468750006145399, -6.646953231504538984 ) ) ;
#9459=DIRECTION ( 'NONE',  ( -0.000000000000000000, -1.000000000000000000, -0.000000000000000000 ) ) ;
#9465=CARTESIAN_POINT ( 'NONE',  ( 13.49999999999999645, 198.0500000000000114, -23.38268590217984766 ) ) ;
#9477=CARTESIAN_POINT ( 'NONE',  ( 15.00000000000000000, 244.1124999999999829, -3.464101615137752610 ) ) ;
#9479=DIRECTION ( 'NONE',  ( 0.000000000000000000, 1.000000000000000000, 0.000000000000000000 ) ) ;
#9482=CARTESIAN_POINT ( 'NONE',  ( 15.24356964374999990, 242.0968750006145171, 0.000000000000000000 ) ) ;
#9483=VERTEX_POINT ( 'NONE', #32647 ) ;
#9487=CARTESIAN_POINT ( 'NONE',  ( 22.60769515458672885, 242.6674038105676345, -5.999999999999998224 ) ) ;
#9488=DIRECTION ( 'NONE',  ( -1.000000000000000000, 0.000000000000000000, 0.000000000000000000 ) ) ;
#9494=ORIENTED_EDGE ( 'NONE', *, *, #34367, .F. ) ;
#9496=CARTESIAN_POINT ( 'NONE',  ( 15.24356964374999990, 246.1468750006145285, 0.000000000000000000 ) ) ;
#9501=ADVANCED_FACE ( 'NONE', ( #13454, #19348 ), #12752, .T. ) ;
#9511=CARTESIAN_POINT ( 'NONE',  ( 20.99999999999999645, 249.1843750006145513, -6.646953231504538984 ) ) ;
#9512=VECTOR ( 'NONE', #3435, 1000.000000000000000 ) ;
#9515=FACE_OUTER_BOUND ( 'NONE', #24779, .T. ) ;
#9517=ORIENTED_EDGE ( 'NONE', *, *, #7760, .F. ) ;
#9518=( BOUNDED_CURVE ( )  B_SPLINE_CURVE ( 2, ( #34156, #8201, #19778, #28462, #31314, #20326, #34527, #23345, #5899 ),
 .UNSPECIFIED., .F., .F. ) 
 B_SPLINE_CURVE_WITH_KNOTS ( ( 3, 2, 2, 2, 3 ),
 ( 0.3369565217391304324, 0.3405797101449275499, 0.3478260869565217295, 0.3550724637681159646, 0.3586956521739130266 ),
 .UNSPECIFIED. ) 
 CURVE ( )  GEOMETRIC_REPRESENTATION_ITEM ( )  RATIONAL_B_SPLINE_CURVE ( ( 0.9330127018922194093, 0.9330127018922194093, 1.000000000000000000, 0.8660254037844387076, 1.000000000000000000, 0.8660254037844387076, 1.000000000000000000, 0.9330127018922198534, 0.9330127018922191873 ) ) 
 REPRESENTATION_ITEM ( '' )  );
#9519=CARTESIAN_POINT ( 'NONE',  ( -27.87471972953270338, 210.0000000000000284, 8.000000000000000000 ) ) ;
#9523=CARTESIAN_POINT ( 'NONE',  ( 20.99999999999997868, 246.5687500012290343, 5.999999999999999112 ) ) ;
#9537=VERTEX_POINT ( 'NONE', #18259 ) ;
#9538=VECTOR ( 'NONE', #10970, 1000.000000000000000 ) ;
#9539=CARTESIAN_POINT ( 'NONE',  ( 23.99999999999999645, 243.6062500012290286, -5.196152422706631135 ) ) ;
#9547=VERTEX_POINT ( 'NONE', #35862 ) ;
#9549=CARTESIAN_POINT ( 'NONE',  ( 26.75643035624999655, 245.0593750006144944, -3.323476615752271712 ) ) ;
#9577=CARTESIAN_POINT ( 'NONE',  ( 20.99999999999997868, 210.0000000000000000, 5.999999999999999112 ) ) ;
#9579=CARTESIAN_POINT ( 'NONE',  ( 23.87821517812500005, 245.9593750006145569, 4.985214923628404016 ) ) ;
#9589=ORIENTED_EDGE ( 'NONE', *, *, #6674, .T. ) ;
#9592=PLANE ( 'NONE',  #1284 ) ;
#9599=CARTESIAN_POINT ( 'NONE',  ( 26.99999999999999645, 243.5312500012290400, -7.347880794884117764E-16 ) ) ;
#9610=CARTESIAN_POINT ( 'NONE',  ( 13.62178482187499640, 199.2031250006145342, -23.59362340125807123 ) ) ;
#9621=CARTESIAN_POINT ( 'NONE',  ( 20.99999999999999289, 240.4937500012290457, -5.999999999999997335 ) ) ;
#9628=CARTESIAN_POINT ( 'NONE',  ( 26.99999999999999645, 244.9187500012290286, -3.464101615137755275 ) ) ;
#9631=EDGE_CURVE ( 'NONE', #13240, #19996, #21157, .T. ) ;
#9634=CARTESIAN_POINT ( 'NONE',  ( 24.00000000000000000, 247.0000000000000000, 5.196152422706629359 ) ) ;
#9635=CARTESIAN_POINT ( 'NONE',  ( -1.926257025242585782E-15, 196.0906250006145228, -31.45816453501076637 ) ) ;
#9640=CARTESIAN_POINT ( 'NONE',  ( -27.24356964374999635, 195.7906250006145115, 15.72908226750539384 ) ) ;
#9642=EDGE_CURVE ( 'NONE', #36568, #2166, #21911, .T. ) ;
#9645=CARTESIAN_POINT ( 'NONE',  ( 15.24356964374999990, 245.7718750006145001, -3.323476615752268604 ) ) ;
#9648=CARTESIAN_POINT ( 'NONE',  ( 26.99999999999999645, 243.0812500012290513, -7.347880794884117764E-16 ) ) ;
#9652=CARTESIAN_POINT ( 'NONE',  ( 20.99999999999999645, 239.9593750006145001, 6.646953231504538984 ) ) ;
#9663=DIRECTION ( 'NONE',  ( 0.000000000000000000, -0.000000000000000000, 1.000000000000000000 ) ) ;
#9669=CARTESIAN_POINT ( 'NONE',  ( 18.12178482187499640, 240.2218750006145171, -4.985214923628404904 ) ) ;
#9683=CARTESIAN_POINT ( 'NONE',  ( 26.75643035624999655, 248.1343750006145115, 3.323476615752267715 ) ) ;
#9691=EDGE_CURVE ( 'NONE', #717, #9547, #12232, .T. ) ;
#9697=CARTESIAN_POINT ( 'NONE',  ( 20.99999999999999645, 246.7093750006145285, 6.646953231504538984 ) ) ;
#9704=CARTESIAN_POINT ( 'NONE',  ( -28.62304584722514988, 203.4962709778747580, 4.665718542665365121 ) ) ;
#9711=ADVANCED_FACE ( 'NONE', ( #23426 ), #20592, .F. ) ;
#9715=ORIENTED_EDGE ( 'NONE', *, *, #34029, .F. ) ;
#9723=CARTESIAN_POINT ( 'NONE',  ( 13.50000000000001421, 195.6500000000000057, 23.38268590217984055 ) ) ;
#9731=CARTESIAN_POINT ( 'NONE',  ( 23.99999999999999645, 243.1562500012290400, -5.196152422706631135 ) ) ;
#9740=CARTESIAN_POINT ( 'NONE',  ( 15.24356964374999990, 244.3093750006145228, -3.323476615752268604 ) ) ;
#9765=CARTESIAN_POINT ( 'NONE',  ( 23.87821517812499650, 244.7593750006145399, -4.985214923628404904 ) ) ;
#9766=ORIENTED_EDGE ( 'NONE', *, *, #18960, .F. ) ;
#9771=CARTESIAN_POINT ( 'NONE',  ( -6.213262668644736308, 222.0587753200859424, 2.499999999999998668 ) ) ;
#9776=CARTESIAN_POINT ( 'NONE',  ( 13.49999999999999645, 196.8125000012290400, -23.38268590217984766 ) ) ;
#9779=( BOUNDED_CURVE ( )  B_SPLINE_CURVE ( 2, ( #29943, #23890, #27102, #1126, #35807, #10032, #36178, #21612, #9850 ),
 .UNSPECIFIED., .F., .F. ) 
 B_SPLINE_CURVE_WITH_KNOTS ( ( 3, 2, 2, 2, 3 ),
 ( 0.1195652173913043653, 0.1231884057971014551, 0.1304347826086956486, 0.1376811594202898559, 0.1413043478260869457 ),
 .UNSPECIFIED. ) 
 CURVE ( )  GEOMETRIC_REPRESENTATION_ITEM ( )  RATIONAL_B_SPLINE_CURVE ( ( 0.9330127018922194093, 0.9330127018922196314, 1.000000000000000000, 0.8660254037844387076, 1.000000000000000000, 0.8660254037844387076, 1.000000000000000000, 0.9330127018922196314, 0.9330127018922194093 ) ) 
 REPRESENTATION_ITEM ( '' )  );
#9784=DIRECTION ( 'NONE',  ( 1.000000000000000000, 0.000000000000000000, 0.000000000000000000 ) ) ;
#9785=CARTESIAN_POINT ( 'NONE',  ( 14.62176384544827101, 216.3782361545538606, 2.408991313804690115 ) ) ;
#9793=CARTESIAN_POINT ( 'NONE',  ( 5.778771075727756162E-15, 198.1156250006145285, 31.45816453501075927 ) ) ;
#9796=ORIENTED_EDGE ( 'NONE', *, *, #14549, .T. ) ;
#9811=CARTESIAN_POINT ( 'NONE',  ( 27.00000000000000355, 199.3249999999999886, -3.306546357697854128E-15 ) ) ;
#9816=DIRECTION ( 'NONE',  ( -0.000000000000000000, 1.000000000000000000, -0.000000000000000000 ) ) ;
#9819=CARTESIAN_POINT ( 'NONE',  ( 15.00000000000000178, 245.5375000000000227, 3.464101615137757051 ) ) ;
#9820=CARTESIAN_POINT ( 'NONE',  ( -13.62178482187498396, 196.2781250006145228, 23.59362340125808188 ) ) ;
#9825=CARTESIAN_POINT ( 'NONE',  ( -27.24356964374999635, 196.2406250006145285, 15.72908226750539384 ) ) ;
#9828=( BOUNDED_CURVE ( )  B_SPLINE_CURVE ( 2, ( #24260, #15161, #26710, #741, #552, #35051, #35803, #32589, #12312 ),
 .UNSPECIFIED., .F., .F. ) 
 B_SPLINE_CURVE_WITH_KNOTS ( ( 3, 2, 2, 2, 3 ),
 ( 0.1413043478260869457, 0.1449275362318840632, 0.1521739130434782705, 0.1594202898550724501, 0.1630434782608695676 ),
 .UNSPECIFIED. ) 
 CURVE ( )  GEOMETRIC_REPRESENTATION_ITEM ( )  RATIONAL_B_SPLINE_CURVE ( ( 0.9330127018922194093, 0.9330127018922190762, 1.000000000000000000, 0.8660254037844387076, 1.000000000000000000, 0.8660254037844387076, 1.000000000000000000, 0.9330127018922190762, 0.9330127018922194093 ) ) 
 REPRESENTATION_ITEM ( '' )  );
#9830=CARTESIAN_POINT ( 'NONE',  ( 15.24356964374999990, 245.3218750006145399, -3.323476615752268604 ) ) ;
#9832=CARTESIAN_POINT ( 'NONE',  ( 24.00000000000000000, 243.0062500012290627, 5.196152422706629359 ) ) ;
#9837=CARTESIAN_POINT ( 'NONE',  ( 26.75643035624999655, 240.0343750006145740, 3.323476615752267271 ) ) ;
#9842=SHAPE_REPRESENTATION ( 'head', ( #17215 ), #29865 ) ;
#9850=CARTESIAN_POINT ( 'NONE',  ( 20.99999999999998579, 248.1437500012290229, -5.999999999999997335 ) ) ;
#9852=CARTESIAN_POINT ( 'NONE',  ( -29.00000000000002487, 210.0000000000000000, -8.000000000000000000 ) ) ;
#9853=CARTESIAN_POINT ( 'NONE',  ( 18.12178482187499640, 248.8843750006145399, -4.985214923628404904 ) ) ;
#9854=ORIENTED_EDGE ( 'NONE', *, *, #36329, .T. ) ;
#9860=AXIS2_PLACEMENT_3D ( 'NONE', #12838, #30658, #1083 ) ;
#9866=CARTESIAN_POINT ( 'NONE',  ( 18.12178482187500350, 247.5718750006145115, 4.985214923628407568 ) ) ;
#9871=PLANE ( 'NONE',  #8737 ) ;
#9872=EDGE_LOOP ( 'NONE', ( #36579, #32194, #28361, #31587 ) ) ;
#9878=AXIS2_PLACEMENT_3D ( 'NONE', #13817, #25364, #37468 ) ;
#9881=CARTESIAN_POINT ( 'NONE',  ( 15.24356964375000167, 247.0843750006145285, 3.323476615752272600 ) ) ;
#9884=CARTESIAN_POINT ( 'NONE',  ( 19.39230484541324984, 246.0424038105676630, 5.999999999999991118 ) ) ;
#9900=CARTESIAN_POINT ( 'NONE',  ( 15.00000000000000178, 246.9437500012290343, 3.464101615137757051 ) ) ;
#9901=CARTESIAN_POINT ( 'NONE',  ( -13.50000000000000533, 195.8750000000000284, -23.38268590217984411 ) ) ;
#9908=CARTESIAN_POINT ( 'NONE',  ( 26.99999999999999645, 243.5312500012290400, -7.347880794884117764E-16 ) ) ;
#9914=VECTOR ( 'NONE', #27338, 1000.000000000000000 ) ;
#9917=CARTESIAN_POINT ( 'NONE',  ( 15.24356964375000167, 244.3843750006145115, 3.323476615752272600 ) ) ;
#9932=CARTESIAN_POINT ( 'NONE',  ( 13.50000000000001421, 199.7000000000000171, 23.38268590217984055 ) ) ;
#9937=DIRECTION ( 'NONE',  ( -4.130293990420971855E-17, 1.000000000000000000, 0.000000000000000000 ) ) ;
#9938=ORIENTED_EDGE ( 'NONE', *, *, #21739, .T. ) ;
#9946=CARTESIAN_POINT ( 'NONE',  ( 26.75643035624999655, 249.1843750006145228, -7.049594010296217766E-16 ) ) ;
#9948=CARTESIAN_POINT ( 'NONE',  ( 26.75643035624999655, 244.6468750006145285, 3.323476615752267271 ) ) ;
#9959=ORIENTED_EDGE ( 'NONE', *, *, #32027, .F. ) ;
#9969=CARTESIAN_POINT ( 'NONE',  ( 18.00000000000000355, 243.8312500012290513, 5.196152422706632912 ) ) ;
#9971=CARTESIAN_POINT ( 'NONE',  ( 19.39230484541324628, 245.4075961894322973, -5.999999999999989342 ) ) ;
#9978=CARTESIAN_POINT ( 'NONE',  ( -27.24356964374999990, 199.3156250006145171, -15.72908226750537786 ) ) ;
#9984=CARTESIAN_POINT ( 'NONE',  ( -7.234628195640328663, 197.8424038105676743, 26.99999999999999289 ) ) ;
#9994=CARTESIAN_POINT ( 'NONE',  ( -26.99999999999998934, 199.5874999999999773, 15.58845726811991561 ) ) ;
#10004=CARTESIAN_POINT ( 'NONE',  ( 24.00000000000000000, 246.1000000000000227, 5.196152422706629359 ) ) ;
#10005=CARTESIAN_POINT ( 'NONE',  ( 27.24356964374999279, 195.5656250006145171, -15.72908226750539207 ) ) ;
#10009=ORIENTED_EDGE ( 'NONE', *, *, #33282, .F. ) ;
#10010=CARTESIAN_POINT ( 'NONE',  ( -27.00000000000000355, 197.8625000012290513, 0.000000000000000000 ) ) ;
#10015=CARTESIAN_POINT ( 'NONE',  ( 15.24356964374999990, 245.8093750006145228, 0.000000000000000000 ) ) ;
#10021=CARTESIAN_POINT ( 'NONE',  ( 15.24356964374999990, 240.2968750006145342, 0.000000000000000000 ) ) ;
#10025=CYLINDRICAL_SURFACE ( 'NONE', #22585, 27.00000000000000000 ) ;
#10027=AXIS2_PLACEMENT_3D ( 'NONE', #1323, #28180, #3979 ) ;
#10030=CARTESIAN_POINT ( 'NONE',  ( 20.99999999999999289, 248.5937500012290400, -5.999999999999997335 ) ) ;
#10032=CARTESIAN_POINT ( 'NONE',  ( 15.00000000000000000, 248.2187500012290684, -3.464101615137752610 ) ) ;
#10033=AXIS2_PLACEMENT_3D ( 'NONE', #13186, #24741, #36291 ) ;
#10037=CARTESIAN_POINT ( 'NONE',  ( 23.87821517812500005, 239.9968750006144944, 4.985214923628404016 ) ) ;
#10038=ORIENTED_EDGE ( 'NONE', *, *, #1533, .T. ) ;
#10041=CARTESIAN_POINT ( 'NONE',  ( 20.99999999999997513, 246.7375000000000398, -5.999999999999999112 ) ) ;
#10042=( BOUNDED_SURFACE ( )  B_SPLINE_SURFACE ( 1, 2, ( 
 ( #6981, #19109, #7537, #18550, #4495, #16072, #15695, #24407, #35956, #4676, #27808, #9994, #36512, #18738, #27428, #30279, #15884, #13035, #24590, #36142, #10183, #33310, #13223, #10556, #22133, #5596, #23053, #16444, #5049, #36702, #34235, #37254, #22502, #8278, #16994, #19302, #13597, #16814, #28174, #16632, #27989, #4864, #17182, #28722, #2019, #7719, #8458, #25702, #7908, #31393, #19851, #2392, #20028, #2579, #5237, #22691, #13785, #14148, #30840, #5413, #11302, #25886, #31573, #10927, #28534, #2204, #37068, #2760, #25332, #25147, #8096, #11114, #34049, #36881, #22870, #19669, #31208, #13966, #28356, #25515, #10741, #34420, #22314, #19481, #14332, #37434, #11484, #33866, #31028, #6877, #2945, #17738, #35672, #14515, #4025, #1369, #20209, #24317, #12940, #35860, #34599, #11850, #20401, #29278, #23419, #99, #8641, #284, #34970, #31942, #9901, #7077, #15790, #17554, #4212, #18644, #9723, #21296, #31758, #32832, #5974, #29089, #30186, #33025, #18452, #3132, #987, #29994, #21485, #34785, #20583, #9013, #32127, #6164, #15597 ),
 ( #3318, #14700, #26249, #5788, #17368, #27339, #28909, #26071, #11663, #23237, #27153, #8829, #1176, #24129, #14889, #26437, #12750, #12563, #1925, #30571, #19391, #24502, #36605, #30934, #5140, #25239, #27713, #13493, #7441, #16346, #36790, #21850, #36048, #24868, #27895, #1743, #19013, #4951, #13309, #10459, #19203, #36416, #22037, #21663, #25051, #7256, #36233, #10645, #33588, #33402, #28268, #13691, #33775, #30376, #7628, #22223, #4398, #16533, #2300, #10093, #10833, #33216, #22408, #18830, #30750, #10275, #4773, #7815, #27529, #15979, #28080, #2113, #4588, #33956, #7998, #16721, #16164, #31122, #19570, #1554, #13126, #24680, #9, #11205, #22778, #34883, #11765, #25978, #34326, #17275, #34692, #3041, #14060, #37341, #17091, #14242, #28630, #37165, #19763, #31301, #14611, #5883, #5329, #26163, #8372, #22964, #2667, #36978, #8188, #25792, #25425, #25608, #16905, #19943, #32036, #23150, #23331, #29187, #22595, #31482, #28446, #2851, #11391, #2484, #17462, #13876, #5507, #14424, #34141, #197, #34511, #8551, #17652, #20118, #8922 ) ),
 .UNSPECIFIED., .F., .F., .F. ) 
 B_SPLINE_SURFACE_WITH_KNOTS ( ( 2, 2 ),
 ( 3, 2, 2, 2, 2, 2, 2, 2, 2, 2, 2, 2, 2, 2, 2, 2, 2, 2, 2, 2, 2, 2, 2, 2, 2, 2, 2, 2, 2, 2, 2, 2, 2, 2, 2, 2, 2, 2, 2, 2, 2, 2, 2, 2, 2, 2, 2, 2, 2, 2, 2, 2, 2, 2, 2, 2, 2, 2, 2, 2, 2, 2, 2, 2, 2, 2, 2, 3 ),
 ( 0.000000000000000000, 1.000000000000000000 ),
 ( 0.000000000000000000, 0.01388888888888888812, 0.02777777777777777624, 0.04166666666666666435, 0.05555555555555555247, 0.06944444444444444753, 0.08333333333333332871, 0.09722222222222222376, 0.1111111111111111049, 0.1250000000000000000, 0.1388888888888888951, 0.1527777777777777901, 0.1666666666666666574, 0.1805555555555555525, 0.1944444444444444475, 0.2083333333333333426, 0.2222222222222222099, 0.2361111111111111049, 0.2500000000000000000, 0.2638888888888888951, 0.2777777777777777901, 0.2916666666666666852, 0.3055555555555555802, 0.3194444444444444198, 0.3333333333333333148, 0.3472222222222222099, 0.3611111111111111049, 0.3750000000000000000, 0.3888888888888888951, 0.4027777777777777901, 0.4166666666666666852, 0.4305555555555555802, 0.4444444444444444198, 0.4583333333333333148, 0.4722222222222222099, 0.4861111111111111049, 0.5000000000000000000, 0.5138888888888888395, 0.5277777777777777901, 0.5416666666666666297, 0.5555555555555555802, 0.5694444444444444198, 0.5833333333333333703, 0.5972222222222222099, 0.6111111111111111605, 0.6250000000000000000, 0.6388888888888888395, 0.6527777777777777901, 0.6666666666666666297, 0.6805555555555555802, 0.6944444444444444198, 0.7083333333333333703, 0.7222222222222222099, 0.7361111111111111605, 0.7500000000000000000, 0.7638888888888888395, 0.7777777777777777901, 0.7916666666666666297, 0.8055555555555555802, 0.8194444444444444198, 0.8333333333333333703, 0.8472222222222222099, 0.8611111111111111605, 0.8750000000000000000, 0.8888888888888888395, 0.9027777777777777901, 0.9166666666666666297, 0.9258785558164617235 ),
 .UNSPECIFIED. ) 
 GEOMETRIC_REPRESENTATION_ITEM ( )  RATIONAL_B_SPLINE_SURFACE ( (
 ( 1.000000000000000000, 0.8660254037844387076, 1.000000000000000000, 0.8660254037844387076, 1.000000000000000000, 0.8660254037844387076, 1.000000000000000000, 0.8660254037844387076, 1.000000000000000000, 0.8660254037844387076, 1.000000000000000000, 0.8660254037844387076, 1.000000000000000000, 0.8660254037844387076, 1.000000000000000000, 0.8660254037844387076, 1.000000000000000000, 0.8660254037844387076, 1.000000000000000000, 0.8660254037844387076, 1.000000000000000000, 0.8660254037844387076, 1.000000000000000000, 0.8660254037844387076, 1.000000000000000000, 0.8660254037844387076, 1.000000000000000000, 0.8660254037844387076, 1.000000000000000000, 0.8660254037844387076, 1.000000000000000000, 0.8660254037844387076, 1.000000000000000000, 0.8660254037844387076, 1.000000000000000000, 0.8660254037844387076, 1.000000000000000000, 0.8660254037844387076, 1.000000000000000000, 0.8660254037844387076, 1.000000000000000000, 0.8660254037844387076, 1.000000000000000000, 0.8660254037844387076, 1.000000000000000000, 0.8660254037844387076, 1.000000000000000000, 0.8660254037844387076, 1.000000000000000000, 0.8660254037844387076, 1.000000000000000000, 0.8660254037844387076, 1.000000000000000000, 0.8660254037844387076, 1.000000000000000000, 0.8660254037844387076, 1.000000000000000000, 0.8660254037844387076, 1.000000000000000000, 0.8660254037844387076, 1.000000000000000000, 0.8660254037844387076, 1.000000000000000000, 0.8660254037844387076, 1.000000000000000000, 0.8660254037844387076, 1.000000000000000000, 0.8660254037844387076, 1.000000000000000000, 0.8660254037844387076, 1.000000000000000000, 0.8660254037844387076, 1.000000000000000000, 0.8660254037844387076, 1.000000000000000000, 0.8660254037844387076, 1.000000000000000000, 0.8660254037844387076, 1.000000000000000000, 0.8660254037844387076, 1.000000000000000000, 0.8660254037844387076, 1.000000000000000000, 0.8660254037844387076, 1.000000000000000000, 0.8660254037844387076, 1.000000000000000000, 0.8660254037844387076, 1.000000000000000000, 0.8660254037844387076, 1.000000000000000000, 0.8660254037844387076, 1.000000000000000000, 0.8660254037844387076, 1.000000000000000000, 0.8660254037844387076, 1.000000000000000000, 0.8660254037844387076, 1.000000000000000000, 0.8660254037844387076, 1.000000000000000000, 0.8660254037844387076, 1.000000000000000000, 0.8660254037844387076, 1.000000000000000000, 0.8660254037844387076, 1.000000000000000000, 0.8660254037844387076, 1.000000000000000000, 0.8660254037844387076, 1.000000000000000000, 0.8660254037844387076, 1.000000000000000000, 0.8660254037844387076, 1.000000000000000000, 0.8660254037844387076, 1.000000000000000000, 0.8660254037844387076, 1.000000000000000000, 0.8660254037844387076, 1.000000000000000000, 0.8660254037844387076, 1.000000000000000000, 0.8660254037844387076, 1.000000000000000000, 0.8660254037844387076, 1.000000000000000000, 0.8660254037844387076, 1.000000000000000000, 0.8660254037844387076, 1.000000000000000000, 0.8660254037844387076, 1.000000000000000000, 0.9111405426957062126, 0.9401542251575389919),
 ( 1.000000000000000000, 0.8660254037844387076, 1.000000000000000000, 0.8660254037844387076, 1.000000000000000000, 0.8660254037844387076, 1.000000000000000000, 0.8660254037844387076, 1.000000000000000000, 0.8660254037844387076, 1.000000000000000000, 0.8660254037844387076, 1.000000000000000000, 0.8660254037844387076, 1.000000000000000000, 0.8660254037844387076, 1.000000000000000000, 0.8660254037844387076, 1.000000000000000000, 0.8660254037844387076, 1.000000000000000000, 0.8660254037844387076, 1.000000000000000000, 0.8660254037844387076, 1.000000000000000000, 0.8660254037844387076, 1.000000000000000000, 0.8660254037844387076, 1.000000000000000000, 0.8660254037844387076, 1.000000000000000000, 0.8660254037844387076, 1.000000000000000000, 0.8660254037844387076, 1.000000000000000000, 0.8660254037844387076, 1.000000000000000000, 0.8660254037844387076, 1.000000000000000000, 0.8660254037844387076, 1.000000000000000000, 0.8660254037844387076, 1.000000000000000000, 0.8660254037844387076, 1.000000000000000000, 0.8660254037844387076, 1.000000000000000000, 0.8660254037844387076, 1.000000000000000000, 0.8660254037844387076, 1.000000000000000000, 0.8660254037844387076, 1.000000000000000000, 0.8660254037844387076, 1.000000000000000000, 0.8660254037844387076, 1.000000000000000000, 0.8660254037844387076, 1.000000000000000000, 0.8660254037844387076, 1.000000000000000000, 0.8660254037844387076, 1.000000000000000000, 0.8660254037844387076, 1.000000000000000000, 0.8660254037844387076, 1.000000000000000000, 0.8660254037844387076, 1.000000000000000000, 0.8660254037844387076, 1.000000000000000000, 0.8660254037844387076, 1.000000000000000000, 0.8660254037844387076, 1.000000000000000000, 0.8660254037844387076, 1.000000000000000000, 0.8660254037844387076, 1.000000000000000000, 0.8660254037844387076, 1.000000000000000000, 0.8660254037844387076, 1.000000000000000000, 0.8660254037844387076, 1.000000000000000000, 0.8660254037844387076, 1.000000000000000000, 0.8660254037844387076, 1.000000000000000000, 0.8660254037844387076, 1.000000000000000000, 0.8660254037844387076, 1.000000000000000000, 0.8660254037844387076, 1.000000000000000000, 0.8660254037844387076, 1.000000000000000000, 0.8660254037844387076, 1.000000000000000000, 0.8660254037844387076, 1.000000000000000000, 0.8660254037844387076, 1.000000000000000000, 0.8660254037844387076, 1.000000000000000000, 0.8660254037844387076, 1.000000000000000000, 0.8660254037844387076, 1.000000000000000000, 0.8660254037844387076, 1.000000000000000000, 0.8660254037844387076, 1.000000000000000000, 0.8660254037844387076, 1.000000000000000000, 0.8660254037844387076, 1.000000000000000000, 0.8660254037844387076, 1.000000000000000000, 0.8660254037844387076, 1.000000000000000000, 0.8660254037844387076, 1.000000000000000000, 0.8660254037844387076, 1.000000000000000000, 0.8660254037844387076, 1.000000000000000000, 0.8660254037844387076, 1.000000000000000000, 0.8660254037844387076, 1.000000000000000000, 0.8660254037844387076, 1.000000000000000000, 0.9111405426957062126, 0.9401542251575389919) ) ) 
 REPRESENTATION_ITEM ( '' )  SURFACE ( )  );
#10046=CARTESIAN_POINT ( 'NONE',  ( 15.24356964374999990, 243.5593750006145228, 0.000000000000000000 ) ) ;
#10047=EDGE_CURVE ( 'NONE', #24921, #5552, #22003, .T. ) ;
#10053=CARTESIAN_POINT ( 'NONE',  ( 26.75643035624999655, 247.2343750006145058, 3.323476615752267715 ) ) ;
#10067=( BOUNDED_SURFACE ( )  B_SPLINE_SURFACE ( 1, 2, ( 
 ( #21040, #32577, #13062, #10213, #21786, #1114, #6618, #19510, #36540, #7746, #4891, #10769, #16471, #2604, #33893, #36352, #31237, #31057, #13814, #5078, #28205, #10583, #2234, #13627, #22162, #28565, #13994, #34076, #30687, #28384, #28016, #16658, #7935, #24801, #10399, #25545, #21975, #37097, #33520, #2048, #33706, #25361, #25178, #27832, #7563, #36908, #19138, #10956, #4705, #22529, #16285, #19329, #1862, #34265, #8126, #19697, #13431, #5267, #36730, #22342, #16845, #2421, #11144, #24980, #22721, #8309, #19881, #31423, #30868, #5443, #17025, #5628, #29503, #37283, #17401, #23269, #23643, #9046, #20434, #14735, #17211, #31785, #9231, #12068, #28752, #14176, #5820, #14920, #29120, #17961, #26469, #34628, #20806, #25918, #2790, #11513, #32348, #6386, #20618, #35003, #23450, #502, #31977, #11331, #25732, #26283, #34449, #32158, #317, #37463, #28941, #132, #6197, #31603, #17588, #11882, #11696, #3163, #17770, #22901, #29312, #8490, #14363, #20059, #8858, #23083, #3352, #8672, #2977, #35186, #20243, #14547, #26101, #34815, #6006 ),
 ( #18905, #21184, #4289, #18532, #7332, #15867, #24019, #10166, #15297, #6574, #879, #36125, #33291, #9978, #12822, #30263, #9610, #3544, #27228, #29691, #18335, #27410, #26850, #15107, #24574, #23829, #26658, #1442, #35748, #12450, #13018, #21559, #12638, #6964, #29883, #9422, #21742, #15487, #32724, #688, #12259, #3914, #32534, #35370, #20997, #9793, #32910, #24390, #35564, #6761, #21371, #27041, #1067, #24203, #30070, #4104, #18150, #15677, #3724, #33104, #1253, #35937, #7148, #18722, #4657, #33849, #19283, #27790, #34217, #19651, #2185, #36305, #34032, #10536, #36684, #2002, #8262, #16054, #31193, #30458, #5218, #4475, #7701, #16240, #13575, #30823, #33473, #27602, #2375, #24755, #4846, #25128, #13386, #13766, #19464, #1817, #10353, #1633, #36864, #10722, #7890, #16425, #27971, #16612, #22296, #13205, #21926, #31011, #8076, #22486, #5032, #28339, #28154, #25312, #24938, #10909, #16794, #36493, #7517, #13950, #19089, #30641, #11099, #25499, #22113, #37051, #33661, #22672, #34952, #23037, #8442, #12022, #8997, #29261, #23221 ) ),
 .UNSPECIFIED., .F., .F., .F. ) 
 B_SPLINE_SURFACE_WITH_KNOTS ( ( 2, 2 ),
 ( 3, 2, 2, 2, 2, 2, 2, 2, 2, 2, 2, 2, 2, 2, 2, 2, 2, 2, 2, 2, 2, 2, 2, 2, 2, 2, 2, 2, 2, 2, 2, 2, 2, 2, 2, 2, 2, 2, 2, 2, 2, 2, 2, 2, 2, 2, 2, 2, 2, 2, 2, 2, 2, 2, 2, 2, 2, 2, 2, 2, 2, 2, 2, 2, 2, 2, 2, 3 ),
 ( 0.000000000000000000, 1.000000000000000000 ),
 ( 0.000000000000000000, 0.01388888888888888812, 0.02777777777777777624, 0.04166666666666666435, 0.05555555555555555247, 0.06944444444444444753, 0.08333333333333332871, 0.09722222222222222376, 0.1111111111111111049, 0.1250000000000000000, 0.1388888888888888951, 0.1527777777777777901, 0.1666666666666666574, 0.1805555555555555525, 0.1944444444444444475, 0.2083333333333333426, 0.2222222222222222099, 0.2361111111111111049, 0.2500000000000000000, 0.2638888888888888951, 0.2777777777777777901, 0.2916666666666666852, 0.3055555555555555802, 0.3194444444444444198, 0.3333333333333333148, 0.3472222222222222099, 0.3611111111111111049, 0.3750000000000000000, 0.3888888888888888951, 0.4027777777777777901, 0.4166666666666666852, 0.4305555555555555802, 0.4444444444444444198, 0.4583333333333333148, 0.4722222222222222099, 0.4861111111111111049, 0.5000000000000000000, 0.5138888888888888395, 0.5277777777777777901, 0.5416666666666666297, 0.5555555555555555802, 0.5694444444444444198, 0.5833333333333333703, 0.5972222222222222099, 0.6111111111111111605, 0.6250000000000000000, 0.6388888888888888395, 0.6527777777777777901, 0.6666666666666666297, 0.6805555555555555802, 0.6944444444444444198, 0.7083333333333333703, 0.7222222222222222099, 0.7361111111111111605, 0.7500000000000000000, 0.7638888888888888395, 0.7777777777777777901, 0.7916666666666666297, 0.8055555555555555802, 0.8194444444444444198, 0.8333333333333333703, 0.8472222222222222099, 0.8611111111111111605, 0.8750000000000000000, 0.8888888888888888395, 0.9027777777777777901, 0.9166666666666666297, 0.9258785558287927486 ),
 .UNSPECIFIED. ) 
 GEOMETRIC_REPRESENTATION_ITEM ( )  RATIONAL_B_SPLINE_SURFACE ( (
 ( 1.000000000000000000, 0.8660254037844387076, 1.000000000000000000, 0.8660254037844387076, 1.000000000000000000, 0.8660254037844387076, 1.000000000000000000, 0.8660254037844387076, 1.000000000000000000, 0.8660254037844387076, 1.000000000000000000, 0.8660254037844387076, 1.000000000000000000, 0.8660254037844387076, 1.000000000000000000, 0.8660254037844387076, 1.000000000000000000, 0.8660254037844387076, 1.000000000000000000, 0.8660254037844387076, 1.000000000000000000, 0.8660254037844387076, 1.000000000000000000, 0.8660254037844387076, 1.000000000000000000, 0.8660254037844387076, 1.000000000000000000, 0.8660254037844387076, 1.000000000000000000, 0.8660254037844387076, 1.000000000000000000, 0.8660254037844387076, 1.000000000000000000, 0.8660254037844387076, 1.000000000000000000, 0.8660254037844387076, 1.000000000000000000, 0.8660254037844387076, 1.000000000000000000, 0.8660254037844387076, 1.000000000000000000, 0.8660254037844387076, 1.000000000000000000, 0.8660254037844387076, 1.000000000000000000, 0.8660254037844387076, 1.000000000000000000, 0.8660254037844387076, 1.000000000000000000, 0.8660254037844387076, 1.000000000000000000, 0.8660254037844387076, 1.000000000000000000, 0.8660254037844387076, 1.000000000000000000, 0.8660254037844387076, 1.000000000000000000, 0.8660254037844387076, 1.000000000000000000, 0.8660254037844387076, 1.000000000000000000, 0.8660254037844387076, 1.000000000000000000, 0.8660254037844387076, 1.000000000000000000, 0.8660254037844387076, 1.000000000000000000, 0.8660254037844387076, 1.000000000000000000, 0.8660254037844387076, 1.000000000000000000, 0.8660254037844387076, 1.000000000000000000, 0.8660254037844387076, 1.000000000000000000, 0.8660254037844387076, 1.000000000000000000, 0.8660254037844387076, 1.000000000000000000, 0.8660254037844387076, 1.000000000000000000, 0.8660254037844387076, 1.000000000000000000, 0.8660254037844387076, 1.000000000000000000, 0.8660254037844387076, 1.000000000000000000, 0.8660254037844387076, 1.000000000000000000, 0.8660254037844387076, 1.000000000000000000, 0.8660254037844387076, 1.000000000000000000, 0.8660254037844387076, 1.000000000000000000, 0.8660254037844387076, 1.000000000000000000, 0.8660254037844387076, 1.000000000000000000, 0.8660254037844387076, 1.000000000000000000, 0.8660254037844387076, 1.000000000000000000, 0.8660254037844387076, 1.000000000000000000, 0.8660254037844387076, 1.000000000000000000, 0.8660254037844387076, 1.000000000000000000, 0.8660254037844387076, 1.000000000000000000, 0.8660254037844387076, 1.000000000000000000, 0.8660254037844387076, 1.000000000000000000, 0.8660254037844387076, 1.000000000000000000, 0.8660254037844387076, 1.000000000000000000, 0.8660254037844387076, 1.000000000000000000, 0.8660254037844387076, 1.000000000000000000, 0.8660254037844387076, 1.000000000000000000, 0.8660254037844387076, 1.000000000000000000, 0.8660254037844387076, 1.000000000000000000, 0.8660254037844387076, 1.000000000000000000, 0.8660254037844387076, 1.000000000000000000, 0.9111405425767590271, 0.9401542252352144136),
 ( 1.000000000000000000, 0.8660254037844387076, 1.000000000000000000, 0.8660254037844387076, 1.000000000000000000, 0.8660254037844387076, 1.000000000000000000, 0.8660254037844387076, 1.000000000000000000, 0.8660254037844387076, 1.000000000000000000, 0.8660254037844387076, 1.000000000000000000, 0.8660254037844387076, 1.000000000000000000, 0.8660254037844387076, 1.000000000000000000, 0.8660254037844387076, 1.000000000000000000, 0.8660254037844387076, 1.000000000000000000, 0.8660254037844387076, 1.000000000000000000, 0.8660254037844387076, 1.000000000000000000, 0.8660254037844387076, 1.000000000000000000, 0.8660254037844387076, 1.000000000000000000, 0.8660254037844387076, 1.000000000000000000, 0.8660254037844387076, 1.000000000000000000, 0.8660254037844387076, 1.000000000000000000, 0.8660254037844387076, 1.000000000000000000, 0.8660254037844387076, 1.000000000000000000, 0.8660254037844387076, 1.000000000000000000, 0.8660254037844387076, 1.000000000000000000, 0.8660254037844387076, 1.000000000000000000, 0.8660254037844387076, 1.000000000000000000, 0.8660254037844387076, 1.000000000000000000, 0.8660254037844387076, 1.000000000000000000, 0.8660254037844387076, 1.000000000000000000, 0.8660254037844387076, 1.000000000000000000, 0.8660254037844387076, 1.000000000000000000, 0.8660254037844387076, 1.000000000000000000, 0.8660254037844387076, 1.000000000000000000, 0.8660254037844387076, 1.000000000000000000, 0.8660254037844387076, 1.000000000000000000, 0.8660254037844387076, 1.000000000000000000, 0.8660254037844387076, 1.000000000000000000, 0.8660254037844387076, 1.000000000000000000, 0.8660254037844387076, 1.000000000000000000, 0.8660254037844387076, 1.000000000000000000, 0.8660254037844387076, 1.000000000000000000, 0.8660254037844387076, 1.000000000000000000, 0.8660254037844387076, 1.000000000000000000, 0.8660254037844387076, 1.000000000000000000, 0.8660254037844387076, 1.000000000000000000, 0.8660254037844387076, 1.000000000000000000, 0.8660254037844387076, 1.000000000000000000, 0.8660254037844387076, 1.000000000000000000, 0.8660254037844387076, 1.000000000000000000, 0.8660254037844387076, 1.000000000000000000, 0.8660254037844387076, 1.000000000000000000, 0.8660254037844387076, 1.000000000000000000, 0.8660254037844387076, 1.000000000000000000, 0.8660254037844387076, 1.000000000000000000, 0.8660254037844387076, 1.000000000000000000, 0.8660254037844387076, 1.000000000000000000, 0.8660254037844387076, 1.000000000000000000, 0.8660254037844387076, 1.000000000000000000, 0.8660254037844387076, 1.000000000000000000, 0.8660254037844387076, 1.000000000000000000, 0.8660254037844387076, 1.000000000000000000, 0.8660254037844387076, 1.000000000000000000, 0.8660254037844387076, 1.000000000000000000, 0.8660254037844387076, 1.000000000000000000, 0.8660254037844387076, 1.000000000000000000, 0.8660254037844387076, 1.000000000000000000, 0.8660254037844387076, 1.000000000000000000, 0.8660254037844387076, 1.000000000000000000, 0.8660254037844387076, 1.000000000000000000, 0.9111405425767590271, 0.9401542252352144136) ) ) 
 REPRESENTATION_ITEM ( '' )  SURFACE ( )  );
#10069=CARTESIAN_POINT ( 'NONE',  ( 18.12178482187500350, 246.6718750006145342, 4.985214923628407568 ) ) ;
#10076=EDGE_CURVE ( 'NONE', #21259, #7355, #7594, .T. ) ;
#10089=DIRECTION ( 'NONE',  ( -0.000000000000000000, 1.000000000000000000, -0.000000000000000000 ) ) ;
#10092=CARTESIAN_POINT ( 'NONE',  ( 15.00000000000000178, 245.0875000000000057, 3.464101615137757051 ) ) ;
#10093=CARTESIAN_POINT ( 'NONE',  ( -27.24356964374999635, 197.6468750006145285, 15.72908226750539384 ) ) ;
#10098=CARTESIAN_POINT ( 'NONE',  ( 15.00000000000000000, 244.6187500012290172, -3.464101615137752166 ) ) ;
#10107=CARTESIAN_POINT ( 'NONE',  ( 15.24356964375000167, 243.4843750006145058, 3.323476615752272600 ) ) ;
#10131=CARTESIAN_POINT ( 'NONE',  ( -13.49999999999998401, 199.1750000000000114, 23.38268590217985476 ) ) ;
#10133=CARTESIAN_POINT ( 'NONE',  ( -26.99999999999999645, 195.5374999999999943, 15.58845726811991561 ) ) ;
#10135=FACE_OUTER_BOUND ( 'NONE', #15985, .T. ) ;
#10137=CARTESIAN_POINT ( 'NONE',  ( 20.99999999999999645, 244.7968750006145342, -6.646953231504538984 ) ) ;
#10146=ORIENTED_EDGE ( 'NONE', *, *, #31383, .F. ) ;
#10166=CARTESIAN_POINT ( 'NONE',  ( 27.24356964375000700, 199.5406250006145683, 15.72908226750537075 ) ) ;
#10183=CARTESIAN_POINT ( 'NONE',  ( 13.50000000000001421, 199.2500000000000000, 23.38268590217984055 ) ) ;
#10184=CARTESIAN_POINT ( 'NONE',  ( 1.069080835302379631E-14, 199.2125000000000057, 27.00000000000000000 ) ) ;
#10187=CARTESIAN_POINT ( 'NONE',  ( 19.39230484541326049, 241.8075961894323029, -5.999999999999997335 ) ) ;
#10189=EDGE_CURVE ( 'NONE', #34895, #24301, #8502, .T. ) ;
#10193=CARTESIAN_POINT ( 'NONE',  ( 21.00000000000000000, 244.9375000000000000, -6.928203230275506996 ) ) ;
#10194=CARTESIAN_POINT ( 'NONE',  ( -29.00000000000002487, 215.7563705986615901, -5.555555555555559799 ) ) ;
#10202=CARTESIAN_POINT ( 'NONE',  ( 13.49999999999999645, 197.7125000012290172, -23.38268590217984766 ) ) ;
#10203=CARTESIAN_POINT ( 'NONE',  ( 15.00000000000000000, 248.7062500012290229, 0.000000000000000000 ) ) ;
#10206=CARTESIAN_POINT ( 'NONE',  ( 26.75643035624999655, 245.1343750006145115, -7.049594010296217766E-16 ) ) ;
#10208=CARTESIAN_POINT ( 'NONE',  ( 23.99999999999999645, 243.1562500012290400, -5.196152422706631135 ) ) ;
#10213=CARTESIAN_POINT ( 'NONE',  ( -1.926257025242585782E-15, 199.7468750006145513, -31.45816453501075927 ) ) ;
#10227=CARTESIAN_POINT ( 'NONE',  ( 26.75643035624999655, 241.0093750006144830, -3.323476615752271712 ) ) ;
#10231=CARTESIAN_POINT ( 'NONE',  ( 5.778771075727756162E-15, 198.1718750006145342, 31.45816453501076637 ) ) ;
#10234=CARTESIAN_POINT ( 'NONE',  ( 21.00000000000000000, 242.7718750006145854, 6.646953231504538984 ) ) ;
#10239=CARTESIAN_POINT ( 'NONE',  ( 21.00000000000000000, 244.4593750006145001, 6.646953231504538984 ) ) ;
#10244=EDGE_CURVE ( 'NONE', #27444, #35917, #20090, .T. ) ;
#10247=ORIENTED_EDGE ( 'NONE', *, *, #1776, .F. ) ;
#10253=CARTESIAN_POINT ( 'NONE',  ( 26.75643035624999655, 246.8218750006145115, -7.049594010296217766E-16 ) ) ;
#10275=CARTESIAN_POINT ( 'NONE',  ( 27.24356964374999635, 197.4218750006145342, -15.72908226750539029 ) ) ;
#10281=CARTESIAN_POINT ( 'NONE',  ( 26.99999999999999645, 244.9187500012290286, -3.464101615137755275 ) ) ;
#10287=EDGE_CURVE ( 'NONE', #29663, #11836, #21908, .T. ) ;
#10288=( BOUNDED_CURVE ( )  B_SPLINE_CURVE ( 2, ( #4442, #24171, #6926, #12417, #35532, #21151, #23797, #35715, #15263 ),
 .UNSPECIFIED., .F., .F. ) 
 B_SPLINE_CURVE_WITH_KNOTS ( ( 3, 2, 2, 2, 3 ),
 ( 0.2065217391304347838, 0.2101449275362318736, 0.2173913043478260809, 0.2246376811594202882, 0.2282608695652173780 ),
 .UNSPECIFIED. ) 
 CURVE ( )  GEOMETRIC_REPRESENTATION_ITEM ( )  RATIONAL_B_SPLINE_CURVE ( ( 0.9330127018922194093, 0.9330127018922194093, 1.000000000000000000, 0.8660254037844387076, 1.000000000000000000, 0.8660254037844387076, 1.000000000000000000, 0.9330127018922196314, 0.9330127018922194093 ) ) 
 REPRESENTATION_ITEM ( '' )  );
#10301=CARTESIAN_POINT ( 'NONE',  ( -10.38983282724226065, 218.0043899860427530, -3.786144536302608277 ) ) ;
#10310=ORIENTED_EDGE ( 'NONE', *, *, #32309, .F. ) ;
#10318=CARTESIAN_POINT ( 'NONE',  ( 18.12178482187500350, 247.2343750006145342, 4.985214923628407568 ) ) ;
#10320=CARTESIAN_POINT ( 'NONE',  ( 15.24356964374999990, 243.9718750006145456, -3.323476615752268604 ) ) ;
#10322=ORIENTED_EDGE ( 'NONE', *, *, #21252, .T. ) ;
#10323=( BOUNDED_CURVE ( )  B_SPLINE_CURVE ( 2, ( #10925, #22500, #19667, #16812, #28354, #14513, #5786, #3505, #23604 ),
 .UNSPECIFIED., .F., .F. ) 
 B_SPLINE_CURVE_WITH_KNOTS ( ( 3, 2, 2, 2, 3 ),
 ( 0.07608695652173913526, 0.07971014492753622505, 0.08695652173913043237, 0.09420289855072463969, 0.09782608695652174335 ),
 .UNSPECIFIED. ) 
 CURVE ( )  GEOMETRIC_REPRESENTATION_ITEM ( )  RATIONAL_B_SPLINE_CURVE ( ( 0.9330127018922192983, 0.9330127018922194093, 1.000000000000000000, 0.8660254037844387076, 1.000000000000000000, 0.8660254037844387076, 1.000000000000000000, 0.9330127018922194093, 0.9330127018922194093 ) ) 
 REPRESENTATION_ITEM ( '' )  );
#10332=ORIENTED_EDGE ( 'NONE', *, *, #13410, .T. ) ;
#10344=FACE_OUTER_BOUND ( 'NONE', #30664, .T. ) ;
#10353=CARTESIAN_POINT ( 'NONE',  ( -27.24356964375000345, 196.2031250006145342, 0.000000000000000000 ) ) ;
#10357=EDGE_LOOP ( 'NONE', ( #31713, #31910, #5647, #27351 ) ) ;
#10361=CARTESIAN_POINT ( 'NONE',  ( 20.99999999999998579, 247.6937500012290059, -5.999999999999997335 ) ) ;
#10375=DIRECTION ( 'NONE',  ( -0.000000000000000000, -1.000000000000000000, -0.000000000000000000 ) ) ;
#10380=CARTESIAN_POINT ( 'NONE',  ( 15.00000000000000178, 246.4375000000000000, 3.464101615137757051 ) ) ;
#10381=DIRECTION ( 'NONE',  ( 0.000000000000000000, -1.000000000000000000, 0.000000000000000000 ) ) ;
#10385=VERTEX_POINT ( 'NONE', #18705 ) ;
#10386=CARTESIAN_POINT ( 'NONE',  ( 5.727106289114498080E-15, 197.5250000012290457, 31.17691453623979214 ) ) ;
#10390=CARTESIAN_POINT ( 'NONE',  ( 26.75643035624999655, 245.5843750006145285, -7.049594010296217766E-16 ) ) ;
#10399=CARTESIAN_POINT ( 'NONE',  ( -13.62178482187498396, 198.5843750006145569, 23.59362340125808188 ) ) ;
#10405=CARTESIAN_POINT ( 'NONE',  ( 0.000000000000000000, 210.0000000000000284, 0.000000000000000000 ) ) ;
#10412=CARTESIAN_POINT ( 'NONE',  ( 0.000000000000000000, 210.0000000000000284, -27.00000000000000000 ) ) ;
#10415=CARTESIAN_POINT ( 'NONE',  ( 15.24356964374999990, 239.8468750006145171, 0.000000000000000000 ) ) ;
#10419=CARTESIAN_POINT ( 'NONE',  ( 27.24356964374999279, 198.3218750006145399, -15.72908226750539207 ) ) ;
#10422=CARTESIAN_POINT ( 'NONE',  ( 26.75643035624999655, 242.0218750006145285, -3.323476615752271712 ) ) ;
#10429=CARTESIAN_POINT ( 'NONE',  ( 15.24356964374999990, 245.2468750006145228, 0.000000000000000000 ) ) ;
#10442=CARTESIAN_POINT ( 'NONE',  ( 15.24356964375000167, 245.7343750006144774, 3.323476615752272600 ) ) ;
#10446=ORIENTED_EDGE ( 'NONE', *, *, #26971, .T. ) ;
#10459=CARTESIAN_POINT ( 'NONE',  ( -1.926257025242585782E-15, 198.3968750006145285, -31.45816453501075927 ) ) ;
#10461=DIRECTION ( 'NONE',  ( 0.000000000000000000, 0.000000000000000000, 1.000000000000000000 ) ) ;
#10466=CARTESIAN_POINT ( 'NONE',  ( 21.00000000000000000, 240.9437500012290911, -6.928203230275506996 ) ) ;
#10469=CARTESIAN_POINT ( 'NONE',  ( 27.24356964375000345, 198.6781250006145569, -3.336375036156643733E-15 ) ) ;
#10477=CARTESIAN_POINT ( 'NONE',  ( -7.234628195640316228, 196.3075961894323598, -27.00000000000000000 ) ) ;
#10480=( BOUNDED_CURVE ( )  B_SPLINE_CURVE ( 2, ( #2096, #33754, #13476, #4567, #27875, #22205, #36587, #13674, #16887 ),
 .UNSPECIFIED., .F., .F. ) 
 B_SPLINE_CURVE_WITH_KNOTS ( ( 3, 2, 2, 2, 3 ),
 ( 0.3958333333333333703, 0.4027777777777777901, 0.4166666666666666852, 0.4305555555555555802, 0.4375000000000000000 ),
 .UNSPECIFIED. ) 
 CURVE ( )  GEOMETRIC_REPRESENTATION_ITEM ( )  RATIONAL_B_SPLINE_CURVE ( ( 0.9330127018922194093, 0.9330127018922196314, 1.000000000000000000, 0.8660254037844387076, 1.000000000000000000, 0.8660254037844387076, 1.000000000000000000, 0.9330127018922194093, 0.9330127018922194093 ) ) 
 REPRESENTATION_ITEM ( '' )  );
#10502=CARTESIAN_POINT ( 'NONE',  ( 18.12178482187500350, 248.5843750006145285, 4.985214923628407568 ) ) ;
#10504=CARTESIAN_POINT ( 'NONE',  ( 18.12178482187499640, 243.9343750006145513, -4.985214923628404904 ) ) ;
#10506=CARTESIAN_POINT ( 'NONE',  ( 3.253724281355069334E-15, 199.8875000000000455, -27.00000000000000000 ) ) ;
#10512=EDGE_CURVE ( 'NONE', #30621, #18936, #21310, .T. ) ;
#10515=ORIENTED_EDGE ( 'NONE', *, *, #20929, .T. ) ;
#10522=CARTESIAN_POINT ( 'NONE',  ( 23.87821517812500005, 249.4468750006145115, 4.985214923628404016 ) ) ;
#10527=ADVANCED_FACE ( 'NONE', ( #35873 ), #33042, .F. ) ;
#10528=CARTESIAN_POINT ( 'NONE',  ( 7.136082524517427750, 215.1989690533051771, -3.001545256184917854 ) ) ;
#10530=DIRECTION ( 'NONE',  ( 0.000000000000000000, 0.000000000000000000, 1.000000000000000000 ) ) ;
#10536=CARTESIAN_POINT ( 'NONE',  ( -27.24356964374999990, 197.0656250006145171, -15.72908226750537786 ) ) ;
#10550=VECTOR ( 'NONE', #10708, 1000.000000000000000 ) ;
#10556=CARTESIAN_POINT ( 'NONE',  ( -26.99999999999998934, 199.1375000000000171, 15.58845726811991561 ) ) ;
#10557=CARTESIAN_POINT ( 'NONE',  ( -29.00000000000002487, 215.7563705986615901, 5.555555555555559799 ) ) ;
#10561=VERTEX_POINT ( 'NONE', #24405 ) ;
#10565=CARTESIAN_POINT ( 'NONE',  ( 15.00000000000000178, 244.6375000000000171, 3.464101615137757051 ) ) ;
#10569=VERTEX_POINT ( 'NONE', #27244 ) ;
#10570=EDGE_LOOP ( 'NONE', ( #29914, #32232, #28673, #10009, #18077, #26451 ) ) ;
#10571=CARTESIAN_POINT ( 'NONE',  ( 5.727106289114498080E-15, 198.8750000012290400, 31.17691453623979214 ) ) ;
#10576=CARTESIAN_POINT ( 'NONE',  ( 21.00000000000000000, 242.9968750006145228, -6.646953231504538984 ) ) ;
#10580=EDGE_CURVE ( 'NONE', #3896, #33538, #9239, .T. ) ;
#10583=CARTESIAN_POINT ( 'NONE',  ( 5.778771075727756162E-15, 199.0718750006145399, 31.45816453501075927 ) ) ;
#10600=CARTESIAN_POINT ( 'NONE',  ( -1.926257025242585782E-15, 197.4968750006145513, -31.45816453501076637 ) ) ;
#10604=CARTESIAN_POINT ( 'NONE',  ( 18.12178482187500350, 243.1843750006145513, 4.985214923628407568 ) ) ;
#10605=CARTESIAN_POINT ( 'NONE',  ( 1.120210788295102201E-13, 195.3875000000000455, -27.00000000000000711 ) ) ;
#10609=VERTEX_POINT ( 'NONE', #1267 ) ;
#10612=CARTESIAN_POINT ( 'NONE',  ( 23.87821517812499650, 245.5468750006145058, -4.985214923628404904 ) ) ;
#10617=CARTESIAN_POINT ( 'NONE',  ( 24.00000000000000000, 244.2999999999999829, 5.196152422706629359 ) ) ;
#10625=CARTESIAN_POINT ( 'NONE',  ( 18.12178482187499640, 243.3718750006145228, -4.985214923628404904 ) ) ;
#10631=VECTOR ( 'NONE', #10707, 1000.000000000000000 ) ;
#10633=CARTESIAN_POINT ( 'NONE',  ( -27.00000000000000355, 199.5500000000000114, 0.000000000000000000 ) ) ;
#10635=CARTESIAN_POINT ( 'NONE',  ( 22.60769515458670753, 242.7236538117967086, -6.000000000000011546 ) ) ;
#10644=CARTESIAN_POINT ( 'NONE',  ( 21.00000000000001066, 247.0187500012290513, 5.999999999999998224 ) ) ;
#10645=CARTESIAN_POINT ( 'NONE',  ( -27.24356964374999635, 198.0968750006145456, 15.72908226750539384 ) ) ;
#10646=EDGE_CURVE ( 'NONE', #5744, #12855, #9269, .T. ) ;
#10648=CARTESIAN_POINT ( 'NONE',  ( 26.99999999999999645, 243.8875000000000171, 3.464101615137751278 ) ) ;
#10651=ORIENTED_EDGE ( 'NONE', *, *, #19461, .F. ) ;
#10652=CARTESIAN_POINT ( 'NONE',  ( 18.00000000000000000, 240.5312500012290400, -5.196152422706630247 ) ) ;
#10655=CARTESIAN_POINT ( 'NONE',  ( 27.24356964375000700, 198.1906250006145740, 15.72908226750537075 ) ) ;
#10666=CARTESIAN_POINT ( 'NONE',  ( -3.253724281355068545E-15, 196.2874999999999659, -27.00000000000000000 ) ) ;
#10675=LINE ( 'NONE', #11565, #25498 ) ;
#10679=CARTESIAN_POINT ( 'NONE',  ( 18.00000000000000000, 244.1312500012290343, -5.196152422706630247 ) ) ;
#10685=CARTESIAN_POINT ( 'NONE',  ( 21.00000000000000000, 210.0000000000000284, 8.000000000000000000 ) ) ;
#10688=CARTESIAN_POINT ( 'NONE',  ( 15.24356964374999990, 247.6093750006145342, 0.000000000000000000 ) ) ;
#10690=CARTESIAN_POINT ( 'NONE',  ( 23.87821517812500005, 240.5593750006145228, 4.985214923628404016 ) ) ;
#10694=AXIS2_PLACEMENT_3D ( 'NONE', #14970, #3213, #29740 ) ;
#10695=CARTESIAN_POINT ( 'NONE',  ( 18.00000000000000000, 249.0812500012290513, -5.196152422706630247 ) ) ;
#10699=CARTESIAN_POINT ( 'NONE',  ( 26.99999999999999645, 240.8312500012290513, -7.347880794884117764E-16 ) ) ;
#10707=DIRECTION ( 'NONE',  ( 0.000000000000000000, 1.000000000000000000, 0.000000000000000000 ) ) ;
#10708=DIRECTION ( 'NONE',  ( -0.000000000000000000, 1.000000000000000000, -0.000000000000000000 ) ) ;
#10714=CARTESIAN_POINT ( 'NONE',  ( 14.59897497552647749, 216.4010250244744498, 0.7232488345312237943 ) ) ;
#10716=AXIS2_PLACEMENT_3D ( 'NONE', #32870, #9194, #9005 ) ;
#10722=CARTESIAN_POINT ( 'NONE',  ( -1.926257025242585782E-15, 196.0906250006145228, -31.45816453501075927 ) ) ;
#10728=EDGE_CURVE ( 'NONE', #16873, #18271, #20141, .T. ) ;
#10739=CARTESIAN_POINT ( 'NONE',  ( -3.253724281355068545E-15, 198.6500000012290172, -27.00000000000000000 ) ) ;
#10741=CARTESIAN_POINT ( 'NONE',  ( 13.50000000000001421, 197.0000000000000000, 23.38268590217984055 ) ) ;
#10745=CARTESIAN_POINT ( 'NONE',  ( 15.00000000000000000, 241.8625000000000114, -3.464101615137752610 ) ) ;
#10752=CARTESIAN_POINT ( 'NONE',  ( 18.00000000000000000, 242.7249999999999943, -5.196152422706630247 ) ) ;
#10758=EDGE_LOOP ( 'NONE', ( #27822, #7183, #1445, #23423 ) ) ;
#10759=CARTESIAN_POINT ( 'NONE',  ( 26.99999999999999645, 197.2250000012290059, -15.58845726811990495 ) ) ;
#10760=DIRECTION ( 'NONE',  ( 0.000000000000000000, 0.000000000000000000, 1.000000000000000000 ) ) ;
#10764=CARTESIAN_POINT ( 'NONE',  ( 21.00000000000000000, 242.3218750006145115, 6.646953231504538984 ) ) ;
#10769=CARTESIAN_POINT ( 'NONE',  ( -27.24356964374999635, 199.4468750006145399, 15.72908226750539384 ) ) ;
#10790=CARTESIAN_POINT ( 'NONE',  ( -13.62178482187498396, 197.6843750006145228, 23.59362340125808188 ) ) ;
#10794=CARTESIAN_POINT ( 'NONE',  ( 18.00000000000000000, 239.6312500012290343, -5.196152422706630247 ) ) ;
#10795=CARTESIAN_POINT ( 'NONE',  ( 15.24356964374999990, 239.9593750006145285, 0.000000000000000000 ) ) ;
#10800=ORIENTED_EDGE ( 'NONE', *, *, #19639, .F. ) ;
#10801=CARTESIAN_POINT ( 'NONE',  ( 18.12178482187500350, 245.3218750006145115, 4.985214923628407568 ) ) ;
#10802=EDGE_CURVE ( 'NONE', #6368, #31527, #6810, .T. ) ;
#10813=ADVANCED_FACE ( 'NONE', ( #7013 ), #18773, .F. ) ;
#10815=CARTESIAN_POINT ( 'NONE',  ( 15.24356964374999990, 244.3468750006145171, 0.000000000000000000 ) ) ;
#10822=CARTESIAN_POINT ( 'NONE',  ( 19.39230484541326049, 244.5075961894323200, -5.999999999999997335 ) ) ;
#10828=ORIENTED_EDGE ( 'NONE', *, *, #6247, .T. ) ;
#10833=CARTESIAN_POINT ( 'NONE',  ( -27.24356964375000345, 197.6093750006145342, 0.000000000000000000 ) ) ;
#10834=DIRECTION ( 'NONE',  ( -1.000000000000000000, -6.123233995736766036E-17, 0.000000000000000000 ) ) ;
#10841=CARTESIAN_POINT ( 'NONE',  ( 15.00000000000000000, 241.4687500012290684, -3.464101615137752166 ) ) ;
#10846=ORIENTED_EDGE ( 'NONE', *, *, #3559, .T. ) ;
#10860=CARTESIAN_POINT ( 'NONE',  ( -9.244191109966227060, 218.8665654034646479, -3.366944586054378519 ) ) ;
#10873=CARTESIAN_POINT ( 'NONE',  ( 23.99999999999999645, 247.5999999999999943, -5.196152422706631135 ) ) ;
#10877=CARTESIAN_POINT ( 'NONE',  ( 15.24356964374999990, 248.0218750006145285, -3.323476615752268604 ) ) ;
#10879=CARTESIAN_POINT ( 'NONE',  ( 26.75643035624999655, 242.8468750006145171, 3.323476615752267271 ) ) ;
#10883=CARTESIAN_POINT ( 'NONE',  ( 26.99999999999999645, 247.6187500012290741, -3.464101615137755275 ) ) ;
#10892=ORIENTED_EDGE ( 'NONE', *, *, #10287, .F. ) ;
#10897=CARTESIAN_POINT ( 'NONE',  ( 23.87821517812500005, 248.0968750006144887, 4.985214923628404016 ) ) ;
#10900=CARTESIAN_POINT ( 'NONE',  ( 6.418300056333647419, 215.4681374788750361, 2.477503916095803227 ) ) ;
#10909=CARTESIAN_POINT ( 'NONE',  ( 27.24356964375000700, 195.4906250006145001, 15.72908226750537075 ) ) ;
#10913=CARTESIAN_POINT ( 'NONE',  ( 22.60769515458672885, 242.0888461906613713, 5.999999999999997335 ) ) ;
#10925=CARTESIAN_POINT ( 'NONE',  ( 20.99999999999999289, 249.2125000000000057, 5.999999999999999112 ) ) ;
#10927=CARTESIAN_POINT ( 'NONE',  ( -1.909035429704832693E-15, 197.6375000000000171, -31.17691453623979214 ) ) ;
#10931=CARTESIAN_POINT ( 'NONE',  ( 20.99999999999999645, 249.5218750006145285, 6.646953231504538984 ) ) ;
#10939=( BOUNDED_CURVE ( )  B_SPLINE_CURVE ( 2, ( #19333, #7939, #2609, #19515, #22907, #31061, #5271, #13818, #5085 ),
 .UNSPECIFIED., .F., .F. ) 
 B_SPLINE_CURVE_WITH_KNOTS ( ( 3, 2, 2, 2, 3 ),
 ( 0.4456521739130434590, 0.4492753623188405765, 0.4565217391304347561, 0.4637681159420289911, 0.4673913043478261087 ),
 .UNSPECIFIED. ) 
 CURVE ( )  GEOMETRIC_REPRESENTATION_ITEM ( )  RATIONAL_B_SPLINE_CURVE ( ( 0.9330127018922191873, 0.9330127018922187432, 1.000000000000000000, 0.8660254037844387076, 1.000000000000000000, 0.8660254037844387076, 1.000000000000000000, 0.9330127018922188542, 0.9330127018922194093 ) ) 
 REPRESENTATION_ITEM ( '' )  );
#10940=CARTESIAN_POINT ( 'NONE',  ( 23.99999999999999645, 244.4499999999999886, -5.196152422706631135 ) ) ;
#10943=VERTEX_POINT ( 'NONE', #18953 ) ;
#10945=CARTESIAN_POINT ( 'NONE',  ( -13.50000000000000533, 195.9875000012290229, -23.38268590217984411 ) ) ;
#10949=CARTESIAN_POINT ( 'NONE',  ( 26.75643035624999655, 242.9218750006145626, -3.323476615752271712 ) ) ;
#10954=( BOUNDED_CURVE ( )  B_SPLINE_CURVE ( 2, ( #28430, #20293, #14043, #17259, #28800, #2836, #14408, #8129, #11560 ),
 .UNSPECIFIED., .F., .F. ) 
 B_SPLINE_CURVE_WITH_KNOTS ( ( 3, 2, 2, 2, 3 ),
 ( 0.9239130434782608647, 0.9275362318840579823, 0.9347826086956522174, 0.9420289855072463414, 0.9456521739130434590 ),
 .UNSPECIFIED. ) 
 CURVE ( )  GEOMETRIC_REPRESENTATION_ITEM ( )  RATIONAL_B_SPLINE_CURVE ( ( 0.9330127018922194093, 0.9330127018922194093, 1.000000000000000000, 0.8660254037844387076, 1.000000000000000000, 0.8660254037844387076, 1.000000000000000000, 0.9330127018922194093, 0.9330127018922194093 ) ) 
 REPRESENTATION_ITEM ( '' )  );
#10956=CARTESIAN_POINT ( 'NONE',  ( -27.24356964374999635, 198.0968750006145456, 15.72908226750539384 ) ) ;
#10965=CARTESIAN_POINT ( 'NONE',  ( 26.99999999999999645, 247.1312500012290343, -7.347880794884117764E-16 ) ) ;
#10969=CARTESIAN_POINT ( 'NONE',  ( 17.54540804174073187, 195.0000000000000000, -20.52215039046394907 ) ) ;
#10970=DIRECTION ( 'NONE',  ( -0.000000000000000000, -1.000000000000000000, -0.000000000000000000 ) ) ;
#10971=CIRCLE ( 'NONE', #29111, 5.999999999999999112 ) ;
#10973=CIRCLE ( 'NONE', #30352, 27.00000000000000000 ) ;
#10976=CARTESIAN_POINT ( 'NONE',  ( -27.24356964375000345, 198.4718750006145171, -15.72908226750537786 ) ) ;
#10979=CARTESIAN_POINT ( 'NONE',  ( 15.00000000000000000, 239.6687500012290570, -3.464101615137752610 ) ) ;
#10980=CARTESIAN_POINT ( 'NONE',  ( 18.12178482187500350, 240.0343750006145171, 4.985214923628407568 ) ) ;
#10981=DIRECTION ( 'NONE',  ( 0.000000000000000000, 0.000000000000000000, 1.000000000000000000 ) ) ;
#10986=CARTESIAN_POINT ( 'NONE',  ( 15.24356964374999990, 243.8593750006145342, -3.323476615752268604 ) ) ;
#10995=AXIS2_PLACEMENT_3D ( 'NONE', #26958, #989, #22181 ) ;
#10999=CARTESIAN_POINT ( 'NONE',  ( 20.99999999999999645, 244.4593750006145285, 6.646953231504538984 ) ) ;
#11001=CARTESIAN_POINT ( 'NONE',  ( 23.99999999999999645, 240.4000000000000057, -5.196152422706631135 ) ) ;
#11010=CARTESIAN_POINT ( 'NONE',  ( 20.99999999999995026, 242.7437500012290741, -5.999999999999998224 ) ) ;
#11013=CARTESIAN_POINT ( 'NONE',  ( 20.99999999999997513, 245.8937500012290798, -5.999999999999999112 ) ) ;
#11017=VECTOR ( 'NONE', #35577, 1000.000000000000000 ) ;
#11023=CARTESIAN_POINT ( 'NONE',  ( 2.999999999999997335, 244.5000000000000000, 2.500000000000000000 ) ) ;
#11026=ORIENTED_EDGE ( 'NONE', *, *, #5250, .F. ) ;
#11027=CARTESIAN_POINT ( 'NONE',  ( 15.00000000000000178, 241.0937500012290116, 3.464101615137757051 ) ) ;
#11032=B_SPLINE_CURVE_WITH_KNOTS ( 'NONE', 3,
 ( #19681, #29670, #32137, #18316, #20783, #23807, #9401, #6940, #4082, #35163, #9771, #3518 ),
 .UNSPECIFIED., .F., .F.,
 ( 4, 2, 2, 2, 2, 4 ),
 ( -2.000000094622903833E-05, 0.002989282327806173489, 0.005998564656558575368, 0.007503205820934752239, 0.009007846985310929977, 0.01201712931406334617 ),
 .UNSPECIFIED. ) ;
#11040=CARTESIAN_POINT ( 'NONE',  ( -7.946041369334237991, 195.0000000000000000, 26.05901981062767092 ) ) ;
#11044=CARTESIAN_POINT ( 'NONE',  ( -13.49999999999998401, 197.9375000012290400, 23.38268590217985476 ) ) ;
#11054=CARTESIAN_POINT ( 'NONE',  ( 18.00000000000000000, 247.7312500012290570, -5.196152422706630247 ) ) ;
#11061=CARTESIAN_POINT ( 'NONE',  ( 20.99999999999999645, 185.0294372515228645, -5.999999999999999112 ) ) ;
#11063=ADVANCED_FACE ( 'NONE', ( #3963 ), #1305, .F. ) ;
#11064=CARTESIAN_POINT ( 'NONE',  ( 23.87821517812499650, 248.3593750006145342, -4.985214923628404904 ) ) ;
#11066=CARTESIAN_POINT ( 'NONE',  ( 20.99999999999999645, 242.7718750006145854, 6.646953231504538984 ) ) ;
#11070=CARTESIAN_POINT ( 'NONE',  ( 15.00000000000000000, 248.6687500012290286, -3.464101615137752166 ) ) ;
#11074=LINE ( 'NONE', #13928, #25639 ) ;
#11077=EDGE_LOOP ( 'NONE', ( #2715, #27117, #21100, #11131 ) ) ;
#11086=ADVANCED_FACE ( 'NONE', ( #36357 ), #10025, .F. ) ;
#11089=CARTESIAN_POINT ( 'NONE',  ( 15.00964601948014732, 225.9742772813838769, -0.3926987779609585338 ) ) ;
#11091=CARTESIAN_POINT ( 'NONE',  ( 1.069080835302379631E-14, 196.9624999999999773, 27.00000000000000000 ) ) ;
#11099=CARTESIAN_POINT ( 'NONE',  ( -13.62178482187500528, 195.2281250006145399, -23.59362340125807123 ) ) ;
#11114=CARTESIAN_POINT ( 'NONE',  ( -26.99999999999998934, 197.3375000000000057, 15.58845726811991561 ) ) ;
#11118=CARTESIAN_POINT ( 'NONE',  ( 23.87821517812499650, 249.7093750006145285, -4.985214923628404904 ) ) ;
#11126=CARTESIAN_POINT ( 'NONE',  ( 26.99999999999999645, 243.0249999999999773, -7.347880794884117764E-16 ) ) ;
#11127=CARTESIAN_POINT ( 'NONE',  ( -7.234628195640289583, 198.5575961894323029, -27.00000000000001421 ) ) ;
#11131=ORIENTED_EDGE ( 'NONE', *, *, #16784, .T. ) ;
#11132=CARTESIAN_POINT ( 'NONE',  ( 13.50000000000001421, 194.8625000012290513, 23.38268590217984055 ) ) ;
#11137=CARTESIAN_POINT ( 'NONE',  ( 18.12178482187500350, 241.8343750006145285, 4.985214923628407568 ) ) ;
#11144=CARTESIAN_POINT ( 'NONE',  ( -13.62178482187500528, 197.5343750006145456, -23.59362340125807123 ) ) ;
#11159=CARTESIAN_POINT ( 'NONE',  ( 7.234628195640363302, 195.0299038117966575, -26.99999999999996803 ) ) ;
#11160=CARTESIAN_POINT ( 'NONE',  ( 26.99999999999999645, 248.4812500012290570, -7.347880794884117764E-16 ) ) ;
#11164=CARTESIAN_POINT ( 'NONE',  ( -4.500000000000001776, 227.8255434699758837, 2.500000000000000000 ) ) ;
#11168=CARTESIAN_POINT ( 'NONE',  ( 18.12178482187499640, 241.6843750006145513, -4.985214923628404904 ) ) ;
#11169=CARTESIAN_POINT ( 'NONE',  ( 27.24356964375000700, 199.5406250006145967, 15.72908226750537075 ) ) ;
#11172=ORIENTED_EDGE ( 'NONE', *, *, #7834, .T. ) ;
#11174=CARTESIAN_POINT ( 'NONE',  ( 23.87821517812499650, 241.0468750006145058, -4.985214923628404904 ) ) ;
#11184=CARTESIAN_POINT ( 'NONE',  ( 26.75643035624999655, 243.2593750006145115, -3.323476615752271268 ) ) ;
#11194=CARTESIAN_POINT ( 'NONE',  ( 19.39230484541326049, 241.4138461906613884, -5.999999999999997335 ) ) ;
#11203=CARTESIAN_POINT ( 'NONE',  ( 23.99999999999999645, 241.3000000000000114, -5.196152422706631135 ) ) ;
#11205=CARTESIAN_POINT ( 'NONE',  ( -27.24356964374999635, 196.7468750006145797, 15.72908226750539384 ) ) ;
#11206=CARTESIAN_POINT ( 'NONE',  ( 26.99999999999999645, 246.1750000000000114, -7.347880794884117764E-16 ) ) ;
#11207=DIRECTION ( 'NONE',  ( 0.000000000000000000, -1.000000000000000000, 0.000000000000000000 ) ) ;
#11211=( BOUNDED_CURVE ( )  B_SPLINE_CURVE ( 2, ( #11701, #8313, #34453, #31427, #31607, #25736, #22906, #20249, #23088 ),
 .UNSPECIFIED., .F., .F. ) 
 B_SPLINE_CURVE_WITH_KNOTS ( ( 3, 2, 2, 2, 3 ),
 ( 0.9021739130434782705, 0.9057971014492753881, 0.9130434782608695121, 0.9202898550724637472, 0.9239130434782608647 ),
 .UNSPECIFIED. ) 
 CURVE ( )  GEOMETRIC_REPRESENTATION_ITEM ( )  RATIONAL_B_SPLINE_CURVE ( ( 0.9330127018922194093, 0.9330127018922194093, 1.000000000000000000, 0.8660254037844387076, 1.000000000000000000, 0.8660254037844387076, 1.000000000000000000, 0.9330127018922194093, 0.9330127018922194093 ) ) 
 REPRESENTATION_ITEM ( '' )  );
#11212=CARTESIAN_POINT ( 'NONE',  ( 15.00000000000000000, 240.6062500012290286, 0.000000000000000000 ) ) ;
#11218=ORIENTED_EDGE ( 'NONE', *, *, #28378, .F. ) ;
#11222=EDGE_CURVE ( 'NONE', #4778, #13411, #32608, .T. ) ;
#11223=VECTOR ( 'NONE', #3788, 1000.000000000000000 ) ;
#11230=ORIENTED_EDGE ( 'NONE', *, *, #4506, .F. ) ;
#11241=LINE ( 'NONE', #13346, #29024 ) ;
#11244=CARTESIAN_POINT ( 'NONE',  ( -13.50000000000000533, 199.0250000000000057, -23.38268590217984411 ) ) ;
#11247=CYLINDRICAL_SURFACE ( 'NONE', #32675, 27.00000000000000000 ) ;
#11250=CARTESIAN_POINT ( 'NONE',  ( 23.87821517812499650, 244.3093750006145228, -4.985214923628404904 ) ) ;
#11252=CARTESIAN_POINT ( 'NONE',  ( 26.75643035624999655, 241.1218750006145228, -3.323476615752271268 ) ) ;
#11253=ORIENTED_EDGE ( 'NONE', *, *, #6629, .F. ) ;
#11256=CARTESIAN_POINT ( 'NONE',  ( 24.00000000000000000, 248.8562500012290570, 5.196152422706629359 ) ) ;
#11272=CARTESIAN_POINT ( 'NONE',  ( 23.87821517812500005, 248.9968750006145228, 4.985214923628404016 ) ) ;
#11277=CARTESIAN_POINT ( 'NONE',  ( 14.97710761593488904, 216.0228923840610662, 0.2612666680233010630 ) ) ;
#11290=CARTESIAN_POINT ( 'NONE',  ( 23.99999999999999645, 242.2562500012290627, -5.196152422706631135 ) ) ;
#11298=CARTESIAN_POINT ( 'NONE',  ( 20.99999999999999645, 185.0294372515228645, 0.000000000000000000 ) ) ;
#11300=CARTESIAN_POINT ( 'NONE',  ( 21.00000000000000000, 243.4187500012290002, 5.999999999999998224 ) ) ;
#11302=CARTESIAN_POINT ( 'NONE',  ( -27.00000000000000355, 197.7500000000000000, 0.000000000000000000 ) ) ;
#11305=CARTESIAN_POINT ( 'NONE',  ( 20.99999999999999645, 249.7468750006145797, -6.646953231504538984 ) ) ;
#11306=ORIENTED_EDGE ( 'NONE', *, *, #27014, .F. ) ;
#11312=CARTESIAN_POINT ( 'NONE',  ( 15.00000000000000178, 242.8375000000000057, 3.464101615137757051 ) ) ;
#11313=CARTESIAN_POINT ( 'NONE',  ( -26.99999999999999645, 198.6875000000000284, 15.58845726811991561 ) ) ;
#11315=ORIENTED_EDGE ( 'NONE', *, *, #6818, .F. ) ;
#11318=CARTESIAN_POINT ( 'NONE',  ( -26.99999999999998934, 197.0000000012290400, 15.58845726811991561 ) ) ;
#11322=CARTESIAN_POINT ( 'NONE',  ( 15.24356964374999990, 243.5218750006145569, -3.323476615752268604 ) ) ;
#11325=CARTESIAN_POINT ( 'NONE',  ( 21.00000000000000000, 242.9687500012290684, 5.999999999999998224 ) ) ;
#11330=CARTESIAN_POINT ( 'NONE',  ( 27.00344680842688661, 195.0000000000000000, -2.333320423711915392 ) ) ;
#11331=CARTESIAN_POINT ( 'NONE',  ( 27.24356964375000700, 195.9968750006145513, 15.72908226750537075 ) ) ;
#11333=VERTEX_POINT ( 'NONE', #28570 ) ;
#11334=EDGE_CURVE ( 'NONE', #18637, #25480, #10939, .T. ) ;
#11351=CIRCLE ( 'NONE', #2253, 2.649999999999990585 ) ;
#11352=CARTESIAN_POINT ( 'NONE',  ( -3.253724281355068545E-15, 196.2874999999999659, -27.00000000000000000 ) ) ;
#11356=CARTESIAN_POINT ( 'NONE',  ( 23.87821517812500005, 240.1093750006145342, 4.985214923628404016 ) ) ;
#11357=CARTESIAN_POINT ( 'NONE',  ( 13.62178482187501416, 198.1531250006145228, 23.59362340125806767 ) ) ;
#11361=ORIENTED_EDGE ( 'NONE', *, *, #11334, .T. ) ;
#11362=CARTESIAN_POINT ( 'NONE',  ( 5.778771075727756162E-15, 198.1156250006145285, 31.45816453501075927 ) ) ;
#11363=CARTESIAN_POINT ( 'NONE',  ( 23.87821517812500005, 242.6968750006145115, 4.985214923628404016 ) ) ;
#11371=CARTESIAN_POINT ( 'NONE',  ( 15.24356964374999990, 244.7968750006145058, 0.000000000000000000 ) ) ;
#11373=CARTESIAN_POINT ( 'NONE',  ( 24.00000000000000000, 246.6062500012290570, 5.196152422706629359 ) ) ;
#11378=AXIS2_PLACEMENT_3D ( 'NONE', #28816, #34512, #20119 ) ;
#11382=CARTESIAN_POINT ( 'NONE',  ( 20.99999999999999289, 241.3937500012289945, -5.999999999999997335 ) ) ;
#11385=EDGE_LOOP ( 'NONE', ( #8265, #8645, #26661, #24287 ) ) ;
#11389=FACE_OUTER_BOUND ( 'NONE', #8557, .T. ) ;
#11391=CARTESIAN_POINT ( 'NONE',  ( -13.62178482187500528, 195.2843750006145456, -23.59362340125807123 ) ) ;
#11392=CARTESIAN_POINT ( 'NONE',  ( 22.60769515458672174, 246.0825961894323370, 6.000000000000004441 ) ) ;
#11393=CARTESIAN_POINT ( 'NONE',  ( 3.306546357697853733E-15, 210.0000000000000284, 27.00000000000000000 ) ) ;
#11394=EDGE_CURVE ( 'NONE', #24643, #483, #25737, .T. ) ;
#11399=VERTEX_POINT ( 'NONE', #31609 ) ;
#11400=CARTESIAN_POINT ( 'NONE',  ( 15.24356964374999990, 248.8093750006144944, -3.323476615752268604 ) ) ;
#11406=AXIS2_PLACEMENT_3D ( 'NONE', #36898, #28192, #10760 ) ;
#11409=EDGE_CURVE ( 'NONE', #5512, #25530, #29068, .T. ) ;
#11411=EDGE_CURVE ( 'NONE', #10569, #253, #36603, .T. ) ;
#11414=CARTESIAN_POINT ( 'NONE',  ( -20.75254460673100709, 194.9999999999999716, 17.57977308427575025 ) ) ;
#11420=CARTESIAN_POINT ( 'NONE',  ( -27.00000000000000355, 197.8250000012290570, -15.58845726811989429 ) ) ;
#11435=CARTESIAN_POINT ( 'NONE',  ( 18.12178482187499640, 246.1843750006145228, -4.985214923628404904 ) ) ;
#11437=CARTESIAN_POINT ( 'NONE',  ( 26.75643035624999655, 242.9218750006145626, -3.323476615752271268 ) ) ;
#11441=CARTESIAN_POINT ( 'NONE',  ( 24.00000000000000000, 245.2562500012290627, 5.196152422706629359 ) ) ;
#11442=ORIENTED_EDGE ( 'NONE', *, *, #28150, .F. ) ;
#11455=CARTESIAN_POINT ( 'NONE',  ( 21.00000000000000000, 245.8093750006144944, 6.646953231504538984 ) ) ;
#11470=VERTEX_POINT ( 'NONE', #26664 ) ;
#11480=DIRECTION ( 'NONE',  ( -0.000000000000000000, -1.000000000000000000, -0.000000000000000000 ) ) ;
#11484=CARTESIAN_POINT ( 'NONE',  ( -13.50000000000000533, 196.7750000000000057, -23.38268590217984411 ) ) ;
#11487=CARTESIAN_POINT ( 'NONE',  ( 18.12178482187500350, 248.5843750006145285, 4.985214923628407568 ) ) ;
#11494=CARTESIAN_POINT ( 'NONE',  ( 26.99999999999999645, 241.2249999999999943, -7.347880794884117764E-16 ) ) ;
#11498=ORIENTED_EDGE ( 'NONE', *, *, #10244, .F. ) ;
#11500=CARTESIAN_POINT ( 'NONE',  ( 27.00000000000000355, 195.8375000012290457, -3.306546357697854128E-15 ) ) ;
#11507=CARTESIAN_POINT ( 'NONE',  ( 18.00000000000000000, 242.7812500012290400, -5.196152422706630247 ) ) ;
#11512=CARTESIAN_POINT ( 'NONE',  ( 12.48663586349064403, 194.9999999999999716, 24.21355016816918493 ) ) ;
#11513=CARTESIAN_POINT ( 'NONE',  ( -27.24356964374999635, 196.2968750006145342, 15.72908226750539384 ) ) ;
#11515=EDGE_CURVE ( 'NONE', #9547, #18985, #23089, .T. ) ;
#11518=FACE_OUTER_BOUND ( 'NONE', #23809, .T. ) ;
#11523=CARTESIAN_POINT ( 'NONE',  ( 7.234628195640295800, 197.0950961906613941, 27.00000000000001066 ) ) ;
#11533=CARTESIAN_POINT ( 'NONE',  ( -13.62178482187498396, 195.4343750006145228, 23.59362340125808188 ) ) ;
#11537=CARTESIAN_POINT ( 'NONE',  ( 26.75643035624999655, 240.2218750006145171, -3.323476615752271712 ) ) ;
#11538=CARTESIAN_POINT ( 'NONE',  ( -13.62178482187500528, 198.3781250006145171, -23.59362340125807123 ) ) ;
#11543=CARTESIAN_POINT ( 'NONE',  ( -13.62178482187498396, 197.1781250006145569, 23.59362340125808188 ) ) ;
#11544=CARTESIAN_POINT ( 'NONE',  ( 26.75643035624999655, 242.3218750006145399, -7.049594010296217766E-16 ) ) ;
#11549=EDGE_CURVE ( 'NONE', #23800, #16763, #22939, .T. ) ;
#11553=CARTESIAN_POINT ( 'NONE',  ( 15.24356964375000167, 242.1343750006145683, 3.323476615752272600 ) ) ;
#11560=CARTESIAN_POINT ( 'NONE',  ( 21.00000000000000000, 239.8187500012290059, 5.999999999999998224 ) ) ;
#11562=CARTESIAN_POINT ( 'NONE',  ( 1.069080835302379631E-14, 198.8750000012290400, 27.00000000000000000 ) ) ;
#11565=CARTESIAN_POINT ( 'NONE',  ( -27.12178482187499995, 199.9296875003072671, 0.000000000000000000 ) ) ;
#11569=CARTESIAN_POINT ( 'NONE',  ( 26.75643035624999655, 243.2218750006145171, -7.049594010296217766E-16 ) ) ;
#11575=CARTESIAN_POINT ( 'NONE',  ( 20.99999999999999289, 243.5874999999999488, -5.999999999999997335 ) ) ;
#11576=CARTESIAN_POINT ( 'NONE',  ( 20.99999999999999645, 185.0294372515228645, 5.999999999999999112 ) ) ;
#11582=CARTESIAN_POINT ( 'NONE',  ( 21.00000000000000000, 249.4093750006145171, 6.646953231504538984 ) ) ;
#11592=CARTESIAN_POINT ( 'NONE',  ( 20.99999999999999645, 249.4093750006145171, 6.646953231504538984 ) ) ;
#11594=CARTESIAN_POINT ( 'NONE',  ( -26.95863322649103111, 194.9999999999998863, -2.574242593721492334 ) ) ;
#11598=ORIENTED_EDGE ( 'NONE', *, *, #20298, .F. ) ;
#11606=ORIENTED_EDGE ( 'NONE', *, *, #1948, .T. ) ;
#11608=AXIS2_PLACEMENT_3D ( 'NONE', #5970, #17550, #31389 ) ;
#11612=CARTESIAN_POINT ( 'NONE',  ( 27.00000000000001421, 196.2500000012290116, 15.58845726811988897 ) ) ;
#11613=CARTESIAN_POINT ( 'NONE',  ( -3.253724281355068545E-15, 197.6374999999999602, -27.00000000000000000 ) ) ;
#11614=CARTESIAN_POINT ( 'NONE',  ( 26.99999999999999645, 246.1937500012290343, 3.464101615137751278 ) ) ;
#11615=CARTESIAN_POINT ( 'NONE',  ( 15.24356964374999990, 245.7718750006145001, -3.323476615752268604 ) ) ;
#11621=CARTESIAN_POINT ( 'NONE',  ( 15.00000000000000000, 246.8687500012290457, -3.464101615137752166 ) ) ;
#11625=CARTESIAN_POINT ( 'NONE',  ( 13.50000000000001421, 198.0125000012290286, 23.38268590217984055 ) ) ;
#11630=ORIENTED_EDGE ( 'NONE', *, *, #11687, .F. ) ;
#11635=CARTESIAN_POINT ( 'NONE',  ( 23.87821517812500005, 247.6468750006145285, 4.985214923628404016 ) ) ;
#11638=CARTESIAN_POINT ( 'NONE',  ( 17.99309595496827541, 218.0184107867384000, -5.206989594057217730 ) ) ;
#11660=EDGE_CURVE ( 'NONE', #35488, #10943, #2797, .T. ) ;
#11663=CARTESIAN_POINT ( 'NONE',  ( 13.62178482187501416, 199.5593750006145513, 23.59362340125806767 ) ) ;
#11666=CARTESIAN_POINT ( 'NONE',  ( 26.75643035624999655, 248.3218750006145399, -3.323476615752271268 ) ) ;
#11674=CARTESIAN_POINT ( 'NONE',  ( 21.00000000000000000, 240.2125000000000057, 6.928203230275506996 ) ) ;
#11682=CARTESIAN_POINT ( 'NONE',  ( -13.50000000000000533, 195.0875000012290457, -23.38268590217984411 ) ) ;
#11687=EDGE_CURVE ( 'NONE', #190, #8211, #1741, .T. ) ;
#11688=CARTESIAN_POINT ( 'NONE',  ( 15.24356964375000167, 241.3468750006145456, 3.323476615752272600 ) ) ;
#11696=CARTESIAN_POINT ( 'NONE',  ( 13.62178482187501416, 195.5093750006145399, 23.59362340125806767 ) ) ;
#11701=CARTESIAN_POINT ( 'NONE',  ( 21.00000000000000000, 240.6624999999999943, 5.999999999999998224 ) ) ;
#11709=CARTESIAN_POINT ( 'NONE',  ( 20.99999999999995381, 244.7125000000000057, 5.999999999999998224 ) ) ;
#11713=ORIENTED_EDGE ( 'NONE', *, *, #1726, .F. ) ;
#11716=DIRECTION ( 'NONE',  ( -0.000000000000000000, 1.000000000000000000, -0.000000000000000000 ) ) ;
#11717=EDGE_CURVE ( 'NONE', #3008, #7787, #18912, .T. ) ;
#11721=CARTESIAN_POINT ( 'NONE',  ( 15.00000000000000000, 247.2999999999999829, 0.000000000000000000 ) ) ;
#11722=CARTESIAN_POINT ( 'NONE',  ( -27.24356964374999279, 199.3906250006145342, 15.72908226750539384 ) ) ;
#11724=( BOUNDED_CURVE ( )  B_SPLINE_CURVE ( 2, ( #22649, #16590, #36661, #5008, #10699, #27765, #28134, #22090, #34195 ),
 .UNSPECIFIED., .F., .F. ) 
 B_SPLINE_CURVE_WITH_KNOTS ( ( 3, 2, 2, 2, 3 ),
 ( 0.8369565217391303769, 0.8405797101449274944, 0.8478260869565217295, 0.8550724637681159646, 0.8586956521739130821 ),
 .UNSPECIFIED. ) 
 CURVE ( )  GEOMETRIC_REPRESENTATION_ITEM ( )  RATIONAL_B_SPLINE_CURVE ( ( 0.9330127018922192983, 0.9330127018922182991, 1.000000000000000000, 0.8660254037844387076, 1.000000000000000000, 0.8660254037844387076, 1.000000000000000000, 0.9330127018922194093, 0.9330127018922194093 ) ) 
 REPRESENTATION_ITEM ( '' )  );
#11727=ORIENTED_EDGE ( 'NONE', *, *, #2771, .F. ) ;
#11729=CARTESIAN_POINT ( 'NONE',  ( -27.24356964374999635, 197.1406250006145058, 15.72908226750539384 ) ) ;
#11730=CARTESIAN_POINT ( 'NONE',  ( 15.24356964374999990, 242.5093750006144830, -3.323476615752268604 ) ) ;
#11734=CARTESIAN_POINT ( 'NONE',  ( 15.24356964374999990, 248.4718750006145171, -3.323476615752268604 ) ) ;
#11736=EDGE_CURVE ( 'NONE', #21332, #17896, #21191, .T. ) ;
#11741=CARTESIAN_POINT ( 'NONE',  ( 15.24356964375000167, 241.2343750006145058, 3.323476615752272600 ) ) ;
#11743=CARTESIAN_POINT ( 'NONE',  ( 20.99999999999997868, 246.5687500012290343, 5.999999999999999112 ) ) ;
#11755=CARTESIAN_POINT ( 'NONE',  ( 18.12178482187500350, 243.0718750006145399, 4.985214923628407568 ) ) ;
#11764=CARTESIAN_POINT ( 'NONE',  ( 26.99999999999999645, 241.2624999999999886, -3.464101615137755275 ) ) ;
#11765=CARTESIAN_POINT ( 'NONE',  ( -13.62178482187500528, 196.6343750006145399, -23.59362340125807123 ) ) ;
#11772=CARTESIAN_POINT ( 'NONE',  ( 15.00000000000000000, 240.1187500012290172, -3.464101615137752166 ) ) ;
#11782=CARTESIAN_POINT ( 'NONE',  ( 18.12178482187499640, 248.3218750006145115, -4.985214923628404904 ) ) ;
#11783=CARTESIAN_POINT ( 'NONE',  ( -24.63748681676955954, 195.0000000000001137, -11.14284646165792481 ) ) ;
#11787=VERTEX_POINT ( 'NONE', #885 ) ;
#11788=CARTESIAN_POINT ( 'NONE',  ( -28.92959262791929476, 202.2584803510073641, 2.084043131378895186 ) ) ;
#11797=CARTESIAN_POINT ( 'NONE',  ( 1.120210788295102201E-13, 195.5000000012290400, -27.00000000000000711 ) ) ;
#11804=CARTESIAN_POINT ( 'NONE',  ( 23.87821517812500005, 244.6093750006145342, 4.985214923628404016 ) ) ;
#11806=CARTESIAN_POINT ( 'NONE',  ( 20.99999999999999645, 240.2968750006145342, -6.646953231504538984 ) ) ;
#11809=CARTESIAN_POINT ( 'NONE',  ( 18.00000000000000355, 245.6312500012290343, 5.196152422706632912 ) ) ;
#11812=CARTESIAN_POINT ( 'NONE',  ( 19.39230484541324984, 246.9424038105676118, 5.999999999999991118 ) ) ;
#11816=EDGE_LOOP ( 'NONE', ( #15750, #25316, #14668, #21821, #9589, #21843 ) ) ;
#11819=VERTEX_POINT ( 'NONE', #26856 ) ;
#11822=CARTESIAN_POINT ( 'NONE',  ( 23.87821517812499650, 247.7968750006145058, -4.985214923628404904 ) ) ;
#11825=CARTESIAN_POINT ( 'NONE',  ( 13.90958069845121869, 212.6589072380886023, -5.392997762646073667 ) ) ;
#11836=VERTEX_POINT ( 'NONE', #10361 ) ;
#11842=CYLINDRICAL_SURFACE ( 'NONE', #10716, 5.999999999999999112 ) ;
#11850=CARTESIAN_POINT ( 'NONE',  ( 26.99999999999999645, 196.2125000000000057, -15.58845726811990495 ) ) ;
#11853=CARTESIAN_POINT ( 'NONE',  ( 15.24356964375000167, 245.8468750006145171, 3.323476615752272600 ) ) ;
#11854=ORIENTED_EDGE ( 'NONE', *, *, #18430, .T. ) ;
#11860=CARTESIAN_POINT ( 'NONE',  ( 15.00000000000000000, 241.4499999999999886, 0.000000000000000000 ) ) ;
#11863=EDGE_LOOP ( 'NONE', ( #19937, #26774, #36032, #6116 ) ) ;
#11865=DIRECTION ( 'NONE',  ( -0.000000000000000000, 1.000000000000000000, -0.000000000000000000 ) ) ;
#11866=CARTESIAN_POINT ( 'NONE',  ( 26.99999999999999645, 246.5874999999999773, 3.464101615137751278 ) ) ;
#11870=CARTESIAN_POINT ( 'NONE',  ( 26.99999999999999645, 249.3624999999999829, -3.464101615137755275 ) ) ;
#11871=CARTESIAN_POINT ( 'NONE',  ( 15.24356964374999990, 241.2718750006145569, -3.323476615752268604 ) ) ;
#11882=CARTESIAN_POINT ( 'NONE',  ( 27.24356964375000700, 195.5468750006145342, 15.72908226750537075 ) ) ;
#11896=CARTESIAN_POINT ( 'NONE',  ( 26.99999999999999645, 245.6875000000000000, 3.464101615137751278 ) ) ;
#11901=ORIENTED_EDGE ( 'NONE', *, *, #12401, .T. ) ;
#11904=CARTESIAN_POINT ( 'NONE',  ( 27.24356964374999279, 195.6218750006145228, -15.72908226750539207 ) ) ;
#11908=CARTESIAN_POINT ( 'NONE',  ( 21.00000000000000000, 247.4125000000000227, 6.928203230275506996 ) ) ;
#11909=CARTESIAN_POINT ( 'NONE',  ( 27.24356964375000700, 198.1906250006145740, 15.72908226750537075 ) ) ;
#11914=ORIENTED_EDGE ( 'NONE', *, *, #2844, .F. ) ;
#11915=CARTESIAN_POINT ( 'NONE',  ( 13.62178482187499640, 195.1531250006145513, -23.59362340125807123 ) ) ;
#11916=CARTESIAN_POINT ( 'NONE',  ( 21.00000000000000000, 243.3343750006145285, -6.646953231504538984 ) ) ;
#11920=CARTESIAN_POINT ( 'NONE',  ( 15.24356964374999990, 246.7093750006145569, 0.000000000000000000 ) ) ;
#11925=CARTESIAN_POINT ( 'NONE',  ( 26.75643035624999655, 241.8718750006145228, -7.049594010296217766E-16 ) ) ;
#11937=CARTESIAN_POINT ( 'NONE',  ( 20.99999999999997513, 245.3875000000000455, -5.999999999999999112 ) ) ;
#11939=CARTESIAN_POINT ( 'NONE',  ( 13.49999999999999645, 199.0625000012290400, -23.38268590217984766 ) ) ;
#11940=( BOUNDED_CURVE ( )  B_SPLINE_CURVE ( 3, ( #24559, #36109, #13559, #24925 ),
 .UNSPECIFIED., .F., .F. ) 
 B_SPLINE_CURVE_WITH_KNOTS ( ( 4, 4 ),
 ( 0.000000000000000000, 1.570796326794895670 ),
 .UNSPECIFIED. ) 
 CURVE ( )  GEOMETRIC_REPRESENTATION_ITEM ( )  RATIONAL_B_SPLINE_CURVE ( ( 1.000000000000000000, 0.8047378541243652705, 0.8047378541243652705, 1.000000000000000000 ) ) 
 REPRESENTATION_ITEM ( '' )  );
#11943=CARTESIAN_POINT ( 'NONE',  ( 26.75643035624999655, 241.4593750006145285, -3.323476615752271712 ) ) ;
#11944=ORIENTED_EDGE ( 'NONE', *, *, #10244, .T. ) ;
#11945=DIRECTION ( 'NONE',  ( -1.000000000000000000, -6.123233995736766036E-17, 0.000000000000000000 ) ) ;
#11949=CYLINDRICAL_SURFACE ( 'NONE', #22148, 5.999999999999999112 ) ;
#11950=FACE_OUTER_BOUND ( 'NONE', #20514, .T. ) ;
#11951=CARTESIAN_POINT ( 'NONE',  ( 4.611372152710607075, 195.0000000000000000, 26.85403668788741527 ) ) ;
#11956=CARTESIAN_POINT ( 'NONE',  ( 24.00000000000000000, 240.3062500012290457, 5.196152422706629359 ) ) ;
#11968=CARTESIAN_POINT ( 'NONE',  ( -26.64709556143852964, 195.0000000000000853, -4.774896623102089954 ) ) ;
#11973=CARTESIAN_POINT ( 'NONE',  ( 18.00000000000000000, 248.5749999999999886, -5.196152422706630247 ) ) ;
#11982=ORIENTED_EDGE ( 'NONE', *, *, #31483, .F. ) ;
#11991=CARTESIAN_POINT ( 'NONE',  ( 23.87821517812499650, 246.1093750006145342, -4.985214923628404904 ) ) ;
#11993=CARTESIAN_POINT ( 'NONE',  ( 15.24356964374999990, 240.4093750006145456, 0.000000000000000000 ) ) ;
#11997=CARTESIAN_POINT ( 'NONE',  ( 15.00000000000000178, 246.4937500012290457, 3.464101615137757051 ) ) ;
#12008=CARTESIAN_POINT ( 'NONE',  ( 23.87821517812500005, 246.7468750006145228, 4.985214923628404016 ) ) ;
#12012=VECTOR ( 'NONE', #32730, 1000.000000000000000 ) ;
#12014=( NAMED_UNIT ( * ) SI_UNIT ( $, .STERADIAN. ) SOLID_ANGLE_UNIT ( ) );
#12017=EDGE_CURVE ( 'NONE', #31527, #33538, #15993, .T. ) ;
#12022=CARTESIAN_POINT ( 'NONE',  ( -27.24356964374999635, 194.8906250006145342, 15.72908226750539384 ) ) ;
#12029=CARTESIAN_POINT ( 'NONE',  ( 19.97220920615905371, 239.6536485351579699, -5.828890057712500017 ) ) ;
#12040=CARTESIAN_POINT ( 'NONE',  ( 23.87821517812500005, 245.5093750006145399, 4.985214923628404016 ) ) ;
#12047=CARTESIAN_POINT ( 'NONE',  ( 21.00000000000000000, 241.7874999999999943, -6.928203230275506996 ) ) ;
#12052=LINE ( 'NONE', #14349, #3058 ) ;
#12054=CARTESIAN_POINT ( 'NONE',  ( 18.00000000000000355, 248.2750000000000057, 5.196152422706632912 ) ) ;
#12059=CARTESIAN_POINT ( 'NONE',  ( 18.12178482187500350, 240.9343750006145513, 4.985214923628407568 ) ) ;
#12067=CARTESIAN_POINT ( 'NONE',  ( 17.54540804174073187, 195.0000000000000000, -20.52215039046394907 ) ) ;
#12068=CARTESIAN_POINT ( 'NONE',  ( -27.24356964374999635, 196.7468750006145797, 15.72908226750539384 ) ) ;
#12071=VERTEX_POINT ( 'NONE', #33856 ) ;
#12073=CARTESIAN_POINT ( 'NONE',  ( 20.99999999999999289, 244.5437500012290570, -5.999999999999997335 ) ) ;
#12084=CARTESIAN_POINT ( 'NONE',  ( 20.99999999999998579, 247.6937500012290059, -5.999999999999997335 ) ) ;
#12085=ORIENTED_EDGE ( 'NONE', *, *, #6247, .F. ) ;
#12088=CARTESIAN_POINT ( 'NONE',  ( -26.99999999999999645, 198.3500000012290343, 15.58845726811991561 ) ) ;
#12092=CARTESIAN_POINT ( 'NONE',  ( 18.00000000000000000, 247.6750000000000114, -5.196152422706630247 ) ) ;
#12093=CARTESIAN_POINT ( 'NONE',  ( 27.24356964374999279, 196.9156250006145399, -15.72908226750539207 ) ) ;
#12097=ORIENTED_EDGE ( 'NONE', *, *, #35164, .F. ) ;
#12098=CARTESIAN_POINT ( 'NONE',  ( 27.24356964375000345, 195.5281250006145228, -3.336375036156643733E-15 ) ) ;
#12099=CARTESIAN_POINT ( 'NONE',  ( 23.87821517812500005, 239.9968750006144944, 4.985214923628404016 ) ) ;
#12102=CARTESIAN_POINT ( 'NONE',  ( 26.75643035624999655, 248.3218750006145399, -3.323476615752271712 ) ) ;
#12108=CARTESIAN_POINT ( 'NONE',  ( 26.75643035624999655, 240.9718750006145171, -7.049594010296217766E-16 ) ) ;
#12120=CARTESIAN_POINT ( 'NONE',  ( 15.12178482187499995, 249.9296875003072387, 0.000000000000000000 ) ) ;
#12126=CARTESIAN_POINT ( 'NONE',  ( 18.12178482187500350, 242.6218750006145228, 4.985214923628407568 ) ) ;
#12127=EDGE_LOOP ( 'NONE', ( #9129, #11361, #22790, #2673 ) ) ;
#12131=CARTESIAN_POINT ( 'NONE',  ( 2.999999999999997780, 244.5000000000000000, 2.500000000000000000 ) ) ;
#12139=CARTESIAN_POINT ( 'NONE',  ( 21.00000000000000000, 249.1843750006144944, -6.646953231504538984 ) ) ;
#12165=CARTESIAN_POINT ( 'NONE',  ( 18.00000000000000355, 246.5312500012290400, 5.196152422706632912 ) ) ;
#12169=CARTESIAN_POINT ( 'NONE',  ( 5.438367727407757144E-14, 197.7500000012290400, -27.00000000000000000 ) ) ;
#12171=CARTESIAN_POINT ( 'NONE',  ( 19.39230484541326760, 242.4424038105676686, 5.999999999999999112 ) ) ;
#12178=CARTESIAN_POINT ( 'NONE',  ( 26.75643035624999655, 242.4718750006145456, -3.323476615752271712 ) ) ;
#12180=CARTESIAN_POINT ( 'NONE',  ( 20.99999999999999645, 240.5218750006145285, 6.646953231504538984 ) ) ;
#12183=CARTESIAN_POINT ( 'NONE',  ( 18.00000000000000000, 245.4812500012290570, -5.196152422706630247 ) ) ;
#12187=CARTESIAN_POINT ( 'NONE',  ( 19.39230484541324628, 246.7575961894322631, -5.999999999999989342 ) ) ;
#12191=ORIENTED_EDGE ( 'NONE', *, *, #10512, .T. ) ;
#12195=CARTESIAN_POINT ( 'NONE',  ( 15.24356964374999990, 245.6968750006145115, 0.000000000000000000 ) ) ;
#12198=CARTESIAN_POINT ( 'NONE',  ( 14.16903250679951043, 216.8309674931686004, -1.338899061176967997 ) ) ;
#12200=SURFACE_SIDE_STYLE ('',( #26602 ) ) ;
#12201=( BOUNDED_CURVE ( )  B_SPLINE_CURVE ( 2, ( #12264, #35191, #9238, #17966, #29508, #3549, #26663, #23835, #35376 ),
 .UNSPECIFIED., .F., .T. ) 
 B_SPLINE_CURVE_WITH_KNOTS ( ( 3, 2, 2, 2, 3 ),
 ( 0.4021739130434782705, 0.4057971014492753881, 0.4130434782608695676, 0.4202898550724637472, 0.4239130434782608647 ),
 .UNSPECIFIED. ) 
 CURVE ( )  GEOMETRIC_REPRESENTATION_ITEM ( )  RATIONAL_B_SPLINE_CURVE ( ( 0.9330127018922194093, 0.9330127018922194093, 1.000000000000000000, 0.8660254037844387076, 1.000000000000000000, 0.8660254037844387076, 1.000000000000000000, 0.9330127018922194093, 0.9330127018922194093 ) ) 
 REPRESENTATION_ITEM ( '' )  );
#12203=AXIS2_PLACEMENT_3D ( 'NONE', #5547, #7854, #27753 ) ;
#12211=AXIS2_PLACEMENT_3D ( 'NONE', #11298, #22687, #95 ) ;
#12223=CARTESIAN_POINT ( 'NONE',  ( 24.00000000000000000, 241.2062500012290513, 5.196152422706629359 ) ) ;
#12225=CARTESIAN_POINT ( 'NONE',  ( 20.99999999999999645, 192.3000000000000398, 0.000000000000000000 ) ) ;
#12227=CARTESIAN_POINT ( 'NONE',  ( 15.24356964375000167, 247.6468750006145854, 3.323476615752272600 ) ) ;
#12232=LINE ( 'NONE', #29477, #17113 ) ;
#12235=CARTESIAN_POINT ( 'NONE',  ( 21.00000000000000000, 242.2374999999999829, -6.928203230275506996 ) ) ;
#12238=ORIENTED_EDGE ( 'NONE', *, *, #37101, .F. ) ;
#12240=CARTESIAN_POINT ( 'NONE',  ( 7.234628195640363302, 196.8299038117967257, -26.99999999999996803 ) ) ;
#12242=DIRECTION ( 'NONE',  ( 0.000000000000000000, 0.000000000000000000, 1.000000000000000000 ) ) ;
#12249=CARTESIAN_POINT ( 'NONE',  ( -3.253724281355068545E-15, 195.9500000012290002, -27.00000000000000355 ) ) ;
#12259=CARTESIAN_POINT ( 'NONE',  ( 13.62178482187499640, 198.3031250006145285, -23.59362340125807123 ) ) ;
#12264=CARTESIAN_POINT ( 'NONE',  ( 20.99999999999999289, 245.4437500012290343, -5.999999999999997335 ) ) ;
#12273=LINE ( 'NONE', #32545, #11017 ) ;
#12276=CYLINDRICAL_SURFACE ( 'NONE', #6383, 27.00000000000000000 ) ;
#12277=CARTESIAN_POINT ( 'NONE',  ( 20.99999999999999645, 185.0294372515228645, 0.000000000000000000 ) ) ;
#12280=CARTESIAN_POINT ( 'NONE',  ( -4.694659320240884604E-14, 197.4124999999999943, 27.00000000000000000 ) ) ;
#12285=CARTESIAN_POINT ( 'NONE',  ( 15.00000000000000000, 247.7500000000000000, 0.000000000000000000 ) ) ;
#12286=CARTESIAN_POINT ( 'NONE',  ( 27.24356964375000345, 196.8781250006145171, -3.336375036156643733E-15 ) ) ;
#12291=CARTESIAN_POINT ( 'NONE',  ( -13.62178482187500528, 195.6781250006145569, -23.59362340125807123 ) ) ;
#12292=CARTESIAN_POINT ( 'NONE',  ( 26.75643035624999655, 240.9343750006144944, 3.323476615752267715 ) ) ;
#12295=CARTESIAN_POINT ( 'NONE',  ( 26.75643035624999655, 247.3468750006145171, 3.323476615752267715 ) ) ;
#12301=CARTESIAN_POINT ( 'NONE',  ( 18.12178482187499640, 242.4718750006145171, -4.985214923628404904 ) ) ;
#12312=CARTESIAN_POINT ( 'NONE',  ( 20.99999999999998579, 248.3124999999999716, 5.999999999999998224 ) ) ;
#12313=LINE ( 'NONE', #26522, #32149 ) ;
#12320=CARTESIAN_POINT ( 'NONE',  ( 26.75643035624999655, 243.2593750006145115, -3.323476615752271712 ) ) ;
#12321=ORIENTED_EDGE ( 'NONE', *, *, #14077, .T. ) ;
#12324=CARTESIAN_POINT ( 'NONE',  ( 5.778771075727756162E-15, 199.5218750006145569, 31.45816453501076637 ) ) ;
#12325=DIRECTION ( 'NONE',  ( -0.9848055780335318588, 2.371220701776928982E-05, 0.1736605105133940674 ) ) ;
#12332=CARTESIAN_POINT ( 'NONE',  ( 26.75643035624999655, 246.4093750006145171, -3.323476615752271712 ) ) ;
#12341=ORIENTED_EDGE ( 'NONE', *, *, #2771, .T. ) ;
#12345=CARTESIAN_POINT ( 'NONE',  ( 0.000000000000000000, 210.0000000000000284, -28.99999999999999645 ) ) ;
#12352=ORIENTED_EDGE ( 'NONE', *, *, #6818, .T. ) ;
#12353=LINE ( 'NONE', #23926, #13113 ) ;
#12359=CARTESIAN_POINT ( 'NONE',  ( 20.99999999999999645, 202.0000000000000000, 0.000000000000000000 ) ) ;
#12363=ORIENTED_EDGE ( 'NONE', *, *, #31285, .F. ) ;
#12364=CARTESIAN_POINT ( 'NONE',  ( 26.99999999999999645, 197.6750000012290229, -15.58845726811990495 ) ) ;
#12370=CARTESIAN_POINT ( 'NONE',  ( 13.49999999999999645, 195.9125000012290343, -23.38268590217984766 ) ) ;
#12377=CARTESIAN_POINT ( 'NONE',  ( 26.99999999999999645, 243.1187500012290172, -3.464101615137755275 ) ) ;
#12380=FACE_OUTER_BOUND ( 'NONE', #15088, .T. ) ;
#12389=CARTESIAN_POINT ( 'NONE',  ( 26.75643035624999655, 243.7093750006145285, -3.323476615752271712 ) ) ;
#12401=EDGE_CURVE ( 'NONE', #11787, #18467, #35437, .T. ) ;
#12405=CARTESIAN_POINT ( 'NONE',  ( 5.438367727407757775E-14, 198.0875000000000057, -27.00000000000000355 ) ) ;
#12417=CARTESIAN_POINT ( 'NONE',  ( 15.00000000000000178, 247.3937500012290513, 3.464101615137757051 ) ) ;
#12419=CARTESIAN_POINT ( 'NONE',  ( 18.12178482187500350, 245.4343750006145228, 4.985214923628407568 ) ) ;
#12422=CYLINDRICAL_SURFACE ( 'NONE', #21445, 5.999999999999999112 ) ;
#12423=EDGE_CURVE ( 'NONE', #29694, #6323, #26191, .T. ) ;
#12424=DIRECTION ( 'NONE',  ( 0.000000000000000000, 0.000000000000000000, 1.000000000000000000 ) ) ;
#12431=ORIENTED_EDGE ( 'NONE', *, *, #15030, .F. ) ;
#12432=FACE_OUTER_BOUND ( 'NONE', #22931, .T. ) ;
#12433=CARTESIAN_POINT ( 'NONE',  ( 20.99999999999999289, 243.5874999999999488, -5.999999999999997335 ) ) ;
#12434=CARTESIAN_POINT ( 'NONE',  ( 23.99999999999999645, 246.6999999999999886, -5.196152422706631135 ) ) ;
#12435=CARTESIAN_POINT ( 'NONE',  ( 13.50000000000001421, 195.2000000000000171, 23.38268590217984055 ) ) ;
#12439=CARTESIAN_POINT ( 'NONE',  ( 1.120210788295102201E-13, 197.1875000000000568, -27.00000000000000711 ) ) ;
#12441=CARTESIAN_POINT ( 'NONE',  ( 14.95628864315606421, 216.0437113568463303, 2.958957796639721582 ) ) ;
#12443=AXIS2_PLACEMENT_3D ( 'NONE', #22698, #7726, #4871 ) ;
#12450=CARTESIAN_POINT ( 'NONE',  ( 27.24356964374999635, 198.7156250006145513, -15.72908226750539029 ) ) ;
#12457=DIRECTION ( 'NONE',  ( -0.000000000000000000, -1.000000000000000000, -0.000000000000000000 ) ) ;
#12470=EDGE_CURVE ( 'NONE', #33602, #14808, #1208, .T. ) ;
#12476=CARTESIAN_POINT ( 'NONE',  ( 15.00000000000000178, 247.3374999999999773, 3.464101615137757051 ) ) ;
#12477=CARTESIAN_POINT ( 'NONE',  ( -13.62178482187500528, 195.6781250006145569, -23.59362340125807123 ) ) ;
#12482=CARTESIAN_POINT ( 'NONE',  ( -1.926257025242585782E-15, 196.0906250006145228, -31.45816453501075927 ) ) ;
#12483=CARTESIAN_POINT ( 'NONE',  ( 26.75643035624999655, 240.5218750006145001, -7.049594010296217766E-16 ) ) ;
#12487=CARTESIAN_POINT ( 'NONE',  ( 15.24356964374999990, 248.0593750006145228, 0.000000000000000000 ) ) ;
#12490=CARTESIAN_POINT ( 'NONE',  ( 22.60769515458672885, 243.1736538117966973, -5.999999999999998224 ) ) ;
#12495=CARTESIAN_POINT ( 'NONE',  ( 18.12178482187500350, 239.9218750006145058, 4.985214923628407568 ) ) ;
#12514=CARTESIAN_POINT ( 'NONE',  ( 26.75643035624999655, 249.1843750006145228, -7.049594010296217766E-16 ) ) ;
#12519=CARTESIAN_POINT ( 'NONE',  ( -1.926257025242585782E-15, 199.7468750006145513, -31.45816453501076637 ) ) ;
#12528=CARTESIAN_POINT ( 'NONE',  ( 26.75643035624999655, 247.7593750006145399, -3.323476615752271712 ) ) ;
#12534=VERTEX_POINT ( 'NONE', #18294 ) ;
#12542=CARTESIAN_POINT ( 'NONE',  ( 23.87821517812499650, 246.8968750006145285, -4.985214923628404904 ) ) ;
#12543=AXIS2_PLACEMENT_3D ( 'NONE', #21734, #25812, #19591 ) ;
#12548=EDGE_LOOP ( 'NONE', ( #29374, #6944, #27249, #898 ) ) ;
#12553=CARTESIAN_POINT ( 'NONE',  ( 18.00000000000000355, 249.2312500012290570, 5.196152422706632912 ) ) ;
#12563=CARTESIAN_POINT ( 'NONE',  ( 27.24356964374999635, 199.2218750006145456, -15.72908226750539029 ) ) ;
#12569=VERTEX_POINT ( 'NONE', #12405 ) ;
#12570=CARTESIAN_POINT ( 'NONE',  ( 21.00000000000000000, 243.4187500012290286, 6.928203230275506996 ) ) ;
#12578=CARTESIAN_POINT ( 'NONE',  ( 15.24356964374999990, 243.4468750006145115, 0.000000000000000000 ) ) ;
#12582=PRESENTATION_STYLE_ASSIGNMENT (( #17904 ) ) ;
#12588=FACE_OUTER_BOUND ( 'NONE', #20621, .T. ) ;
#12602=CARTESIAN_POINT ( 'NONE',  ( -4.500000000000001776, 227.8255434699758837, -2.500000000000000000 ) ) ;
#12604=DIRECTION ( 'NONE',  ( -0.000000000000000000, 1.000000000000000000, -0.000000000000000000 ) ) ;
#12607=CARTESIAN_POINT ( 'NONE',  ( 15.24356964374999990, 247.5718750006145399, -3.323476615752268604 ) ) ;
#12620=EDGE_LOOP ( 'NONE', ( #25163, #4640, #1879, #13089 ) ) ;
#12621=CARTESIAN_POINT ( 'NONE',  ( 7.234628195640322446, 196.6450961906613770, 26.99999999999999645 ) ) ;
#12629=CARTESIAN_POINT ( 'NONE',  ( 15.84454946586467194, 211.9332939503076148, 5.693556627483092214 ) ) ;
#12637=CARTESIAN_POINT ( 'NONE',  ( 24.00000000000000000, 247.0000000000000000, 5.196152422706629359 ) ) ;
#12638=CARTESIAN_POINT ( 'NONE',  ( 13.62178482187501416, 198.6031250006145399, 23.59362340125806767 ) ) ;
#12645=CARTESIAN_POINT ( 'NONE',  ( -3.253724281355068545E-15, 197.6374999999999602, -27.00000000000000000 ) ) ;
#12651=CARTESIAN_POINT ( 'NONE',  ( 21.00000000000000000, 240.7187500012290400, 5.999999999999998224 ) ) ;
#12656=DIRECTION ( 'NONE',  ( -0.000000000000000000, 1.000000000000000000, -0.000000000000000000 ) ) ;
#12663=CARTESIAN_POINT ( 'NONE',  ( 18.00000000000000000, 246.7750000000000057, -5.196152422706630247 ) ) ;
#12664=CARTESIAN_POINT ( 'NONE',  ( 27.24356964374999279, 196.4656250006145797, -15.72908226750539207 ) ) ;
#12670=CARTESIAN_POINT ( 'NONE',  ( -27.24356964375000345, 195.3031250006145285, 0.000000000000000000 ) ) ;
#12674=CARTESIAN_POINT ( 'NONE',  ( 26.75643035624999655, 245.0968750006145456, 3.323476615752267715 ) ) ;
#12680=PLANE ( 'NONE',  #28280 ) ;
#12695=CARTESIAN_POINT ( 'NONE',  ( 18.12178482187499640, 249.3343750006145285, -4.985214923628404904 ) ) ;
#12709=ORIENTED_EDGE ( 'NONE', *, *, #25346, .F. ) ;
#12710=CARTESIAN_POINT ( 'NONE',  ( 21.00000000000000000, 247.6093750006145342, 6.646953231504538984 ) ) ;
#12715=EDGE_CURVE ( 'NONE', #20600, #29886, #6727, .T. ) ;
#12728=CARTESIAN_POINT ( 'NONE',  ( 23.87821517812499650, 247.3468750006144887, -4.985214923628404904 ) ) ;
#12735=CARTESIAN_POINT ( 'NONE',  ( 26.99999999999999645, 247.9937500012290457, 3.464101615137751278 ) ) ;
#12742=UNCERTAINTY_MEASURE_WITH_UNIT (LENGTH_MEASURE( 1.000000000000000082E-05 ), #3858, 'distance_accuracy_value', 'NONE');
#12750=CARTESIAN_POINT ( 'NONE',  ( 13.62178482187499640, 199.2593750006145399, -23.59362340125807123 ) ) ;
#12752=PLANE ( 'NONE',  #10995 ) ;
#12756=CARTESIAN_POINT ( 'NONE',  ( 26.99999999999999645, 243.9812500012290570, -7.347880794884117764E-16 ) ) ;
#12759=CARTESIAN_POINT ( 'NONE',  ( 13.62178482187501416, 199.5031250006145456, 23.59362340125806767 ) ) ;
#12765=CARTESIAN_POINT ( 'NONE',  ( 15.24356964374999990, 245.2093750006145285, -3.323476615752268604 ) ) ;
#12781=CARTESIAN_POINT ( 'NONE',  ( 20.99999999999995381, 244.3187500012290627, 5.999999999999998224 ) ) ;
#12787=CYLINDRICAL_SURFACE ( 'NONE', #21325, 5.999999999999999112 ) ;
#12793=CARTESIAN_POINT ( 'NONE',  ( 26.75643035624999655, 244.2718750006145001, -3.323476615752271268 ) ) ;
#12803=ORIENTED_EDGE ( 'NONE', *, *, #1726, .T. ) ;
#12812=CARTESIAN_POINT ( 'NONE',  ( -27.00000000000000355, 197.2624999999999886, -15.58845726811989429 ) ) ;
#12822=CARTESIAN_POINT ( 'NONE',  ( -13.62178482187500528, 199.2781250006145228, -23.59362340125807123 ) ) ;
#12838=CARTESIAN_POINT ( 'NONE',  ( 0.000000000000000000, 202.0000000000000000, 0.000000000000000000 ) ) ;
#12847=CARTESIAN_POINT ( 'NONE',  ( -7.234628195640263826, 195.5200961906613770, -27.00000000000003553 ) ) ;
#12850=CARTESIAN_POINT ( 'NONE',  ( 21.00000000000000000, 245.3875000000000455, -6.928203230275506996 ) ) ;
#12851=CARTESIAN_POINT ( 'NONE',  ( 27.24356964375000345, 195.0781250006145342, -3.336375036156643733E-15 ) ) ;
#12855=VERTEX_POINT ( 'NONE', #15824 ) ;
#12857=CARTESIAN_POINT ( 'NONE',  ( -13.50000000000000533, 197.7875000012290627, -23.38268590217984411 ) ) ;
#12858=CARTESIAN_POINT ( 'NONE',  ( 21.00000000000000000, 240.8593750006145342, 6.646953231504538984 ) ) ;
#12863=CARTESIAN_POINT ( 'NONE',  ( 15.24356964375000167, 244.0468750006145342, 3.323476615752272600 ) ) ;
#12865=CARTESIAN_POINT ( 'NONE',  ( 26.99999999999999645, 243.1187500012290172, -3.464101615137755275 ) ) ;
#12869=CARTESIAN_POINT ( 'NONE',  ( 7.234628195640337545, 198.0674038105676971, -26.99999999999999289 ) ) ;
#12881=CARTESIAN_POINT ( 'NONE',  ( 0.000000000000000000, 202.0000000000000000, 0.000000000000000000 ) ) ;
#12884=DIRECTION ( 'NONE',  ( 1.000000000000000000, 0.000000000000000000, 0.000000000000000000 ) ) ;
#12885=CARTESIAN_POINT ( 'NONE',  ( 18.12178482187499640, 249.7843750006145456, -4.985214923628404904 ) ) ;
#12886=ORIENTED_EDGE ( 'NONE', *, *, #33509, .T. ) ;
#12891=CARTESIAN_POINT ( 'NONE',  ( 20.00041297495057080, 239.8598985277379256, -5.668978411116884608 ) ) ;
#12894=CARTESIAN_POINT ( 'NONE',  ( 21.00000000000000000, 242.0968750006145456, -6.646953231504538984 ) ) ;
#12900=ORIENTED_EDGE ( 'NONE', *, *, #30304, .F. ) ;
#12902=CARTESIAN_POINT ( 'NONE',  ( 18.12178482187499640, 247.8718750006145228, -4.985214923628404904 ) ) ;
#12910=MECHANICAL_DESIGN_GEOMETRIC_PRESENTATION_REPRESENTATION('',(#33498),#18381);
#12911=ORIENTED_EDGE ( 'NONE', *, *, #26308, .T. ) ;
#12917=CARTESIAN_POINT ( 'NONE',  ( 18.12178482187499640, 246.5218750006145001, -4.985214923628404904 ) ) ;
#12940=CARTESIAN_POINT ( 'NONE',  ( -13.50000000000000533, 196.3249999999999886, -23.38268590217984411 ) ) ;
#12943=LINE ( 'NONE', #24504, #15127 ) ;
#12945=EDGE_LOOP ( 'NONE', ( #10892, #34753, #5014, #10146 ) ) ;
#12946=CARTESIAN_POINT ( 'NONE',  ( 18.00000000000000355, 244.2812500012290400, 5.196152422706632912 ) ) ;
#12953=ORIENTED_EDGE ( 'NONE', *, *, #8031, .T. ) ;
#12955=CARTESIAN_POINT ( 'NONE',  ( 26.75643035624999655, 244.9843750006145058, 3.323476615752267715 ) ) ;
#12959=AXIS2_PLACEMENT_3D ( 'NONE', #1413, #9396, #659 ) ;
#12973=EDGE_CURVE ( 'NONE', #483, #20369, #8549, .T. ) ;
#12976=DIRECTION ( 'NONE',  ( 0.000000000000000000, 1.000000000000000000, 0.000000000000000000 ) ) ;
#12980=CARTESIAN_POINT ( 'NONE',  ( 0.000000000000000000, 210.0000000000000284, -27.00000000000000000 ) ) ;
#12985=DIRECTION ( 'NONE',  ( -0.000000000000000000, 1.000000000000000000, -0.000000000000000000 ) ) ;
#12987=CARTESIAN_POINT ( 'NONE',  ( 18.12178482187500350, 244.9843750006145342, 4.985214923628407568 ) ) ;
#12990=( BOUNDED_CURVE ( )  B_SPLINE_CURVE ( 2, ( #3130, #26247, #6542, #18115, #29657, #3693, #15261, #8639, #17366 ),
 .UNSPECIFIED., .F., .F. ) 
 B_SPLINE_CURVE_WITH_KNOTS ( ( 3, 2, 2, 2, 3 ),
 ( 0.7708333333333333703, 0.7777777777777777901, 0.7916666666666666297, 0.8055555555555555802, 0.8125000000000000000 ),
 .UNSPECIFIED. ) 
 CURVE ( )  GEOMETRIC_REPRESENTATION_ITEM ( )  RATIONAL_B_SPLINE_CURVE ( ( 0.9330127018922192983, 0.9330127018922198534, 1.000000000000000000, 0.8660254037844387076, 1.000000000000000000, 0.8660254037844387076, 1.000000000000000000, 0.9330127018922194093, 0.9330127018922194093 ) ) 
 REPRESENTATION_ITEM ( '' )  );
#12999=VERTEX_POINT ( 'NONE', #26161 ) ;
#13016=PRODUCT_CONTEXT ( 'NONE', #346, 'mechanical' ) ;
#13018=CARTESIAN_POINT ( 'NONE',  ( 27.24356964375000345, 198.6781250006145569, -3.336375036156643733E-15 ) ) ;
#13022=LINE ( 'NONE', #36309, #30757 ) ;
#13035=CARTESIAN_POINT ( 'NONE',  ( 26.99999999999999645, 199.3625000000000114, -15.58845726811990495 ) ) ;
#13036=CARTESIAN_POINT ( 'NONE',  ( 20.99999999999999645, 185.0294372515228645, 0.000000000000000000 ) ) ;
#13045=CARTESIAN_POINT ( 'NONE',  ( 15.00000000000000178, 245.0875000000000057, 3.464101615137757051 ) ) ;
#13051=CARTESIAN_POINT ( 'NONE',  ( 5.727106289114498080E-15, 197.9750000012290343, 31.17691453623979214 ) ) ;
#13052=CARTESIAN_POINT ( 'NONE',  ( 15.00000000000000000, 248.6687500012290286, -3.464101615137752610 ) ) ;
#13056=CARTESIAN_POINT ( 'NONE',  ( 21.00000000000000000, 246.1468750006145285, -6.646953231504538984 ) ) ;
#13058=FACE_OUTER_BOUND ( 'NONE', #11816, .T. ) ;
#13062=CARTESIAN_POINT ( 'NONE',  ( -13.62178482187500528, 199.7843750006145456, -23.59362340125807123 ) ) ;
#13066=EDGE_CURVE ( 'NONE', #2189, #35593, #16267, .T. ) ;
#13074=CARTESIAN_POINT ( 'NONE',  ( 20.99999999999999645, 185.0294372515228645, 0.000000000000000000 ) ) ;
#13078=CARTESIAN_POINT ( 'NONE',  ( 18.12178482187500350, 240.8218750006145399, 4.985214923628407568 ) ) ;
#13079=VERTEX_POINT ( 'NONE', #17460 ) ;
#13082=CARTESIAN_POINT ( 'NONE',  ( 27.24356964375000345, 198.2843750006145456, -3.336375036156643733E-15 ) ) ;
#13083=DIRECTION ( 'NONE',  ( -0.000000000000000000, 1.000000000000000000, -0.000000000000000000 ) ) ;
#13084=CARTESIAN_POINT ( 'NONE',  ( 21.00000000000000000, 239.8187500012290059, 5.999999999999998224 ) ) ;
#13085=CARTESIAN_POINT ( 'NONE',  ( 15.24356964375000167, 243.5968750006144887, 3.323476615752272600 ) ) ;
#13089=ORIENTED_EDGE ( 'NONE', *, *, #198, .F. ) ;
#13090=CARTESIAN_POINT ( 'NONE',  ( 21.00000000000000000, 244.0093750006145115, 6.646953231504538984 ) ) ;
#13095=ORIENTED_EDGE ( 'NONE', *, *, #6911, .F. ) ;
#13102=AXIS2_PLACEMENT_3D ( 'NONE', #14607, #11945, #20112 ) ;
#13104=CARTESIAN_POINT ( 'NONE',  ( 18.12178482187500350, 247.5718750006145115, 4.985214923628407568 ) ) ;
#13113=VECTOR ( 'NONE', #35467, 1000.000000000000000 ) ;
#13114=ADVANCED_FACE ( 'NONE', ( #11389 ), #29377, .F. ) ;
#13126=CARTESIAN_POINT ( 'NONE',  ( 13.62178482187501416, 196.8593750006145342, 23.59362340125806767 ) ) ;
#13127=CARTESIAN_POINT ( 'NONE',  ( 2.999999999999997335, 244.5000000000000000, 2.500000000000000000 ) ) ;
#13131=CARTESIAN_POINT ( 'NONE',  ( 15.00000000000000000, 243.3062500012290457, 0.000000000000000000 ) ) ;
#13134=CARTESIAN_POINT ( 'NONE',  ( 15.00000000000000000, 242.7625000000000171, -3.464101615137752610 ) ) ;
#13141=EDGE_CURVE ( 'NONE', #11399, #3975, #26416, .T. ) ;
#13154=DIRECTION ( 'NONE',  ( 0.000000000000000000, 0.000000000000000000, 1.000000000000000000 ) ) ;
#13158=CARTESIAN_POINT ( 'NONE',  ( -27.88991936466936750, 208.9463986166298639, -7.947561165778700421 ) ) ;
#13167=CARTESIAN_POINT ( 'NONE',  ( 15.24356964375000167, 248.5468750006145342, 3.323476615752272600 ) ) ;
#13169=CARTESIAN_POINT ( 'NONE',  ( 23.87821517812500005, 244.6093750006145342, 4.985214923628404016 ) ) ;
#13170=ORIENTED_EDGE ( 'NONE', *, *, #18282, .T. ) ;
#13186=CARTESIAN_POINT ( 'NONE',  ( 0.000000000000000000, 210.0000000000000284, 0.000000000000000000 ) ) ;
#13192=EDGE_CURVE ( 'NONE', #9065, #19072, #34172, .T. ) ;
#13193=CARTESIAN_POINT ( 'NONE',  ( -27.00000000000000355, 197.3000000000000114, 0.000000000000000000 ) ) ;
#13194=CARTESIAN_POINT ( 'NONE',  ( 20.21461154673234262, 212.0943692087130614, 5.961323472697788617 ) ) ;
#13196=FACE_OUTER_BOUND ( 'NONE', #34630, .T. ) ;
#13205=CARTESIAN_POINT ( 'NONE',  ( 5.778771075727756162E-15, 195.8656250006145285, 31.45816453501075927 ) ) ;
#13212=CARTESIAN_POINT ( 'NONE',  ( -7.234628195640316228, 197.6575961894323257, -27.00000000000000000 ) ) ;
#13219=CARTESIAN_POINT ( 'NONE',  ( 18.00000000000000355, 246.4749999999999943, 5.196152422706632912 ) ) ;
#13223=CARTESIAN_POINT ( 'NONE',  ( -13.49999999999998401, 199.1750000000000114, 23.38268590217985476 ) ) ;
#13226=CARTESIAN_POINT ( 'NONE',  ( 13.49999999999999645, 199.4000000000000341, -23.38268590217984766 ) ) ;
#13229=CARTESIAN_POINT ( 'NONE',  ( 15.00000000000000000, 241.9000000000000057, 0.000000000000000000 ) ) ;
#13230=ORIENTED_EDGE ( 'NONE', *, *, #37470, .F. ) ;
#13234=CARTESIAN_POINT ( 'NONE',  ( 24.00000000000000000, 246.5499999999999829, 5.196152422706629359 ) ) ;
#13239=VECTOR ( 'NONE', #20641, 1000.000000000000000 ) ;
#13240=VERTEX_POINT ( 'NONE', #10041 ) ;
#13241=CARTESIAN_POINT ( 'NONE',  ( -1.909035429704832693E-15, 199.1000000012290627, -31.17691453623979214 ) ) ;
#13242=FACE_OUTER_BOUND ( 'NONE', #25064, .T. ) ;
#13245=CARTESIAN_POINT ( 'NONE',  ( 18.12178482187499640, 244.3843750006145115, -4.985214923628404904 ) ) ;
#13264=CARTESIAN_POINT ( 'NONE',  ( 18.12178482187500350, 239.9218750006145058, 4.985214923628407568 ) ) ;
#13265=ORIENTED_EDGE ( 'NONE', *, *, #586, .F. ) ;
#13268=CARTESIAN_POINT ( 'NONE',  ( 27.24356964375000700, 198.2468750006145513, 15.72908226750537075 ) ) ;
#13270=CARTESIAN_POINT ( 'NONE',  ( 23.87821517812500005, 243.7093750006145285, 4.985214923628404016 ) ) ;
#13276=CARTESIAN_POINT ( 'NONE',  ( 26.75643035624999655, 243.6718750006145058, -7.049594010296217766E-16 ) ) ;
#13289=CARTESIAN_POINT ( 'NONE',  ( 26.75643035624999655, 246.3718750006145228, -7.049594010296217766E-16 ) ) ;
#13291=CARTESIAN_POINT ( 'NONE',  ( 27.00000000000000000, 202.0000000000000000, 0.000000000000000000 ) ) ;
#13308=CARTESIAN_POINT ( 'NONE',  ( 18.00000000000000355, 245.1250000000000000, 5.196152422706632912 ) ) ;
#13309=CARTESIAN_POINT ( 'NONE',  ( -13.62178482187500528, 198.4343750006145228, -23.59362340125807123 ) ) ;
#13311=CARTESIAN_POINT ( 'NONE',  ( 24.00000000000000000, 242.0499999999999829, 5.196152422706629359 ) ) ;
#13316=CARTESIAN_POINT ( 'NONE',  ( 15.00000000000000000, 240.5687500012290343, -3.464101615137752166 ) ) ;
#13319=DIRECTION ( 'NONE',  ( -1.000000000000000000, -6.123233995736766036E-17, 0.000000000000000000 ) ) ;
#13322=ORIENTED_EDGE ( 'NONE', *, *, #28167, .F. ) ;
#13324=EDGE_CURVE ( 'NONE', #27444, #8598, #511, .T. ) ;
#13346=CARTESIAN_POINT ( 'NONE',  ( 20.99999999999999645, 185.0294372515228645, 5.999999999999999112 ) ) ;
#13347=EDGE_CURVE ( 'NONE', #33209, #3896, #152, .T. ) ;
#13351=DIRECTION ( 'NONE',  ( 0.000000000000000000, 1.000000000000000000, 0.000000000000000000 ) ) ;
#13353=CARTESIAN_POINT ( 'NONE',  ( 15.24356964375000167, 246.7468750006145228, 3.323476615752272600 ) ) ;
#13355=CARTESIAN_POINT ( 'NONE',  ( 23.87821517812500005, 243.2593750006145399, 4.985214923628404016 ) ) ;
#13358=CARTESIAN_POINT ( 'NONE',  ( 26.99999999999999645, 249.4187500012290286, -3.464101615137755275 ) ) ;
#13370=CARTESIAN_POINT ( 'NONE',  ( 18.00000000000000355, 242.0312500012290400, 5.196152422706632912 ) ) ;
#13377=CARTESIAN_POINT ( 'NONE',  ( 6.642437016334202582, 215.3840861188750466, 2.655215585727055849 ) ) ;
#13379=CARTESIAN_POINT ( 'NONE',  ( 13.50000000000001421, 197.0000000000000000, 23.38268590217984055 ) ) ;
#13386=CARTESIAN_POINT ( 'NONE',  ( 13.62178482187501416, 196.3531250006145115, 23.59362340125806767 ) ) ;
#13398=ADVANCED_FACE ( 'NONE', ( #8876 ), #17233, .F. ) ;
#13401=CARTESIAN_POINT ( 'NONE',  ( 21.00000000000000000, 246.5124999999999602, 5.999999999999998224 ) ) ;
#13409=CARTESIAN_POINT ( 'NONE',  ( -3.253724281355068545E-15, 198.6500000012290172, -27.00000000000000000 ) ) ;
#13410=EDGE_CURVE ( 'NONE', #29886, #7355, #19921, .T. ) ;
#13411=VERTEX_POINT ( 'NONE', #11164 ) ;
#13415=CARTESIAN_POINT ( 'NONE',  ( 23.99999999999999645, 243.1000000000000227, -5.196152422706631135 ) ) ;
#13419=EDGE_LOOP ( 'NONE', ( #29394, #5164, #11944, #37187 ) ) ;
#13421=CARTESIAN_POINT ( 'NONE',  ( 5.727106289114498080E-15, 198.4250000012290229, 31.17691453623979214 ) ) ;
#13425=CARTESIAN_POINT ( 'NONE',  ( 23.87821517812500005, 245.9593750006145569, 4.985214923628404016 ) ) ;
#13427=CARTESIAN_POINT ( 'NONE',  ( 0.000000000000000000, 0.000000000000000000, 2.500000000000000000 ) ) ;
#13431=CARTESIAN_POINT ( 'NONE',  ( 13.62178482187501416, 197.7593750006145399, 23.59362340125806767 ) ) ;
#13440=VECTOR ( 'NONE', #8454, 1000.000000000000000 ) ;
#13446=EDGE_CURVE ( 'NONE', #21774, #25338, #6219, .T. ) ;
#13450=ORIENTED_EDGE ( 'NONE', *, *, #5092, .F. ) ;
#13453=CARTESIAN_POINT ( 'NONE',  ( 13.62178482187501416, 196.8593750006145342, 23.59362340125806767 ) ) ;
#13454=FACE_BOUND ( 'NONE', #4038, .T. ) ;
#13457=CARTESIAN_POINT ( 'NONE',  ( 26.75643035624999655, 243.7468750006145228, 3.323476615752267715 ) ) ;
#13463=CARTESIAN_POINT ( 'NONE',  ( 15.24356964375000167, 244.3843750006145115, 3.323476615752272600 ) ) ;
#13467=CARTESIAN_POINT ( 'NONE',  ( 26.99999999999999645, 244.3374999999999773, 3.464101615137751278 ) ) ;
#13475=CARTESIAN_POINT ( 'NONE',  ( 20.99999999999999645, 243.3343750006145285, -6.646953231504538984 ) ) ;
#13476=CARTESIAN_POINT ( 'NONE',  ( -13.49999999999998401, 197.4875000012290229, 23.38268590217985476 ) ) ;
#13493=CARTESIAN_POINT ( 'NONE',  ( -1.926257025242585782E-15, 198.8468750006145740, -31.45816453501075927 ) ) ;
#13498=VERTEX_POINT ( 'NONE', #12280 ) ;
#13499=CIRCLE ( 'NONE', #18441, 5.999999999999999112 ) ;
#13500=CARTESIAN_POINT ( 'NONE',  ( 18.00000000000000355, 242.0312500012290400, 5.196152422706632912 ) ) ;
#13503=CARTESIAN_POINT ( 'NONE',  ( 5.778771075727756162E-15, 198.5656250006145171, 31.45816453501075927 ) ) ;
#13506=AXIS2_PLACEMENT_3D ( 'NONE', #12277, #18355, #29904 ) ;
#13511=EDGE_CURVE ( 'NONE', #3008, #2146, #27652, .T. ) ;
#13520=CARTESIAN_POINT ( 'NONE',  ( -14.50000000000000000, 215.7563705986615901, -5.555555555555558023 ) ) ;
#13528=ADVANCED_FACE ( 'NONE', ( #6408 ), #26871, .F. ) ;
#13531=EDGE_LOOP ( 'NONE', ( #20706, #28086, #22199, #20132 ) ) ;
#13536=CARTESIAN_POINT ( 'NONE',  ( 27.00000000000000355, 195.3875000012290286, -3.306546357697854128E-15 ) ) ;
#13541=CARTESIAN_POINT ( 'NONE',  ( 26.75643035624999655, 248.7343750006145342, -7.049594010296217766E-16 ) ) ;
#13543=CARTESIAN_POINT ( 'NONE',  ( 20.99999999999999645, 242.9968750006145513, -6.646953231504538984 ) ) ;
#13546=CARTESIAN_POINT ( 'NONE',  ( 15.00000000000000000, 248.2187500012290684, -3.464101615137752166 ) ) ;
#13558=AXIS2_PLACEMENT_3D ( 'NONE', #17446, #14409, #14971 ) ;
#13559=CARTESIAN_POINT ( 'NONE',  ( 17.48528137423856066, 206.4852813742385820, -5.999999999999995559 ) ) ;
#13560=LINE ( 'NONE', #22099, #10550 ) ;
#13561=CARTESIAN_POINT ( 'NONE',  ( 26.75643035624999655, 248.6593750006145171, -3.323476615752271712 ) ) ;
#13566=CARTESIAN_POINT ( 'NONE',  ( 15.00000000000045119, 215.9999999999999716, 0.1308996912579823979 ) ) ;
#13568=CARTESIAN_POINT ( 'NONE',  ( 7.234628195640322446, 196.9825961894323427, 26.99999999999999645 ) ) ;
#13575=CARTESIAN_POINT ( 'NONE',  ( -27.24356964375000345, 196.6531250006145513, 0.000000000000000000 ) ) ;
#13597=CARTESIAN_POINT ( 'NONE',  ( -27.00000000000000355, 198.6500000000000341, 0.000000000000000000 ) ) ;
#13601=CARTESIAN_POINT ( 'NONE',  ( 7.234628195640322446, 198.4450961906613600, 26.99999999999999645 ) ) ;
#13609=CARTESIAN_POINT ( 'NONE',  ( 23.99999999999999645, 242.6500000000000057, -5.196152422706631135 ) ) ;
#13611=EDGE_CURVE ( 'NONE', #37310, #19674, #3172, .T. ) ;
#13616=CARTESIAN_POINT ( 'NONE',  ( 13.50000000000001421, 197.5625000012290400, 23.38268590217984055 ) ) ;
#13617=CARTESIAN_POINT ( 'NONE',  ( -27.24356964375000345, 199.8031250006145285, 0.000000000000000000 ) ) ;
#13620=CARTESIAN_POINT ( 'NONE',  ( 26.75643035624999655, 243.7468750006145228, 3.323476615752267715 ) ) ;
#13627=CARTESIAN_POINT ( 'NONE',  ( -27.24356964374999635, 198.9968750006145228, 15.72908226750539384 ) ) ;
#13629=B_SPLINE_CURVE_WITH_KNOTS ( 'NONE', 3,
 ( #34868, #8541, #8910, #20107 ),
 .UNSPECIFIED., .F., .F.,
 ( 4, 4 ),
 ( 0.000000000000000000, 1.000000000000000000 ),
 .UNSPECIFIED. ) ;
#13632=DIRECTION ( 'NONE',  ( 4.818676322157800087E-17, -1.000000000000000000, 5.329070518200755338E-15 ) ) ;
#13640=CARTESIAN_POINT ( 'NONE',  ( 20.99999999999999645, 249.6625000000000512, 5.999999999999998224 ) ) ;
#13644=CARTESIAN_POINT ( 'NONE',  ( -13.62178482187500528, 197.9843750006145626, -23.59362340125807123 ) ) ;
#13648=CARTESIAN_POINT ( 'NONE',  ( 21.00000000000000000, 249.6625000000000227, 6.928203230275506996 ) ) ;
#13655=CARTESIAN_POINT ( 'NONE',  ( 26.75643035624999655, 244.5718750006145115, -7.049594010296217766E-16 ) ) ;
#13657=ADVANCED_FACE ( 'NONE', ( #34001 ), #2158, .F. ) ;
#13671=CARTESIAN_POINT ( 'NONE',  ( 26.75643035624999655, 245.0593750006144944, -3.323476615752271268 ) ) ;
#13674=CARTESIAN_POINT ( 'NONE',  ( -7.234628195640316228, 197.3200961906614168, -27.00000000000000000 ) ) ;
#13687=DIRECTION ( 'NONE',  ( -0.000000000000000000, 1.000000000000000000, -0.000000000000000000 ) ) ;
#13691=CARTESIAN_POINT ( 'NONE',  ( -1.926257025242585782E-15, 197.9468750006145399, -31.45816453501075927 ) ) ;
#13695=ORIENTED_EDGE ( 'NONE', *, *, #1699, .F. ) ;
#13696=CARTESIAN_POINT ( 'NONE',  ( 15.00000000000000000, 241.5062500012290627, 0.000000000000000000 ) ) ;
#13699=CARTESIAN_POINT ( 'NONE',  ( -27.24356964375000345, 198.9031250006145228, 0.000000000000000000 ) ) ;
#13725=( BOUNDED_CURVE ( )  B_SPLINE_CURVE ( 2, ( #23151, #20311, #17276, #31484, #11206, #34693, #5884, #11392, #9116 ),
 .UNSPECIFIED., .F., .F. ) 
 B_SPLINE_CURVE_WITH_KNOTS ( ( 3, 2, 2, 2, 3 ),
 ( 0.3586956521739130266, 0.3623188405797101441, 0.3695652173913043237, 0.3768115942028985588, 0.3804347826086956763 ),
 .UNSPECIFIED. ) 
 CURVE ( )  GEOMETRIC_REPRESENTATION_ITEM ( )  RATIONAL_B_SPLINE_CURVE ( ( 0.9330127018922191873, 0.9330127018922187432, 1.000000000000000000, 0.8660254037844387076, 1.000000000000000000, 0.8660254037844387076, 1.000000000000000000, 0.9330127018922188542, 0.9330127018922194093 ) ) 
 REPRESENTATION_ITEM ( '' )  );
#13732=CARTESIAN_POINT ( 'NONE',  ( 20.99999999999999645, 250.0000000000000000, 0.000000000000000000 ) ) ;
#13734=CARTESIAN_POINT ( 'NONE',  ( 20.99999999999998579, 247.6374999999999886, -5.999999999999997335 ) ) ;
#13735=CARTESIAN_POINT ( 'NONE',  ( 26.75643035624999655, 247.8343750006145285, -7.049594010296217766E-16 ) ) ;
#13737=CARTESIAN_POINT ( 'NONE',  ( 15.24356964375000167, 242.6968750006145399, 3.323476615752272600 ) ) ;
#13742=CARTESIAN_POINT ( 'NONE',  ( 15.00000000000000178, 247.8437500012290684, 3.464101615137757051 ) ) ;
#13748=ORIENTED_EDGE ( 'NONE', *, *, #11515, .F. ) ;
#13753=CYLINDRICAL_SURFACE ( 'NONE', #19131, 5.999999999999999112 ) ;
#13754=CARTESIAN_POINT ( 'NONE',  ( 26.99999999999999645, 247.9375000000000000, 3.464101615137751278 ) ) ;
#13755=CARTESIAN_POINT ( 'NONE',  ( 18.12178482187500350, 248.9218750006145342, 4.985214923628407568 ) ) ;
#13758=CARTESIAN_POINT ( 'NONE',  ( 14.82946893053495252, 216.1705310694576099, -0.5774388102985152926 ) ) ;
#13766=CARTESIAN_POINT ( 'NONE',  ( 5.778771075727756162E-15, 196.3156250006145171, 31.45816453501075927 ) ) ;
#13769=VECTOR ( 'NONE', #16737, 1000.000000000000000 ) ;
#13771=CARTESIAN_POINT ( 'NONE',  ( 24.00000000000000000, 248.8562500012290570, 5.196152422706629359 ) ) ;
#13785=CARTESIAN_POINT ( 'NONE',  ( 13.50000000000001421, 197.9000000000000341, 23.38268590217984055 ) ) ;
#13789=CARTESIAN_POINT ( 'NONE',  ( -29.00000000000002487, 210.0000000000000284, -8.000000000000000000 ) ) ;
#13797=CARTESIAN_POINT ( 'NONE',  ( 24.00000000000000000, 244.2999999999999829, 5.196152422706629359 ) ) ;
#13798=CARTESIAN_POINT ( 'NONE',  ( 20.99999999999999645, 246.1187500012290457, 5.999999999999998224 ) ) ;
#13802=CARTESIAN_POINT ( 'NONE',  ( -27.00000000000000355, 195.6125000012290513, 0.000000000000000000 ) ) ;
#13806=CARTESIAN_POINT ( 'NONE',  ( 26.75643035624999655, 242.0218750006145285, -3.323476615752271712 ) ) ;
#13814=CARTESIAN_POINT ( 'NONE',  ( 27.24356964375000345, 199.1843750006145228, -3.336375036156643733E-15 ) ) ;
#13817=CARTESIAN_POINT ( 'NONE',  ( 0.000000000000000000, 210.0000000000000284, 0.000000000000000000 ) ) ;
#13818=CARTESIAN_POINT ( 'NONE',  ( 22.60769515458672174, 245.1825961894323314, 6.000000000000004441 ) ) ;
#13820=DIRECTION ( 'NONE',  ( -0.000000000000000000, 1.000000000000000000, -0.000000000000000000 ) ) ;
#13828=CARTESIAN_POINT ( 'NONE',  ( 26.99999999999999645, 248.4437500012290343, 3.464101615137751278 ) ) ;
#13829=ORIENTED_EDGE ( 'NONE', *, *, #5043, .T. ) ;
#13833=CARTESIAN_POINT ( 'NONE',  ( -13.62178482187498396, 196.7843750006145456, 23.59362340125808188 ) ) ;
#13837=CARTESIAN_POINT ( 'NONE',  ( 18.12178482187499640, 240.7843750006145171, -4.985214923628404904 ) ) ;
#13841=ORIENTED_EDGE ( 'NONE', *, *, #6679, .T. ) ;
#13843=CARTESIAN_POINT ( 'NONE',  ( 15.24356964374999990, 244.3093750006145228, -3.323476615752268604 ) ) ;
#13849=VECTOR ( 'NONE', #9816, 1000.000000000000000 ) ;
#13855=CARTESIAN_POINT ( 'NONE',  ( 18.12178482187499640, 244.2718750006145001, -4.985214923628404904 ) ) ;
#13856=DIRECTION ( 'NONE',  ( -1.000000000000000000, -4.130293990420971855E-17, 0.000000000000000000 ) ) ;
#13862=CARTESIAN_POINT ( 'NONE',  ( -13.50000000000000533, 199.4750000000000227, -23.38268590217984411 ) ) ;
#13876=CARTESIAN_POINT ( 'NONE',  ( 27.24356964374999635, 195.1718750006145342, -15.72908226750539029 ) ) ;
#13878=ADVANCED_FACE ( 'NONE', ( #9515 ), #21088, .F. ) ;
#13883=CARTESIAN_POINT ( 'NONE',  ( 21.00000000000000000, 242.7437500012290457, -6.928203230275506996 ) ) ;
#13889=ORIENTED_EDGE ( 'NONE', *, *, #10802, .F. ) ;
#13918=CARTESIAN_POINT ( 'NONE',  ( 26.75643035624999655, 246.9343750006145228, -7.049594010296217766E-16 ) ) ;
#13920=CARTESIAN_POINT ( 'NONE',  ( 20.99999999999999645, 242.3218750006145399, 6.646953231504538984 ) ) ;
#13923=CARTESIAN_POINT ( 'NONE',  ( 15.00000000000000000, 249.6062500012290570, 0.000000000000000000 ) ) ;
#13928=CARTESIAN_POINT ( 'NONE',  ( 5.649999999999987921, 244.5000000000000000, 5.000000000000000000 ) ) ;
#13936=CARTESIAN_POINT ( 'NONE',  ( 15.00000000000000178, 241.9937500012290457, 3.464101615137757051 ) ) ;
#13937=CARTESIAN_POINT ( 'NONE',  ( 18.12178482187499640, 249.2218750006145171, -4.985214923628404904 ) ) ;
#13940=CARTESIAN_POINT ( 'NONE',  ( 6.017554903305174285, 215.6184169112604536, -2.114697272285170460 ) ) ;
#13942=CARTESIAN_POINT ( 'NONE',  ( 20.99999999999999645, 185.0294372515228645, 0.000000000000000000 ) ) ;
#13943=CIRCLE ( 'NONE', #2430, 7.500000000000000000 ) ;
#13948=( BOUNDED_CURVE ( )  B_SPLINE_CURVE ( 2, ( #22379, #33927, #25578, #28241, #1896, #13467, #10617, #22196, #33744 ),
 .UNSPECIFIED., .F., .F. ) 
 B_SPLINE_CURVE_WITH_KNOTS ( ( 3, 2, 2, 2, 3 ),
 ( 0.5326086956521739468, 0.5362318840579710644, 0.5434782608695651884, 0.5507246376811594235, 0.5543478260869565410 ),
 .UNSPECIFIED. ) 
 CURVE ( )  GEOMETRIC_REPRESENTATION_ITEM ( )  RATIONAL_B_SPLINE_CURVE ( ( 0.9330127018922194093, 0.9330127018922194093, 1.000000000000000000, 0.8660254037844387076, 1.000000000000000000, 0.8660254037844387076, 1.000000000000000000, 0.9330127018922194093, 0.9330127018922194093 ) ) 
 REPRESENTATION_ITEM ( '' )  );
#13950=CARTESIAN_POINT ( 'NONE',  ( -27.24356964374999635, 195.3406250006145513, 15.72908226750539384 ) ) ;
#13954=CARTESIAN_POINT ( 'NONE',  ( 22.60769515458672885, 240.8674038105676516, -5.999999999999998224 ) ) ;
#13966=CARTESIAN_POINT ( 'NONE',  ( 26.99999999999999645, 197.1125000000000398, -15.58845726811990495 ) ) ;
#13970=CARTESIAN_POINT ( 'NONE',  ( 15.24356964374999990, 248.9218750006145626, -3.323476615752268604 ) ) ;
#13977=CARTESIAN_POINT ( 'NONE',  ( 23.99999999999999645, 243.5499999999999829, -5.196152422706631135 ) ) ;
#13981=CARTESIAN_POINT ( 'NONE',  ( 5.727106289114498080E-15, 195.2750000012290172, 31.17691453623979214 ) ) ;
#13985=CARTESIAN_POINT ( 'NONE',  ( 21.00000000000000000, 243.6718750006145058, 6.646953231504538984 ) ) ;
#13988=CARTESIAN_POINT ( 'NONE',  ( 20.00041297495057080, 239.8598985277379256, -5.668978411116884608 ) ) ;
#13994=CARTESIAN_POINT ( 'NONE',  ( -13.62178482187500528, 198.8843750006145399, -23.59362340125807123 ) ) ;
#13997=DIRECTION ( 'NONE',  ( -0.000000000000000000, 1.000000000000000000, -0.000000000000000000 ) ) ;
#14005=EDGE_CURVE ( 'NONE', #32985, #17695, #33954, .T. ) ;
#14007=FACE_OUTER_BOUND ( 'NONE', #36146, .T. ) ;
#14009=EDGE_LOOP ( 'NONE', ( #20570, #33017, #18224, #30435 ) ) ;
#14010=VECTOR ( 'NONE', #6054, 1000.000000000000000 ) ;
#14014=CARTESIAN_POINT ( 'NONE',  ( 20.99999999999999645, 185.0294372515228645, 0.000000000000000000 ) ) ;
#14017=DIRECTION ( 'NONE',  ( -0.000000000000000000, 1.000000000000000000, -0.000000000000000000 ) ) ;
#14018=CARTESIAN_POINT ( 'NONE',  ( 18.12178482187499640, 240.3343750006145285, -4.985214923628404904 ) ) ;
#14019=CARTESIAN_POINT ( 'NONE',  ( 13.62178482187499640, 198.7531250006145456, -23.59362340125807123 ) ) ;
#14025=CARTESIAN_POINT ( 'NONE',  ( 26.75643035624999655, 241.3843750006145399, 3.323476615752267715 ) ) ;
#14032=AXIS2_PLACEMENT_3D ( 'NONE', #28306, #13351, #19614 ) ;
#14036=CARTESIAN_POINT ( 'NONE',  ( 18.12178482187500350, 243.5218750006145001, 4.985214923628407568 ) ) ;
#14037=VECTOR ( 'NONE', #21522, 1000.000000000000000 ) ;
#14038=EDGE_CURVE ( 'NONE', #12999, #29663, #24008, .T. ) ;
#14043=CARTESIAN_POINT ( 'NONE',  ( 23.99999999999999645, 240.0062500012290627, -5.196152422706631135 ) ) ;
#14044=CARTESIAN_POINT ( 'NONE',  ( 19.39230484541324273, 244.6924038105676686, 5.999999999999987566 ) ) ;
#14056=CARTESIAN_POINT ( 'NONE',  ( 20.99999999999999289, 244.0937500012290116, -5.999999999999997335 ) ) ;
#14060=CARTESIAN_POINT ( 'NONE',  ( 13.62178482187501416, 196.4093750006145456, 23.59362340125806767 ) ) ;
#14061=CARTESIAN_POINT ( 'NONE',  ( 20.99999999999999289, 244.5437500012290286, -5.999999999999997335 ) ) ;
#14065=CARTESIAN_POINT ( 'NONE',  ( 15.00000000000000000, 241.9562500012290513, 0.000000000000000000 ) ) ;
#14070=ORIENTED_EDGE ( 'NONE', *, *, #9163, .F. ) ;
#14075=LINE ( 'NONE', #36995, #13769 ) ;
#14077=EDGE_CURVE ( 'NONE', #4638, #23066, #8064, .T. ) ;
#14081=ORIENTED_EDGE ( 'NONE', *, *, #31453, .T. ) ;
#14097=CARTESIAN_POINT ( 'NONE',  ( 15.00000000000000000, 240.1187500012290741, -3.464101615137752610 ) ) ;
#14098=CARTESIAN_POINT ( 'NONE',  ( 15.24356964374999990, 245.3218750006145399, -3.323476615752268604 ) ) ;
#14100=CARTESIAN_POINT ( 'NONE',  ( 15.24356964374999990, 241.3093750006145228, 0.000000000000000000 ) ) ;
#14103=LINE ( 'NONE', #14289, #6899 ) ;
#14104=CARTESIAN_POINT ( 'NONE',  ( 15.00000000000000178, 248.2937500012290286, 3.464101615137757051 ) ) ;
#14111=ORIENTED_EDGE ( 'NONE', *, *, #22391, .F. ) ;
#14116=DIRECTION ( 'NONE',  ( -0.000000000000000000, 1.000000000000000000, -0.000000000000000000 ) ) ;
#14118=CARTESIAN_POINT ( 'NONE',  ( 15.24356964374999990, 247.9468750006145115, 0.000000000000000000 ) ) ;
#14120=ADVANCED_FACE ( 'NONE', ( #5736 ), #11247, .F. ) ;
#14122=CARTESIAN_POINT ( 'NONE',  ( 15.31535524866706233, 225.1590526702200634, 1.929602858955283162 ) ) ;
#14135=CARTESIAN_POINT ( 'NONE',  ( 20.99999999999999289, 248.8187500012290911, 5.999999999999999112 ) ) ;
#14138=CARTESIAN_POINT ( 'NONE',  ( 15.00000000000000000, 250.0000000000000000, 0.000000000000000000 ) ) ;
#14143=( BOUNDED_CURVE ( )  B_SPLINE_CURVE ( 2, ( #29189, #22780, #29000, #14425, #31853, #26165, #3231, #200, #20120 ),
 .UNSPECIFIED., .F., .F. ) 
 B_SPLINE_CURVE_WITH_KNOTS ( ( 3, 2, 2, 2, 3 ),
 ( 0.4791666666666666852, 0.4861111111111111049, 0.5000000000000000000, 0.5138888888888888395, 0.5208333333333333703 ),
 .UNSPECIFIED. ) 
 CURVE ( )  GEOMETRIC_REPRESENTATION_ITEM ( )  RATIONAL_B_SPLINE_CURVE ( ( 0.9330127018922194093, 0.9330127018922196314, 1.000000000000000000, 0.8660254037844387076, 1.000000000000000000, 0.8660254037844387076, 1.000000000000000000, 0.9330127018922187432, 0.9330127018922192983 ) ) 
 REPRESENTATION_ITEM ( '' )  );
#14148=CARTESIAN_POINT ( 'NONE',  ( 5.727106289114498080E-15, 197.8625000000000114, 31.17691453623979214 ) ) ;
#14151=CARTESIAN_POINT ( 'NONE',  ( 23.87821517812499650, 248.3593750006145342, -4.985214923628404904 ) ) ;
#14158=CARTESIAN_POINT ( 'NONE',  ( 21.00000000000000000, 242.9124999999999943, 6.928203230275506996 ) ) ;
#14164=CARTESIAN_POINT ( 'NONE',  ( -13.50000000000000533, 196.4375000012290400, -23.38268590217984411 ) ) ;
#14165=CARTESIAN_POINT ( 'NONE',  ( 20.99999999999999645, 202.0000000000000000, -5.999999999999999112 ) ) ;
#14168=CARTESIAN_POINT ( 'NONE',  ( 26.75643035624999655, 242.4718750006145456, -3.323476615752271712 ) ) ;
#14176=CARTESIAN_POINT ( 'NONE',  ( -27.24356964374999990, 196.6718750006145342, -15.72908226750537786 ) ) ;
#14183=( GEOMETRIC_REPRESENTATION_CONTEXT ( 3 ) GLOBAL_UNCERTAINTY_ASSIGNED_CONTEXT ( ( #7827 ) ) GLOBAL_UNIT_ASSIGNED_CONTEXT ( ( #25280, #8227, #31337 ) ) REPRESENTATION_CONTEXT ( 'NONE', 'WORKASPACE' ) );
#14193=CARTESIAN_POINT ( 'NONE',  ( 23.99999999999999645, 249.8499999999999943, -5.196152422706631135 ) ) ;
#14198=CARTESIAN_POINT ( 'NONE',  ( 27.24356964375000345, 195.1343750006145399, -3.336375036156643733E-15 ) ) ;
#14201=CARTESIAN_POINT ( 'NONE',  ( 0.000000000000000000, 210.0000000000000284, 0.000000000000000000 ) ) ;
#14202=CARTESIAN_POINT ( 'NONE',  ( 24.00000000000000000, 249.7000000000000171, 5.196152422706629359 ) ) ;
#14203=CARTESIAN_POINT ( 'NONE',  ( -27.24356964375000345, 198.0031250006145456, 0.000000000000000000 ) ) ;
#14208=ORIENTED_EDGE ( 'NONE', *, *, #6109, .T. ) ;
#14209=VERTEX_POINT ( 'NONE', #2530 ) ;
#14211=CARTESIAN_POINT ( 'NONE',  ( 26.75643035624999655, 241.0093750006144830, -3.323476615752271712 ) ) ;
#14219=CARTESIAN_POINT ( 'NONE',  ( 15.24356964374999990, 243.4468750006145115, 0.000000000000000000 ) ) ;
#14224=EDGE_CURVE ( 'NONE', #22557, #22802, #8289, .T. ) ;
#14231=VECTOR ( 'NONE', #6502, 1000.000000000000000 ) ;
#14232=CARTESIAN_POINT ( 'NONE',  ( 20.99999999999995381, 244.3187500012290627, 5.999999999999998224 ) ) ;
#14235=CARTESIAN_POINT ( 'NONE',  ( 23.99999999999999645, 245.8562500012290570, -5.196152422706631135 ) ) ;
#14242=CARTESIAN_POINT ( 'NONE',  ( -27.24356964374999635, 196.2968750006145342, 15.72908226750539384 ) ) ;
#14245=DIRECTION ( 'NONE',  ( -1.000000000000000000, -6.123233995736766036E-17, -0.000000000000000000 ) ) ;
#14248=ORIENTED_EDGE ( 'NONE', *, *, #30942, .F. ) ;
#14250=CARTESIAN_POINT ( 'NONE',  ( 18.12178482187499640, 249.2218750006145171, -4.985214923628404904 ) ) ;
#14257=VECTOR ( 'NONE', #14895, 1000.000000000000000 ) ;
#14262=FACE_OUTER_BOUND ( 'NONE', #15657, .T. ) ;
#14264=CARTESIAN_POINT ( 'NONE',  ( -14.96731853674933888, 195.0000000000000853, 22.75028941543422079 ) ) ;
#14268=ORIENTED_EDGE ( 'NONE', *, *, #27779, .T. ) ;
#14276=ORIENTED_EDGE ( 'NONE', *, *, #27619, .F. ) ;
#14284=CARTESIAN_POINT ( 'NONE',  ( 26.75643035624999655, 245.1718750006145058, -3.323476615752271712 ) ) ;
#14286=CARTESIAN_POINT ( 'NONE',  ( 15.24356964374999990, 240.8593750006145342, 0.000000000000000000 ) ) ;
#14289=CARTESIAN_POINT ( 'NONE',  ( 20.99999999999999645, 185.0294372515228645, -5.999999999999999112 ) ) ;
#14290=CARTESIAN_POINT ( 'NONE',  ( 15.00000000000000178, 245.5937500012290400, 3.464101615137757051 ) ) ;
#14300=VERTEX_POINT ( 'NONE', #3651 ) ;
#14304=FACE_OUTER_BOUND ( 'NONE', #20043, .T. ) ;
#14308=CARTESIAN_POINT ( 'NONE',  ( 14.95628864315848183, 216.0437113568656287, -2.958957796642720961 ) ) ;
#14328=FACE_OUTER_BOUND ( 'NONE', #15276, .T. ) ;
#14332=CARTESIAN_POINT ( 'NONE',  ( -27.00000000000000355, 196.8500000000000227, 0.000000000000000000 ) ) ;
#14335=CARTESIAN_POINT ( 'NONE',  ( 15.24356964374999990, 248.0593750006145228, 0.000000000000000000 ) ) ;
#14343=CARTESIAN_POINT ( 'NONE',  ( 26.99999999999999645, 240.7374999999999829, 3.464101615137751278 ) ) ;
#14344=CARTESIAN_POINT ( 'NONE',  ( 5.438367727407757144E-14, 198.5374999999999943, -27.00000000000000000 ) ) ;
#14349=CARTESIAN_POINT ( 'NONE',  ( 20.99999999999999645, 185.0294372515228645, 5.999999999999999112 ) ) ;
#14350=CARTESIAN_POINT ( 'NONE',  ( -27.00000000000000355, 196.0250000012290457, -15.58845726811989429 ) ) ;
#14355=CARTESIAN_POINT ( 'NONE',  ( 15.24356964374999990, 243.5593750006145228, 0.000000000000000000 ) ) ;
#14362=CARTESIAN_POINT ( 'NONE',  ( 16.25535974507127790, 195.0000000000000000, 21.84619082737673068 ) ) ;
#14363=CARTESIAN_POINT ( 'NONE',  ( -13.62178482187500528, 195.2843750006145456, -23.59362340125807123 ) ) ;
#14366=( BOUNDED_CURVE ( )  B_SPLINE_CURVE ( 2, ( #15587, #35850, #33206, #21475, #33014, #4202, #15779, #24119, #23930 ),
 .UNSPECIFIED., .F., .F. ) 
 B_SPLINE_CURVE_WITH_KNOTS ( ( 3, 2, 2, 2, 3 ),
 ( 0.8152173913043478937, 0.8188405797101449002, 0.8260869565217391353, 0.8333333333333333703, 0.8369565217391303769 ),
 .UNSPECIFIED. ) 
 CURVE ( )  GEOMETRIC_REPRESENTATION_ITEM ( )  RATIONAL_B_SPLINE_CURVE ( ( 0.9330127018922192983, 0.9330127018922202975, 1.000000000000000000, 0.8660254037844387076, 1.000000000000000000, 0.8660254037844387076, 1.000000000000000000, 0.9330127018922202975, 0.9330127018922192983 ) ) 
 REPRESENTATION_ITEM ( '' )  );
#14369=CARTESIAN_POINT ( 'NONE',  ( 3.306546357697853733E-15, 210.0000000000000284, 27.00000000000000000 ) ) ;
#14381=CARTESIAN_POINT ( 'NONE',  ( -27.24356964375000345, 196.2218750006145456, -15.72908226750537786 ) ) ;
#14385=CARTESIAN_POINT ( 'NONE',  ( 26.75643035624999655, 240.1468750006145285, 3.323476615752267715 ) ) ;
#14386=CARTESIAN_POINT ( 'NONE',  ( -27.24356964375000345, 198.4156250006145399, -15.72908226750537786 ) ) ;
#14387=( BOUNDED_CURVE ( )  B_SPLINE_CURVE ( 2, ( #32525, #7141, #6568, #15290, #15858, #21176, #26842, #9971, #32715 ),
 .UNSPECIFIED., .F., .F. ) 
 B_SPLINE_CURVE_WITH_KNOTS ( ( 3, 2, 2, 2, 3 ),
 ( 0.4239130434782608647, 0.4275362318840579823, 0.4347826086956521618, 0.4420289855072463969, 0.4456521739130434590 ),
 .UNSPECIFIED. ) 
 CURVE ( )  GEOMETRIC_REPRESENTATION_ITEM ( )  RATIONAL_B_SPLINE_CURVE ( ( 0.9330127018922194093, 0.9330127018922194093, 1.000000000000000000, 0.8660254037844387076, 1.000000000000000000, 0.8660254037844387076, 1.000000000000000000, 0.9330127018922198534, 0.9330127018922191873 ) ) 
 REPRESENTATION_ITEM ( '' )  );
#14390=EDGE_LOOP ( 'NONE', ( #32318, #14500, #12352, #29293 ) ) ;
#14392=CARTESIAN_POINT ( 'NONE',  ( -13.62178482187498396, 198.9781250006145399, 23.59362340125808188 ) ) ;
#14393=CARTESIAN_POINT ( 'NONE',  ( 26.75643035624999655, 243.1843750006144944, 3.323476615752267715 ) ) ;
#14401=CARTESIAN_POINT ( 'NONE',  ( 20.99999999999999645, 241.7593750006145115, 6.646953231504538984 ) ) ;
#14408=CARTESIAN_POINT ( 'NONE',  ( 24.00000000000000000, 239.8562500012290286, 5.196152422706629359 ) ) ;
#14409=DIRECTION ( 'NONE',  ( -1.000000000000000000, -4.130293990420971855E-17, 0.000000000000000000 ) ) ;
#14422=CARTESIAN_POINT ( 'NONE',  ( 22.60769515458670753, 241.3174038105676686, -6.000000000000011546 ) ) ;
#14423=CARTESIAN_POINT ( 'NONE',  ( 18.00000000000000355, 242.4812500012290570, 5.196152422706632912 ) ) ;
#14424=CARTESIAN_POINT ( 'NONE',  ( 27.24356964375000700, 195.0968750006145456, 15.72908226750537075 ) ) ;
#14425=CARTESIAN_POINT ( 'NONE',  ( -26.99999999999999645, 197.0000000012290116, 15.58845726811991561 ) ) ;
#14431=VERTEX_POINT ( 'NONE', #6500 ) ;
#14432=CARTESIAN_POINT ( 'NONE',  ( 23.87821517812499650, 248.2468750006145228, -4.985214923628404904 ) ) ;
#14442=CARTESIAN_POINT ( 'NONE',  ( 26.75643035624999655, 249.1093750006145058, -3.323476615752271268 ) ) ;
#14444=CARTESIAN_POINT ( 'NONE',  ( -24.36897002145979485, 195.0000000000000284, 12.00491919322965195 ) ) ;
#14449=ORIENTED_EDGE ( 'NONE', *, *, #11549, .T. ) ;
#14457=EDGE_LOOP ( 'NONE', ( #23343, #34011, #17241, #29201, #7127, #23155 ) ) ;
#14465=CARTESIAN_POINT ( 'NONE',  ( 20.99999999999997513, 246.3437500012290684, -5.999999999999999112 ) ) ;
#14466=CARTESIAN_POINT ( 'NONE',  ( 18.12178482187500350, 245.8843750006145115, 4.985214923628407568 ) ) ;
#14468=CARTESIAN_POINT ( 'NONE',  ( 18.12178482187499640, 242.1343750006145115, -4.985214923628404904 ) ) ;
#14473=CARTESIAN_POINT ( 'NONE',  ( 26.99999999999999645, 246.6812500012290457, -7.347880794884117764E-16 ) ) ;
#14486=CARTESIAN_POINT ( 'NONE',  ( 26.75643035624999655, 246.7843750006145171, 3.323476615752267715 ) ) ;
#14489=CARTESIAN_POINT ( 'NONE',  ( 8.278277990405213060, 214.7706457535942661, -3.659938751172172822 ) ) ;
#14499=EDGE_CURVE ( 'NONE', #11470, #1148, #21109, .T. ) ;
#14500=ORIENTED_EDGE ( 'NONE', *, *, #33533, .T. ) ;
#14501=CARTESIAN_POINT ( 'NONE',  ( 26.99999999999999645, 248.9687500012290116, -3.464101615137755275 ) ) ;
#14504=CARTESIAN_POINT ( 'NONE',  ( 15.00000000000000000, 243.2125000000000057, -3.464101615137752610 ) ) ;
#14511=CYLINDRICAL_SURFACE ( 'NONE', #12211, 5.999999999999999112 ) ;
#14513=CARTESIAN_POINT ( 'NONE',  ( 15.00000000000000000, 249.0625000000000000, -3.464101615137752610 ) ) ;
#14515=CARTESIAN_POINT ( 'NONE',  ( 5.727106289114498080E-15, 196.5125000000000171, 31.17691453623979214 ) ) ;
#14518=CARTESIAN_POINT ( 'NONE',  ( 20.99999999999999645, 249.2968750006145342, -6.646953231504538984 ) ) ;
#14521=LINE ( 'NONE', #35156, #14257 ) ;
#14525=CARTESIAN_POINT ( 'NONE',  ( 23.99999999999999645, 240.4000000000000057, -5.196152422706631135 ) ) ;
#14528=ORIENTED_EDGE ( 'NONE', *, *, #14038, .T. ) ;
#14531=CARTESIAN_POINT ( 'NONE',  ( -26.99999999999998934, 195.2000000012290286, 15.58845726811991561 ) ) ;
#14534=VECTOR ( 'NONE', #26960, 1000.000000000000000 ) ;
#14546=CARTESIAN_POINT ( 'NONE',  ( 15.80494806997313439, 195.0000000000000284, 22.17725129625731029 ) ) ;
#14547=CARTESIAN_POINT ( 'NONE',  ( -27.24356964374999635, 194.9468750006145399, 15.72908226750539384 ) ) ;
#14549=EDGE_CURVE ( 'NONE', #3075, #27300, #12943, .T. ) ;
#14557=CARTESIAN_POINT ( 'NONE',  ( 7.234628195640309123, 197.2799038117966859, -27.00000000000000711 ) ) ;
#14558=CIRCLE ( 'NONE', #35735, 28.99999999999999645 ) ;
#14568=CARTESIAN_POINT ( 'NONE',  ( 5.778771075727756162E-15, 195.9218750006145342, 31.45816453501076637 ) ) ;
#14571=CARTESIAN_POINT ( 'NONE',  ( -13.49999999999998401, 198.2750000000000057, 23.38268590217985476 ) ) ;
#14572=CARTESIAN_POINT ( 'NONE',  ( 21.00000000000000000, 249.2125000000000057, 6.928203230275506996 ) ) ;
#14573=CARTESIAN_POINT ( 'NONE',  ( 27.24356964375000345, 199.5781250006145342, -3.336375036156643733E-15 ) ) ;
#14577=ORIENTED_EDGE ( 'NONE', *, *, #15680, .F. ) ;
#14579=CARTESIAN_POINT ( 'NONE',  ( 27.24356964374999635, 199.1656250006145399, -15.72908226750539029 ) ) ;
#14580=CARTESIAN_POINT ( 'NONE',  ( 15.24356964374999990, 241.6468750006145285, 0.000000000000000000 ) ) ;
#14583=CARTESIAN_POINT ( 'NONE',  ( 15.24356964374999990, 247.5718750006145399, -3.323476615752268604 ) ) ;
#14589=CARTESIAN_POINT ( 'NONE',  ( 15.24356964374999990, 242.9968750006145228, 0.000000000000000000 ) ) ;
#14594=EDGE_CURVE ( 'NONE', #21071, #34895, #25976, .T. ) ;
#14605=CARTESIAN_POINT ( 'NONE',  ( 21.00000000000000000, 242.4343750006145228, -6.646953231504538984 ) ) ;
#14607=CARTESIAN_POINT ( 'NONE',  ( -29.00000000000002487, 210.0000000000000000, 0.000000000000000000 ) ) ;
#14611=CARTESIAN_POINT ( 'NONE',  ( 13.62178482187499640, 196.1093750006145342, -23.59362340125807123 ) ) ;
#14612=DIRECTION ( 'NONE',  ( -0.000000000000000000, 1.000000000000000000, -0.000000000000000000 ) ) ;
#14613=CYLINDRICAL_SURFACE ( 'NONE', #35102, 5.999999999999999112 ) ;
#14618=CARTESIAN_POINT ( 'NONE',  ( 21.00000000000000000, 248.2843750006145171, -6.646953231504538984 ) ) ;
#14630=CARTESIAN_POINT ( 'NONE',  ( 15.24356964374999990, 249.2968750006145058, 0.000000000000000000 ) ) ;
#14631=CARTESIAN_POINT ( 'NONE',  ( -24.86337347398900022, 195.0000000000000853, -10.63620294009199441 ) ) ;
#14639=( BOUNDED_CURVE ( )  B_SPLINE_CURVE ( 2, ( #17638, #19930, #14786, #29170, #28985, #6250, #8538, #17828, #31468 ),
 .UNSPECIFIED., .F., .F. ) 
 B_SPLINE_CURVE_WITH_KNOTS ( ( 3, 2, 2, 2, 3 ),
 ( 0.8152173913043478937, 0.8188405797101449002, 0.8260869565217391353, 0.8333333333333333703, 0.8369565217391303769 ),
 .UNSPECIFIED. ) 
 CURVE ( )  GEOMETRIC_REPRESENTATION_ITEM ( )  RATIONAL_B_SPLINE_CURVE ( ( 0.9330127018922192983, 0.9330127018922202975, 1.000000000000000000, 0.8660254037844387076, 1.000000000000000000, 0.8660254037844387076, 1.000000000000000000, 0.9330127018922202975, 0.9330127018922192983 ) ) 
 REPRESENTATION_ITEM ( '' )  );
#14644=VERTEX_POINT ( 'NONE', #7816 ) ;
#14649=CARTESIAN_POINT ( 'NONE',  ( 1.069080835302379631E-14, 195.2750000012290457, 27.00000000000000000 ) ) ;
#14651=CARTESIAN_POINT ( 'NONE',  ( 18.00000000000000355, 240.2312500012290570, 5.196152422706632912 ) ) ;
#14652=CARTESIAN_POINT ( 'NONE',  ( 15.24356964374999990, 246.2593750006145399, 0.000000000000000000 ) ) ;
#14654=DIRECTION ( 'NONE',  ( 0.000000000000000000, 0.000000000000000000, -1.000000000000000000 ) ) ;
#14658=CARTESIAN_POINT ( 'NONE',  ( 26.99999999999999645, 245.7437500012290457, 3.464101615137751278 ) ) ;
#14661=CARTESIAN_POINT ( 'NONE',  ( 27.00000000000001421, 198.0500000012290513, 15.58845726811988897 ) ) ;
#14667=ORIENTED_EDGE ( 'NONE', *, *, #27143, .T. ) ;
#14668=ORIENTED_EDGE ( 'NONE', *, *, #21240, .T. ) ;
#14671=CARTESIAN_POINT ( 'NONE',  ( 21.00000000000000000, 247.1593750006145171, 6.646953231504538984 ) ) ;
#14686=CARTESIAN_POINT ( 'NONE',  ( 22.60769515458672885, 240.6825961894323314, 5.999999999999997335 ) ) ;
#14700=CARTESIAN_POINT ( 'NONE',  ( -27.24356964374999990, 199.8218750006145399, -15.72908226750537786 ) ) ;
#14703=CARTESIAN_POINT ( 'NONE',  ( 23.87821517812499650, 246.1093750006145342, -4.985214923628404904 ) ) ;
#14711=CARTESIAN_POINT ( 'NONE',  ( 18.00000000000000000, 240.9250000000000114, -5.196152422706630247 ) ) ;
#14723=AXIS2_PLACEMENT_3D ( 'NONE', #32354, #3919, #6203 ) ;
#14725=CARTESIAN_POINT ( 'NONE',  ( 20.00041297495057080, 239.8598985277379256, -5.668978411116884608 ) ) ;
#14735=CARTESIAN_POINT ( 'NONE',  ( 27.24356964375000700, 196.8968750006145285, 15.72908226750537075 ) ) ;
#14737=EDGE_CURVE ( 'NONE', #15380, #22146, #5162, .T. ) ;
#14740=CARTESIAN_POINT ( 'NONE',  ( 15.00000000000000000, 244.6562500012290400, 0.000000000000000000 ) ) ;
#14746=CARTESIAN_POINT ( 'NONE',  ( 20.99999999999999645, 250.0000000000000000, 0.000000000000000000 ) ) ;
#14748=CARTESIAN_POINT ( 'NONE',  ( 15.00000000000000000, 249.5499999999999829, 0.000000000000000000 ) ) ;
#14749=CARTESIAN_POINT ( 'NONE',  ( 1.120210788295102201E-13, 196.7375000000000398, -27.00000000000000711 ) ) ;
#14750=AXIS2_PLACEMENT_3D ( 'NONE', #13036, #12656, #27429 ) ;
#14758=CARTESIAN_POINT ( 'NONE',  ( 27.00000000000000355, 196.1750000000000114, -3.306546357697854128E-15 ) ) ;
#14761=CARTESIAN_POINT ( 'NONE',  ( 21.00000000000000000, 248.7624999999999886, 6.928203230275506996 ) ) ;
#14762=CARTESIAN_POINT ( 'NONE',  ( -27.24356964375000345, 197.5156250006145342, -15.72908226750537786 ) ) ;
#14768=CARTESIAN_POINT ( 'NONE',  ( -1.926257025242585782E-15, 198.7906250006145399, -31.45816453501075927 ) ) ;
#14769=CARTESIAN_POINT ( 'NONE',  ( 15.24356964374999990, 242.5468750006145058, 0.000000000000000000 ) ) ;
#14770=EDGE_CURVE ( 'NONE', #22884, #16873, #20605, .T. ) ;
#14773=CARTESIAN_POINT ( 'NONE',  ( 26.75643035624999655, 248.2468750006145797, 3.323476615752267715 ) ) ;
#14775=EDGE_CURVE ( 'NONE', #17027, #10943, #3074, .T. ) ;
#14779=AXIS2_PLACEMENT_3D ( 'NONE', #13732, #33816, #19613 ) ;
#14780=CARTESIAN_POINT ( 'NONE',  ( 18.12178482187500350, 242.1718750006145058, 4.985214923628407568 ) ) ;
#14786=CARTESIAN_POINT ( 'NONE',  ( 18.00000000000000355, 241.1312500012290343, 5.196152422706632912 ) ) ;
#14794=CARTESIAN_POINT ( 'NONE',  ( 21.00000000000000000, 241.5343750006145171, -6.646953231504538984 ) ) ;
#14795=ORIENTED_EDGE ( 'NONE', *, *, #24850, .F. ) ;
#14800=CARTESIAN_POINT ( 'NONE',  ( 23.99999999999999645, 241.7500000000000000, -5.196152422706631135 ) ) ;
#14804=ADVANCED_FACE ( 'NONE', ( #36235 ), #16166, .F. ) ;
#14805=CARTESIAN_POINT ( 'NONE',  ( 4.178139385881633139, 195.0000000000000568, 26.92487590381980667 ) ) ;
#14808=VERTEX_POINT ( 'NONE', #14061 ) ;
#14809=CARTESIAN_POINT ( 'NONE',  ( 23.87821517812499650, 249.1468750006145285, -4.985214923628404904 ) ) ;
#14815=CYLINDRICAL_SURFACE ( 'NONE', #24990, 7.500000000000000000 ) ;
#14822=CARTESIAN_POINT ( 'NONE',  ( 19.39230484541326049, 245.4638461906613998, -5.999999999999997335 ) ) ;
#14829=( BOUNDED_CURVE ( )  B_SPLINE_CURVE ( 2, ( #32764, #12490, #10208, #12865, #9648, #35410, #9832, #32951, #7004 ),
 .UNSPECIFIED., .F., .F. ) 
 B_SPLINE_CURVE_WITH_KNOTS ( ( 3, 2, 2, 2, 3 ),
 ( 0.6195652173913043237, 0.6231884057971014412, 0.6304347826086956763, 0.6376811594202898004, 0.6413043478260869179 ),
 .UNSPECIFIED. ) 
 CURVE ( )  GEOMETRIC_REPRESENTATION_ITEM ( )  RATIONAL_B_SPLINE_CURVE ( ( 0.9330127018922194093, 0.9330127018922194093, 1.000000000000000000, 0.8660254037844387076, 1.000000000000000000, 0.8660254037844387076, 1.000000000000000000, 0.9330127018922194093, 0.9330127018922194093 ) ) 
 REPRESENTATION_ITEM ( '' )  );
#14830=CARTESIAN_POINT ( 'NONE',  ( -28.47956685997937498, 204.1588929126527603, 5.472637659619466355 ) ) ;
#14836=ORIENTED_EDGE ( 'NONE', *, *, #670, .T. ) ;
#14845=CARTESIAN_POINT ( 'NONE',  ( 23.87821517812499650, 244.7593750006145399, -4.985214923628404904 ) ) ;
#14847=CARTESIAN_POINT ( 'NONE',  ( 26.75643035624999655, 240.2218750006145456, -3.323476615752271268 ) ) ;
#14848=EDGE_LOOP ( 'NONE', ( #21456, #35254, #8981, #28311 ) ) ;
#14850=CARTESIAN_POINT ( 'NONE',  ( 15.00000000000000000, 247.3187500012290343, -3.464101615137752166 ) ) ;
#14858=ORIENTED_EDGE ( 'NONE', *, *, #20929, .F. ) ;
#14862=CARTESIAN_POINT ( 'NONE',  ( 26.75643035624999655, 245.5093750006145115, -3.323476615752271712 ) ) ;
#14875=ORIENTED_EDGE ( 'NONE', *, *, #1533, .F. ) ;
#14876=CARTESIAN_POINT ( 'NONE',  ( 26.99999999999999645, 240.8125000000000000, -3.464101615137755275 ) ) ;
#14889=CARTESIAN_POINT ( 'NONE',  ( -13.62178482187500528, 199.3343750006145569, -23.59362340125807123 ) ) ;
#14892=CARTESIAN_POINT ( 'NONE',  ( 15.24356964374999990, 247.1218750006145228, -3.323476615752268604 ) ) ;
#14895=DIRECTION ( 'NONE',  ( 1.000000000000000000, 0.000000000000000000, 0.000000000000000000 ) ) ;
#14899=CARTESIAN_POINT ( 'NONE',  ( 26.99999999999999645, 242.1624999999999659, -3.464101615137755275 ) ) ;
#14902=ORIENTED_EDGE ( 'NONE', *, *, #34903, .F. ) ;
#14910=CARTESIAN_POINT ( 'NONE',  ( 26.75643035624999655, 241.0468750006145058, 3.323476615752267715 ) ) ;
#14912=CARTESIAN_POINT ( 'NONE',  ( 20.99999999999999645, 185.0294372515228645, 5.999999999999999112 ) ) ;
#14920=CARTESIAN_POINT ( 'NONE',  ( -1.926257025242585782E-15, 196.5968750006145456, -31.45816453501075927 ) ) ;
#14939=ORIENTED_EDGE ( 'NONE', *, *, #17291, .T. ) ;
#14946=CARTESIAN_POINT ( 'NONE',  ( 15.00000000000000000, 248.2000000000000171, 0.000000000000000000 ) ) ;
#14947=CARTESIAN_POINT ( 'NONE',  ( 13.62178482187501416, 196.3531250006145115, 23.59362340125806767 ) ) ;
#14952=B_SPLINE_CURVE_WITH_KNOTS ( 'NONE', 1,
 ( #32132, #6171 ),
 .UNSPECIFIED., .F., .F.,
 ( 2, 2 ),
 ( 0.000000000000000000, 1.000000000000000000 ),
 .UNSPECIFIED. ) ;
#14953=CARTESIAN_POINT ( 'NONE',  ( -27.24356964375000345, 196.6531250006145513, 0.000000000000000000 ) ) ;
#14956=EDGE_CURVE ( 'NONE', #30367, #13498, #37343, .T. ) ;
#14959=CARTESIAN_POINT ( 'NONE',  ( 23.87821517812499650, 247.4593750006145285, -4.985214923628404904 ) ) ;
#14964=CARTESIAN_POINT ( 'NONE',  ( 18.12178482187500350, 241.2718750006145001, 4.985214923628407568 ) ) ;
#14970=CARTESIAN_POINT ( 'NONE',  ( 0.000000000000000000, 210.0000000000000284, 0.000000000000000000 ) ) ;
#14971=DIRECTION ( 'NONE',  ( 0.000000000000000000, -1.000000000000000000, 0.000000000000000000 ) ) ;
#14980=CARTESIAN_POINT ( 'NONE',  ( 18.12178482187500350, 241.2718750006145001, 4.985214923628407568 ) ) ;
#14981=ORIENTED_EDGE ( 'NONE', *, *, #20298, .T. ) ;
#14985=CYLINDRICAL_SURFACE ( 'NONE', #21550, 2.649999999999991029 ) ;
#14987=CARTESIAN_POINT ( 'NONE',  ( 14.99999999999999822, 204.0000000000000284, 3.514718625761426019 ) ) ;
#14990=CARTESIAN_POINT ( 'NONE',  ( 28.99999999999999645, 210.0000000000000284, 0.000000000000000000 ) ) ;
#14991=ORIENTED_EDGE ( 'NONE', *, *, #11549, .F. ) ;
#14992=CARTESIAN_POINT ( 'NONE',  ( 21.00000000000000000, 239.8187500012290343, 6.928203230275506996 ) ) ;
#14996=DIRECTION ( 'NONE',  ( 4.130293990420971855E-17, -1.000000000000000000, 0.000000000000000000 ) ) ;
#15002=EDGE_CURVE ( 'NONE', #2711, #32139, #31485, .T. ) ;
#15005=CARTESIAN_POINT ( 'NONE',  ( 15.24356964375000167, 248.8843750006145399, 3.323476615752272600 ) ) ;
#15006=CARTESIAN_POINT ( 'NONE',  ( -27.08961370327137175, 194.9999999999998863, -0.9223232689292477637 ) ) ;
#15011=CARTESIAN_POINT ( 'NONE',  ( 24.00000000000000000, 241.6562500012290400, 5.196152422706629359 ) ) ;
#15026=CARTESIAN_POINT ( 'NONE',  ( -1.045839947578415010E-13, 195.7250000012290343, 27.00000000000000355 ) ) ;
#15027=CARTESIAN_POINT ( 'NONE',  ( 20.99999999999999645, 185.0294372515228645, -5.999999999999999112 ) ) ;
#15028=CARTESIAN_POINT ( 'NONE',  ( 20.99999999999999289, 243.1937500012290343, -5.999999999999997335 ) ) ;
#15030=EDGE_CURVE ( 'NONE', #35488, #3383, #14143, .T. ) ;
#15031=CARTESIAN_POINT ( 'NONE',  ( 21.00000000000000000, 243.2218750006145456, 6.646953231504538984 ) ) ;
#15037=CARTESIAN_POINT ( 'NONE',  ( 21.00000000000000000, 246.3437500012290684, -6.928203230275506996 ) ) ;
#15048=CARTESIAN_POINT ( 'NONE',  ( 15.24356964375000167, 245.7343750006145058, 3.323476615752272600 ) ) ;
#15051=CARTESIAN_POINT ( 'NONE',  ( 16.22935424640156654, 222.7217220095854202, -3.659938751165931148 ) ) ;
#15065=ADVANCED_FACE ( 'NONE', ( #17093 ), #14613, .F. ) ;
#15071=DIRECTION ( 'NONE',  ( -0.000000000000000000, 1.000000000000000000, -0.000000000000000000 ) ) ;
#15073=CARTESIAN_POINT ( 'NONE',  ( 26.99999999999999645, 241.2437500012290457, 3.464101615137751278 ) ) ;
#15075=CARTESIAN_POINT ( 'NONE',  ( 15.00000000000000000, 240.0999999999999943, 0.000000000000000000 ) ) ;
#15077=CARTESIAN_POINT ( 'NONE',  ( 26.75643035624999655, 246.5218750006145285, -3.323476615752271268 ) ) ;
#15084=CARTESIAN_POINT ( 'NONE',  ( 23.99999999999999645, 240.8500000000000227, -5.196152422706631135 ) ) ;
#15088=EDGE_LOOP ( 'NONE', ( #21443, #20726, #24143 ) ) ;
#15090=CARTESIAN_POINT ( 'NONE',  ( 18.00000000000000000, 243.6250000000000000, -5.196152422706630247 ) ) ;
#15098=CARTESIAN_POINT ( 'NONE',  ( 18.12178482187499640, 239.8843750006145115, -4.985214923628404904 ) ) ;
#15100=CARTESIAN_POINT ( 'NONE',  ( -5.043980924894071016, 224.5060857195767596, 2.499999999999999112 ) ) ;
#15106=CARTESIAN_POINT ( 'NONE',  ( 15.00000000000000000, 240.9625000000000057, -3.464101615137752610 ) ) ;
#15107=CARTESIAN_POINT ( 'NONE',  ( -27.24356964374999635, 198.9406250006145171, 15.72908226750539384 ) ) ;
#15112=CARTESIAN_POINT ( 'NONE',  ( -5.732297079746171420, 222.9518338469886203, -2.500000000000000000 ) ) ;
#15120=CARTESIAN_POINT ( 'NONE',  ( 22.60769515458671108, 244.7325961894323143, 6.000000000000010658 ) ) ;
#15122=FACE_OUTER_BOUND ( 'NONE', #34200, .T. ) ;
#15127=VECTOR ( 'NONE', #36050, 1000.000000000000000 ) ;
#15131=CARTESIAN_POINT ( 'NONE',  ( 26.99999999999999645, 248.3875000000000171, 3.464101615137751278 ) ) ;
#15132=CARTESIAN_POINT ( 'NONE',  ( 13.62178482187499640, 196.9531250006145342, -23.59362340125807123 ) ) ;
#15136=CARTESIAN_POINT ( 'NONE',  ( -1.926257025242585782E-15, 195.1906250006145456, -31.45816453501075927 ) ) ;
#15137=CARTESIAN_POINT ( 'NONE',  ( 15.24356964374999990, 240.2968750006145342, 0.000000000000000000 ) ) ;
#15142=CARTESIAN_POINT ( 'NONE',  ( 18.12178482187500350, 247.2343750006145342, 4.985214923628407568 ) ) ;
#15149=CARTESIAN_POINT ( 'NONE',  ( 26.75643035624999655, 241.4218750006145058, -7.049594010296217766E-16 ) ) ;
#15154=EDGE_CURVE ( 'NONE', #18985, #3075, #13943, .T. ) ;
#15161=CARTESIAN_POINT ( 'NONE',  ( 22.60769515458672885, 248.5174038105676004, -6.000000000000000000 ) ) ;
#15162=DIRECTION ( 'NONE',  ( 1.000000000000000000, 0.000000000000000000, -0.000000000000000000 ) ) ;
#15163=CARTESIAN_POINT ( 'NONE',  ( 26.99999999999999645, 198.4625000000000057, -15.58845726811990495 ) ) ;
#15165=CARTESIAN_POINT ( 'NONE',  ( 21.00000000000000000, 249.4375000000000568, -5.999999999999998224 ) ) ;
#15169=CARTESIAN_POINT ( 'NONE',  ( 23.87821517812499650, 241.0468750006145058, -4.985214923628404904 ) ) ;
#15175=PLANE ( 'NONE',  #16701 ) ;
#15183=CARTESIAN_POINT ( 'NONE',  ( 15.24356964375000167, 247.5343750006144887, 3.323476615752272600 ) ) ;
#15197=CARTESIAN_POINT ( 'NONE',  ( 26.75643035624999655, 249.4843750006145058, 3.323476615752267271 ) ) ;
#15204=CARTESIAN_POINT ( 'NONE',  ( 19.39230484541326049, 248.5575961894323314, -5.999999999999994671 ) ) ;
#15212=ORIENTED_EDGE ( 'NONE', *, *, #9163, .T. ) ;
#15218=DIRECTION ( 'NONE',  ( -0.000000000000000000, 1.000000000000000000, -0.000000000000000000 ) ) ;
#15224=CARTESIAN_POINT ( 'NONE',  ( -4.500000000000000888, 210.0000000000000284, -2.500000000000000000 ) ) ;
#15226=CARTESIAN_POINT ( 'NONE',  ( 26.99999999999999645, 243.5687500012290343, -3.464101615137755275 ) ) ;
#15234=ORIENTED_EDGE ( 'NONE', *, *, #10189, .F. ) ;
#15237=CARTESIAN_POINT ( 'NONE',  ( 23.87821517812500005, 245.3968750006145285, 4.985214923628404016 ) ) ;
#15243=FACE_OUTER_BOUND ( 'NONE', #1374, .T. ) ;
#15257=CARTESIAN_POINT ( 'NONE',  ( 22.60769515458672885, 247.2236538117966802, -6.000000000000000000 ) ) ;
#15261=CARTESIAN_POINT ( 'NONE',  ( 13.50000000000001421, 195.6500000000000057, 23.38268590217984055 ) ) ;
#15263=CARTESIAN_POINT ( 'NONE',  ( 20.99999999999998579, 247.2437500012290457, -5.999999999999997335 ) ) ;
#15265=CARTESIAN_POINT ( 'NONE',  ( 26.75643035624999655, 247.4218750006145626, -3.323476615752271268 ) ) ;
#15268=AXIS2_PLACEMENT_3D ( 'NONE', #20446, #31988, #29134 ) ;
#15276=EDGE_LOOP ( 'NONE', ( #32703, #28233, #13322, #36265 ) ) ;
#15287=CARTESIAN_POINT ( 'NONE',  ( 19.39230484541326760, 243.8486538117966802, 5.999999999999999112 ) ) ;
#15290=CARTESIAN_POINT ( 'NONE',  ( 15.00000000000000178, 245.5375000000000227, 3.464101615137757051 ) ) ;
#15297=CARTESIAN_POINT ( 'NONE',  ( 13.62178482187501416, 199.5031250006145456, 23.59362340125806767 ) ) ;
#15302=CARTESIAN_POINT ( 'NONE',  ( 20.99999999999997868, 244.7687500012290513, 5.999999999999999112 ) ) ;
#15304=CARTESIAN_POINT ( 'NONE',  ( -27.00000000000000355, 197.7125000000000057, -15.58845726811989429 ) ) ;
#15313=CARTESIAN_POINT ( 'NONE',  ( 0.000000000000000000, 210.0000000000000284, 0.000000000000000000 ) ) ;
#15316=CARTESIAN_POINT ( 'NONE',  ( 26.99999999999999645, 244.8437500012290400, 3.464101615137751278 ) ) ;
#15319=CARTESIAN_POINT ( 'NONE',  ( -13.50000000000000533, 198.2375000012290229, -23.38268590217984411 ) ) ;
#15323=DIRECTION ( 'NONE',  ( 0.000000000000000000, -0.000000000000000000, 1.000000000000000000 ) ) ;
#15324=CARTESIAN_POINT ( 'NONE',  ( 21.00000000000000000, 248.9874999999999829, -6.928203230275506996 ) ) ;
#15325=CARTESIAN_POINT ( 'NONE',  ( 27.24356964375000700, 197.2906250006145399, 15.72908226750537075 ) ) ;
#15330=CARTESIAN_POINT ( 'NONE',  ( -1.909035429704832693E-15, 199.5500000012290513, -31.17691453623979214 ) ) ;
#15331=CARTESIAN_POINT ( 'NONE',  ( 15.24356964375000167, 239.8843750006145399, 3.323476615752272600 ) ) ;
#15334=CARTESIAN_POINT ( 'NONE',  ( 18.12178482187499640, 248.4343750006145228, -4.985214923628404904 ) ) ;
#15336=AXIS2_PLACEMENT_3D ( 'NONE', #36261, #36446, #4241 ) ;
#15358=CARTESIAN_POINT ( 'NONE',  ( 15.24356964374999990, 243.4093750006145171, -3.323476615752268604 ) ) ;
#15359=ORIENTED_EDGE ( 'NONE', *, *, #26547, .F. ) ;
#15364=( BOUNDED_CURVE ( )  B_SPLINE_CURVE ( 2, ( #32626, #18238, #15577, #1347, #36027, #15769, #9323, #4379, #24660 ),
 .UNSPECIFIED., .F., .F. ) 
 B_SPLINE_CURVE_WITH_KNOTS ( ( 3, 2, 2, 2, 3 ),
 ( 0.06250000000000000000, 0.06944444444444444753, 0.08333333333333332871, 0.09722222222222222376, 0.1041666666666666713 ),
 .UNSPECIFIED. ) 
 CURVE ( )  GEOMETRIC_REPRESENTATION_ITEM ( )  RATIONAL_B_SPLINE_CURVE ( ( 0.9330127018922194093, 0.9330127018922194093, 1.000000000000000000, 0.8660254037844387076, 1.000000000000000000, 0.8660254037844387076, 1.000000000000000000, 0.9330127018922192983, 0.9330127018922194093 ) ) 
 REPRESENTATION_ITEM ( '' )  );
#15371=ORIENTED_EDGE ( 'NONE', *, *, #23681, .T. ) ;
#15374=CARTESIAN_POINT ( 'NONE',  ( 21.00000000000000000, 246.2593750006145115, 6.646953231504538984 ) ) ;
#15380=VERTEX_POINT ( 'NONE', #2427 ) ;
#15385=ADVANCED_FACE ( 'NONE', ( #34083 ), #16665, .F. ) ;
#15388=CARTESIAN_POINT ( 'NONE',  ( 15.24356964374999990, 245.6593750006145740, -3.323476615752268604 ) ) ;
#15390=CARTESIAN_POINT ( 'NONE',  ( 13.49999999999999645, 196.7000000000000171, -23.38268590217984766 ) ) ;
#15392=DIRECTION ( 'NONE',  ( 0.000000000000000000, -0.000000000000000000, 1.000000000000000000 ) ) ;
#15395=CARTESIAN_POINT ( 'NONE',  ( 24.00000000000000000, 247.9562500012290229, 5.196152422706629359 ) ) ;
#15401=AXIS2_PLACEMENT_3D ( 'NONE', #18040, #25485, #14996 ) ;
#15402=CARTESIAN_POINT ( 'NONE',  ( 15.00000000000000000, 249.1187500012290741, -3.464101615137752610 ) ) ;
#15406=EDGE_LOOP ( 'NONE', ( #8472, #22000, #12085, #7611 ) ) ;
#15407=CARTESIAN_POINT ( 'NONE',  ( 10.49999999999999822, 210.0000000000000284, 2.500000000000000000 ) ) ;
#15419=CARTESIAN_POINT ( 'NONE',  ( 18.00000000000000000, 245.0312500012290400, -5.196152422706630247 ) ) ;
#15425=ORIENTED_EDGE ( 'NONE', *, *, #22157, .T. ) ;
#15428=CARTESIAN_POINT ( 'NONE',  ( 18.12178482187500350, 243.5218750006145001, 4.985214923628407568 ) ) ;
#15446=CARTESIAN_POINT ( 'NONE',  ( 20.99999999999999645, 185.0294372515228645, 5.999999999999999112 ) ) ;
#15455=CARTESIAN_POINT ( 'NONE',  ( 26.75643035624999655, 249.5968750006145171, 3.323476615752267715 ) ) ;
#15457=CARTESIAN_POINT ( 'NONE',  ( 18.12178482187500350, 245.8843750006145115, 4.985214923628407568 ) ) ;
#15468=ORIENTED_EDGE ( 'NONE', *, *, #18627, .T. ) ;
#15472=CARTESIAN_POINT ( 'NONE',  ( 22.60769515458670753, 243.1174038105676516, -6.000000000000011546 ) ) ;
#15477=CARTESIAN_POINT ( 'NONE',  ( 19.44430458907412174, 214.1485210958030052, 5.808099892140972109 ) ) ;
#15479=CARTESIAN_POINT ( 'NONE',  ( 0.000000000000000000, 210.0000000000000284, 0.000000000000000000 ) ) ;
#15486=CARTESIAN_POINT ( 'NONE',  ( 23.99999999999999645, 247.1500000000000057, -5.196152422706631135 ) ) ;
#15487=CARTESIAN_POINT ( 'NONE',  ( -27.24356964374999990, 198.4156250006145399, -15.72908226750537786 ) ) ;
#15502=EDGE_CURVE ( 'NONE', #2909, #25376, #26979, .T. ) ;
#15506=PLANE ( 'NONE',  #25053 ) ;
#15509=CARTESIAN_POINT ( 'NONE',  ( 23.99999999999999645, 244.9562500012290513, -5.196152422706631135 ) ) ;
#15511=CARTESIAN_POINT ( 'NONE',  ( -27.00000000000000355, 198.2750000012290172, -15.58845726811989429 ) ) ;
#15514=CARTESIAN_POINT ( 'NONE',  ( 21.00000000000000000, 245.8374999999999773, -6.928203230275506996 ) ) ;
#15515=CARTESIAN_POINT ( 'NONE',  ( 27.24356964375000345, 197.3281250006145342, -3.336375036156643733E-15 ) ) ;
#15522=CARTESIAN_POINT ( 'NONE',  ( 27.24356964375000345, 196.4281250006145569, -3.336375036156643733E-15 ) ) ;
#15526=CARTESIAN_POINT ( 'NONE',  ( 15.24356964375000167, 245.8468750006145171, 3.323476615752272600 ) ) ;
#15541=CARTESIAN_POINT ( 'NONE',  ( 20.99999999999999645, 242.0687500012290059, 5.999999999999998224 ) ) ;
#15542=CARTESIAN_POINT ( 'NONE',  ( 15.00000000000000178, 244.1875000000000000, 3.464101615137757051 ) ) ;
#15547=CARTESIAN_POINT ( 'NONE',  ( 23.87821517812500005, 249.1093750006145342, 4.985214923628404016 ) ) ;
#15554=FACE_OUTER_BOUND ( 'NONE', #17468, .T. ) ;
#15561=CARTESIAN_POINT ( 'NONE',  ( 23.87821517812499650, 247.7968750006145058, -4.985214923628404904 ) ) ;
#15574=CARTESIAN_POINT ( 'NONE',  ( 15.24356964375000167, 246.6343750006145115, 3.323476615752272600 ) ) ;
#15577=CARTESIAN_POINT ( 'NONE',  ( -13.49999999999998401, 199.2875000012290627, 23.38268590217985476 ) ) ;
#15582=CARTESIAN_POINT ( 'NONE',  ( 20.99999999999998579, 248.5374999999999659, -5.999999999999997335 ) ) ;
#15586=( BOUNDED_CURVE ( )  B_SPLINE_CURVE ( 2, ( #21643, #18051, #15390, #33196, #26747, #7237, #779, #26937, #7424 ),
 .UNSPECIFIED., .F., .F. ) 
 B_SPLINE_CURVE_WITH_KNOTS ( ( 3, 2, 2, 2, 3 ),
 ( 0.6041666666666667407, 0.6111111111111111605, 0.6250000000000000000, 0.6388888888888888395, 0.6458333333333333703 ),
 .UNSPECIFIED. ) 
 CURVE ( )  GEOMETRIC_REPRESENTATION_ITEM ( )  RATIONAL_B_SPLINE_CURVE ( ( 0.9330127018922192983, 0.9330127018922198534, 1.000000000000000000, 0.8660254037844387076, 1.000000000000000000, 0.8660254037844387076, 1.000000000000000000, 0.9330127018922187432, 0.9330127018922192983 ) ) 
 REPRESENTATION_ITEM ( '' )  );
#15587=CARTESIAN_POINT ( 'NONE',  ( 20.99999999999995381, 241.5625000000000000, 5.999999999999998224 ) ) ;
#15593=FACE_OUTER_BOUND ( 'NONE', #3190, .T. ) ;
#15597=CARTESIAN_POINT ( 'NONE',  ( -20.68320088531713452, 194.9994763905949924, -17.35526436380663284 ) ) ;
#15603=CARTESIAN_POINT ( 'NONE',  ( 21.00000000000000000, 244.9937500012290741, -6.928203230275506996 ) ) ;
#15606=CARTESIAN_POINT ( 'NONE',  ( 20.99999999999999289, 242.6875000000000000, -5.999999999999997335 ) ) ;
#15612=CARTESIAN_POINT ( 'NONE',  ( 21.00000000000000000, 244.2343750006145626, -6.646953231504538984 ) ) ;
#15617=( NAMED_UNIT ( * ) PLANE_ANGLE_UNIT ( ) SI_UNIT ( $, .RADIAN. ) );
#15633=ORIENTED_EDGE ( 'NONE', *, *, #16918, .F. ) ;
#15643=CARTESIAN_POINT ( 'NONE',  ( 15.24356964375000167, 249.4468750006145399, 3.323476615752272600 ) ) ;
#15645=CARTESIAN_POINT ( 'NONE',  ( 15.24356964374999990, 244.8718750006145797, -3.323476615752268604 ) ) ;
#15646=ORIENTED_EDGE ( 'NONE', *, *, #16439, .T. ) ;
#15657=EDGE_LOOP ( 'NONE', ( #17287, #5740, #33747, #4630, #31255, #3547, #28055 ) ) ;
#15660=DIRECTION ( 'NONE',  ( 0.000000000000000000, 0.000000000000000000, 1.000000000000000000 ) ) ;
#15667=CARTESIAN_POINT ( 'NONE',  ( 14.06021656787942753, 216.9397834321235621, 0.8200469388724418440 ) ) ;
#15677=CARTESIAN_POINT ( 'NONE',  ( 5.778771075727756162E-15, 197.6656250006145399, 31.45816453501075927 ) ) ;
#15680=EDGE_CURVE ( 'NONE', #13498, #17027, #17028, .T. ) ;
#15695=CARTESIAN_POINT ( 'NONE',  ( 27.00000000000000355, 199.7750000000000057, -3.306546357697854128E-15 ) ) ;
#15696=LINE ( 'NONE', #3741, #28661 ) ;
#15702=CARTESIAN_POINT ( 'NONE',  ( -1.045839947578415010E-13, 195.7250000012290343, 27.00000000000000355 ) ) ;
#15705=CARTESIAN_POINT ( 'NONE',  ( 15.00000000000000000, 245.9125000000000227, -3.464101615137752166 ) ) ;
#15706=CARTESIAN_POINT ( 'NONE',  ( -13.62178482187500528, 195.2281250006145399, -23.59362340125807123 ) ) ;
#15710=ORIENTED_EDGE ( 'NONE', *, *, #29602, .F. ) ;
#15711=CARTESIAN_POINT ( 'NONE',  ( -26.99999999999998934, 197.9000000012290172, 15.58845726811991561 ) ) ;
#15715=CARTESIAN_POINT ( 'NONE',  ( 26.75643035624999655, 244.2718750006145001, -3.323476615752271712 ) ) ;
#15722=CARTESIAN_POINT ( 'NONE',  ( 26.99999999999999645, 198.0125000000000739, -15.58845726811990495 ) ) ;
#15736=CARTESIAN_POINT ( 'NONE',  ( 21.00000000000000000, 248.8468750006145456, -6.646953231504538984 ) ) ;
#15740=CARTESIAN_POINT ( 'NONE',  ( 13.62178482187499640, 199.2593750006145399, -23.59362340125807123 ) ) ;
#15744=CARTESIAN_POINT ( 'NONE',  ( 21.00000000000000000, 242.9968750006145228, -6.646953231504538984 ) ) ;
#15750=ORIENTED_EDGE ( 'NONE', *, *, #29030, .T. ) ;
#15751=CARTESIAN_POINT ( 'NONE',  ( 21.00000000000000000, 245.8093750006144944, 6.646953231504538984 ) ) ;
#15755=EDGE_CURVE ( 'NONE', #23005, #36021, #31299, .T. ) ;
#15767=CARTESIAN_POINT ( 'NONE',  ( 26.75643035624999655, 246.8593750006145342, -3.323476615752271268 ) ) ;
#15769=CARTESIAN_POINT ( 'NONE',  ( -27.00000000000000355, 199.1750000012290513, -15.58845726811989429 ) ) ;
#15773=ORIENTED_EDGE ( 'NONE', *, *, #32719, .F. ) ;
#15775=AXIS2_PLACEMENT_3D ( 'NONE', #36230, #10089, #21846 ) ;
#15779=CARTESIAN_POINT ( 'NONE',  ( 18.00000000000000000, 241.3750000000000000, -5.196152422706630247 ) ) ;
#15783=ORIENTED_EDGE ( 'NONE', *, *, #24836, .T. ) ;
#15790=CARTESIAN_POINT ( 'NONE',  ( 13.49999999999999645, 195.8000000000000114, -23.38268590217984766 ) ) ;
#15795=CARTESIAN_POINT ( 'NONE',  ( 26.99999999999999645, 244.8812500012290343, -7.347880794884117764E-16 ) ) ;
#15802=DIRECTION ( 'NONE',  ( -0.000000000000000000, 1.000000000000000000, -0.000000000000000000 ) ) ;
#15803=CARTESIAN_POINT ( 'NONE',  ( 21.00000000000000000, 243.7843750006144887, -6.646953231504538984 ) ) ;
#15807=SHAPE_REPRESENTATION_RELATIONSHIP ( 'NONE' , 'NONE' ,  #9842, #21035 ) ;
#15808=CARTESIAN_POINT ( 'NONE',  ( 20.99999999999999645, 185.0294372515228645, 0.000000000000000000 ) ) ;
#15819=CARTESIAN_POINT ( 'NONE',  ( 20.99999999999999645, 185.0294372515228645, -5.999999999999999112 ) ) ;
#15824=CARTESIAN_POINT ( 'NONE',  ( 0.3500000000000069722, 244.5000000000000000, -2.499999999999999556 ) ) ;
#15828=CARTESIAN_POINT ( 'NONE',  ( 1.120210788295102201E-13, 195.3875000000000455, -27.00000000000000711 ) ) ;
#15831=CARTESIAN_POINT ( 'NONE',  ( 18.12178482187500350, 249.0343750006145456, 4.985214923628407568 ) ) ;
#15833=CARTESIAN_POINT ( 'NONE',  ( 15.24356964374999990, 244.4218750006145058, -3.323476615752268604 ) ) ;
#15841=ORIENTED_EDGE ( 'NONE', *, *, #21063, .F. ) ;
#15845=DIRECTION ( 'NONE',  ( -0.000000000000000000, 1.000000000000000000, -0.000000000000000000 ) ) ;
#15847=CARTESIAN_POINT ( 'NONE',  ( 20.99999999999999645, 249.2687500012290513, 5.999999999999998224 ) ) ;
#15850=VECTOR ( 'NONE', #3701, 1000.000000000000000 ) ;
#15855=CARTESIAN_POINT ( 'NONE',  ( 15.90209636607598931, 223.5944096904600542, 3.170162721592977739 ) ) ;
#15858=CARTESIAN_POINT ( 'NONE',  ( 15.00000000000000000, 245.5000000000000000, 0.000000000000000000 ) ) ;
#15867=CARTESIAN_POINT ( 'NONE',  ( 27.24356964374999635, 199.6156250006145285, -15.72908226750539029 ) ) ;
#15875=( BOUNDED_CURVE ( )  B_SPLINE_CURVE ( 2, ( #10644, #33774, #2112, #9900, #21484, #20309, #28267, #34140, #22594 ),
 .UNSPECIFIED., .F., .F. ) 
 B_SPLINE_CURVE_WITH_KNOTS ( ( 3, 2, 2, 2, 3 ),
 ( 0.2500000000000000000, 0.2536231884057971175, 0.2608695652173912971, 0.2681159420289855322, 0.2717391304347825942 ),
 .UNSPECIFIED. ) 
 CURVE ( )  GEOMETRIC_REPRESENTATION_ITEM ( )  RATIONAL_B_SPLINE_CURVE ( ( 0.9330127018922194093, 0.9330127018922190762, 1.000000000000000000, 0.8660254037844387076, 1.000000000000000000, 0.8660254037844387076, 1.000000000000000000, 0.9330127018922198534, 0.9330127018922191873 ) ) 
 REPRESENTATION_ITEM ( '' )  );
#15882=DIRECTION ( 'NONE',  ( -1.000000000000000000, 0.000000000000000000, 0.000000000000000000 ) ) ;
#15884=CARTESIAN_POINT ( 'NONE',  ( 13.49999999999999645, 199.4000000000000341, -23.38268590217984766 ) ) ;
#15888=CARTESIAN_POINT ( 'NONE',  ( 20.99999999999999289, 241.7874999999999659, -5.999999999999997335 ) ) ;
#15894=CARTESIAN_POINT ( 'NONE',  ( 15.00000000000000178, 246.8874999999999886, 3.464101615137757051 ) ) ;
#15900=CARTESIAN_POINT ( 'NONE',  ( 27.00000000000001066, 198.9500000012290570, 15.58845726811988897 ) ) ;
#15902=EDGE_CURVE ( 'NONE', #20414, #32797, #14558, .T. ) ;
#15905=CARTESIAN_POINT ( 'NONE',  ( 15.24356964374999990, 246.2593750006145399, 0.000000000000000000 ) ) ;
#15912=CARTESIAN_POINT ( 'NONE',  ( 18.12178482187499640, 239.7718750006145001, -4.985214923628404904 ) ) ;
#15924=DIRECTION ( 'NONE',  ( -0.000000000000000000, -1.000000000000000000, -0.000000000000000000 ) ) ;
#15927=CARTESIAN_POINT ( 'NONE',  ( 18.12178482187500350, 249.4843750006145342, 4.985214923628407568 ) ) ;
#15932=CARTESIAN_POINT ( 'NONE',  ( 27.24356964375000700, 196.8968750006144717, 15.72908226750537075 ) ) ;
#15935=CARTESIAN_POINT ( 'NONE',  ( 26.75643035624999655, 243.3718750006145228, -3.323476615752271712 ) ) ;
#15936=VECTOR ( 'NONE', #36942, 1000.000000000000000 ) ;
#15942=CARTESIAN_POINT ( 'NONE',  ( 15.24356964374999990, 247.4968750006145228, 0.000000000000000000 ) ) ;
#15955=CARTESIAN_POINT ( 'NONE',  ( 23.87821517812500005, 247.1968750006145115, 4.985214923628404016 ) ) ;
#15958=CARTESIAN_POINT ( 'NONE',  ( 20.99999999999997868, 246.0625000000000284, 5.999999999999999112 ) ) ;
#15960=ORIENTED_EDGE ( 'NONE', *, *, #22903, .T. ) ;
#15978=CARTESIAN_POINT ( 'NONE',  ( 19.39230484541326049, 244.9575961894323086, -5.999999999999997335 ) ) ;
#15979=CARTESIAN_POINT ( 'NONE',  ( 5.778771075727756162E-15, 197.2718750006145569, 31.45816453501075927 ) ) ;
#15981=VECTOR ( 'NONE', #28535, 1000.000000000000000 ) ;
#15983=CARTESIAN_POINT ( 'NONE',  ( 26.99999999999999645, 242.1625000000000227, -3.464101615137755275 ) ) ;
#15985=EDGE_LOOP ( 'NONE', ( #28319, #7402, #28925, #7046 ) ) ;
#15986=CARTESIAN_POINT ( 'NONE',  ( 24.00000000000000000, 243.4562500012290513, 5.196152422706629359 ) ) ;
#15992=VERTEX_POINT ( 'NONE', #18664 ) ;
#15993=B_SPLINE_CURVE_WITH_KNOTS ( 'NONE', 1,
 ( #33481, #14138 ),
 .UNSPECIFIED., .F., .F.,
 ( 2, 2 ),
 ( 0.000000000000000000, 1.000000000000000000 ),
 .UNSPECIFIED. ) ;
#15995=CARTESIAN_POINT ( 'NONE',  ( 26.75643035624999655, 244.6093750006145342, -3.323476615752271712 ) ) ;
#16006=DIRECTION ( 'NONE',  ( -0.000000000000000000, -1.000000000000000000, -0.000000000000000000 ) ) ;
#16013=CARTESIAN_POINT ( 'NONE',  ( -28.78598427599741072, 202.8118011321232643, -3.549815969672131200 ) ) ;
#16023=CARTESIAN_POINT ( 'NONE',  ( 23.87821517812500005, 245.0593750006145228, 4.985214923628404016 ) ) ;
#16036=CARTESIAN_POINT ( 'NONE',  ( -1.045839947578415010E-13, 196.0625000000000284, 27.00000000000000355 ) ) ;
#16045=CARTESIAN_POINT ( 'NONE',  ( 8.945811011644241972, 214.5203208706332418, 3.964960503605297948 ) ) ;
#16047=CARTESIAN_POINT ( 'NONE',  ( 0.000000000000000000, 0.000000000000000000, 0.000000000000000000 ) ) ;
#16054=CARTESIAN_POINT ( 'NONE',  ( 27.24356964374999635, 196.9156250006145399, -15.72908226750539029 ) ) ;
#16072=CARTESIAN_POINT ( 'NONE',  ( 26.99999999999999645, 199.8125000000000000, -15.58845726811990495 ) ) ;
#16073=CARTESIAN_POINT ( 'NONE',  ( -27.24356964375000345, 199.8312500006145171, 0.000000000000000000 ) ) ;
#16081=CARTESIAN_POINT ( 'NONE',  ( 26.99999999999999645, 244.7874999999999943, 3.464101615137751278 ) ) ;
#16086=ORIENTED_EDGE ( 'NONE', *, *, #29560, .F. ) ;
#16087=CARTESIAN_POINT ( 'NONE',  ( 26.99999999999999645, 199.4750000012290343, -15.58845726811990495 ) ) ;
#16091=CARTESIAN_POINT ( 'NONE',  ( 15.24356964375000167, 246.2968750006145626, 3.323476615752272600 ) ) ;
#16096=ADVANCED_FACE ( 'NONE', ( #15243 ), #30205, .F. ) ;
#16098=CARTESIAN_POINT ( 'NONE',  ( 13.50000000000001421, 197.9000000000000341, 23.38268590217984055 ) ) ;
#16112=CARTESIAN_POINT ( 'NONE',  ( 20.99999999999999289, 240.4937500012290457, -5.999999999999997335 ) ) ;
#16113=CARTESIAN_POINT ( 'NONE',  ( 23.87821517812500005, 249.5593750006145228, 4.985214923628404016 ) ) ;
#16118=CARTESIAN_POINT ( 'NONE',  ( -27.24356964374999279, 196.7468750006145513, 15.72908226750539384 ) ) ;
#16121=CARTESIAN_POINT ( 'NONE',  ( 26.75643035624999655, 242.4343750006145513, -7.049594010296217766E-16 ) ) ;
#16127=CARTESIAN_POINT ( 'NONE',  ( 23.87821517812500005, 245.3968750006145285, 4.985214923628404016 ) ) ;
#16141=CARTESIAN_POINT ( 'NONE',  ( 26.75643035624999655, 245.9218750006145342, -7.049594010296217766E-16 ) ) ;
#16150=CARTESIAN_POINT ( 'NONE',  ( 15.00000000000000178, 244.6375000000000171, 3.464101615137757051 ) ) ;
#16157=EDGE_LOOP ( 'NONE', ( #12431, #31701, #5519, #31306 ) ) ;
#16163=LINE ( 'NONE', #4950, #9914 ) ;
#16164=CARTESIAN_POINT ( 'NONE',  ( 13.62178482187499640, 197.0093750006145399, -23.59362340125807123 ) ) ;
#16166=CYLINDRICAL_SURFACE ( 'NONE', #25432, 6.000000000000005329 ) ;
#16170=CARTESIAN_POINT ( 'NONE',  ( 24.00000000000000000, 241.6562500012290400, 5.196152422706629359 ) ) ;
#16173=CARTESIAN_POINT ( 'NONE',  ( 27.24356964375000345, 199.5781250006145342, -3.336375036156643733E-15 ) ) ;
#16179=AXIS2_PLACEMENT_3D ( 'NONE', #23781, #35514, #6909 ) ;
#16183=CARTESIAN_POINT ( 'NONE',  ( -7.234628195640354420, 196.4924038105676800, 26.99999999999996803 ) ) ;
#16203=CARTESIAN_POINT ( 'NONE',  ( -27.00000000000000355, 199.0999999999999943, 0.000000000000000000 ) ) ;
#16204=CARTESIAN_POINT ( 'NONE',  ( 5.000000000000127010, 225.9999999999999432, 7.999999999999943157 ) ) ;
#16207=CARTESIAN_POINT ( 'NONE',  ( 23.87821517812500005, 248.6593750006145171, 4.985214923628404016 ) ) ;
#16209=CARTESIAN_POINT ( 'NONE',  ( 26.75643035624999655, 243.3718750006145228, -3.323476615752271268 ) ) ;
#16211=CARTESIAN_POINT ( 'NONE',  ( 20.99999999999999645, 241.1125000000000114, 5.999999999999998224 ) ) ;
#16230=CARTESIAN_POINT ( 'NONE',  ( 15.07698242245262144, 225.7947135401293792, 0.9779651927385701882 ) ) ;
#16238=EDGE_CURVE ( 'NONE', #30702, #29886, #23329, .T. ) ;
#16240=CARTESIAN_POINT ( 'NONE',  ( -27.24356964374999635, 196.6906250006145456, 15.72908226750539384 ) ) ;
#16244=VERTEX_POINT ( 'NONE', #1944 ) ;
#16245=DIRECTION ( 'NONE',  ( -0.000000000000000000, 1.000000000000000000, -0.000000000000000000 ) ) ;
#16258=AXIS2_PLACEMENT_3D ( 'NONE', #14014, #31996, #25564 ) ;
#16262=CARTESIAN_POINT ( 'NONE',  ( 0.3500000000000069722, 244.5000000000000000, 5.000000000000000000 ) ) ;
#16267=( BOUNDED_CURVE ( )  B_SPLINE_CURVE ( 2, ( #22776, #14422, #11203, #11764, #23147, #8736, #28813, #20116, #34881 ),
 .UNSPECIFIED., .F., .F. ) 
 B_SPLINE_CURVE_WITH_KNOTS ( ( 3, 2, 2, 2, 3 ),
 ( 0.8369565217391303769, 0.8405797101449274944, 0.8478260869565217295, 0.8550724637681159646, 0.8586956521739130821 ),
 .UNSPECIFIED. ) 
 CURVE ( )  GEOMETRIC_REPRESENTATION_ITEM ( )  RATIONAL_B_SPLINE_CURVE ( ( 0.9330127018922192983, 0.9330127018922182991, 1.000000000000000000, 0.8660254037844387076, 1.000000000000000000, 0.8660254037844387076, 1.000000000000000000, 0.9330127018922194093, 0.9330127018922194093 ) ) 
 REPRESENTATION_ITEM ( '' )  );
#16268=CARTESIAN_POINT ( 'NONE',  ( 15.00000000000000000, 246.8125000000000000, -3.464101615137752166 ) ) ;
#16275=CARTESIAN_POINT ( 'NONE',  ( -1.909035429704832693E-15, 197.3000000012290513, -31.17691453623979214 ) ) ;
#16279=CARTESIAN_POINT ( 'NONE',  ( 18.12178482187500350, 244.0843750006145285, 4.985214923628407568 ) ) ;
#16285=CARTESIAN_POINT ( 'NONE',  ( -13.62178482187500528, 197.9843750006145626, -23.59362340125807123 ) ) ;
#16298=CARTESIAN_POINT ( 'NONE',  ( 18.12178482187500350, 249.0343750006145456, 4.985214923628407568 ) ) ;
#16302=CARTESIAN_POINT ( 'NONE',  ( -1.926257025242585782E-15, 198.8468750006145740, -31.45816453501076637 ) ) ;
#16306=CARTESIAN_POINT ( 'NONE',  ( 18.12178482187500350, 244.0843750006145285, 4.985214923628407568 ) ) ;
#16311=EDGE_LOOP ( 'NONE', ( #20225, #27821, #8843, #7923 ) ) ;
#16312=ORIENTED_EDGE ( 'NONE', *, *, #10287, .T. ) ;
#16313=CARTESIAN_POINT ( 'NONE',  ( 23.87821517812500005, 244.0468750006145058, 4.985214923628404016 ) ) ;
#16326=CARTESIAN_POINT ( 'NONE',  ( 18.12178482187500350, 243.9718750006145171, 4.985214923628407568 ) ) ;
#16327=DIRECTION ( 'NONE',  ( 4.130293990420971855E-17, -1.000000000000000000, 0.000000000000000000 ) ) ;
#16331=EDGE_CURVE ( 'NONE', #8598, #6593, #28884, .T. ) ;
#16334=CARTESIAN_POINT ( 'NONE',  ( 20.99999999999995381, 244.7125000000000057, 5.999999999999998224 ) ) ;
#16340=DIRECTION ( 'NONE',  ( 0.000000000000000000, 0.000000000000000000, 1.000000000000000000 ) ) ;
#16345=CARTESIAN_POINT ( 'NONE',  ( 20.99999999999999289, 244.9374999999999716, -5.999999999999997335 ) ) ;
#16346=CARTESIAN_POINT ( 'NONE',  ( 27.24356964374999635, 198.7718750006145569, -15.72908226750539029 ) ) ;
#16352=CARTESIAN_POINT ( 'NONE',  ( 26.99999999999999645, 241.2812500012290400, -7.347880794884117764E-16 ) ) ;
#16356=CARTESIAN_POINT ( 'NONE',  ( 27.24356964375000700, 198.6406250006145058, 15.72908226750537075 ) ) ;
#16383=( BOUNDED_CURVE ( )  B_SPLINE_CURVE ( 2, ( #36720, #34066, #33508, #1667, #36529, #30491, #1853, #18755, #30297 ),
 .UNSPECIFIED., .F., .F. ) 
 B_SPLINE_CURVE_WITH_KNOTS ( ( 3, 2, 2, 2, 3 ),
 ( 0.5625000000000000000, 0.5694444444444444198, 0.5833333333333333703, 0.5972222222222222099, 0.6041666666666667407 ),
 .UNSPECIFIED. ) 
 CURVE ( )  GEOMETRIC_REPRESENTATION_ITEM ( )  RATIONAL_B_SPLINE_CURVE ( ( 0.9330127018922194093, 0.9330127018922194093, 1.000000000000000000, 0.8660254037844387076, 1.000000000000000000, 0.8660254037844387076, 1.000000000000000000, 0.9330127018922187432, 0.9330127018922192983 ) ) 
 REPRESENTATION_ITEM ( '' )  );
#16384=CARTESIAN_POINT ( 'NONE',  ( -29.00000000000001066, 202.0000000000000000, -0.5248785063507624971 ) ) ;
#16390=CARTESIAN_POINT ( 'NONE',  ( 26.99999999999999645, 195.4250000012290229, -15.58845726811990495 ) ) ;
#16393=CARTESIAN_POINT ( 'NONE',  ( 15.24356964375000167, 247.6468750006145569, 3.323476615752272600 ) ) ;
#16395=CARTESIAN_POINT ( 'NONE',  ( 18.12178482187499640, 243.0343750006145456, -4.985214923628404904 ) ) ;
#16396=ORIENTED_EDGE ( 'NONE', *, *, #19461, .T. ) ;
#16397=CARTESIAN_POINT ( 'NONE',  ( 26.99999999999999645, 248.4812500012290570, -7.347880794884117764E-16 ) ) ;
#16411=CARTESIAN_POINT ( 'NONE',  ( 21.00000000000000000, 248.9593750006145285, 6.646953231504538984 ) ) ;
#16415=CARTESIAN_POINT ( 'NONE',  ( 15.07698242245260722, 225.7947135401219612, -0.9779651927385025756 ) ) ;
#16425=CARTESIAN_POINT ( 'NONE',  ( 27.24356964374999635, 196.0156250006145626, -15.72908226750539029 ) ) ;
#16429=DIRECTION ( 'NONE',  ( -1.000000000000000000, 0.000000000000000000, 0.000000000000000000 ) ) ;
#16439=EDGE_CURVE ( 'NONE', #25531, #14300, #15364, .T. ) ;
#16440=DIRECTION ( 'NONE',  ( -0.000000000000000000, -1.000000000000000000, -0.000000000000000000 ) ) ;
#16444=CARTESIAN_POINT ( 'NONE',  ( -1.909035429704832693E-15, 198.9875000000000114, -31.17691453623979214 ) ) ;
#16454=CARTESIAN_POINT ( 'NONE',  ( 15.00000000000000000, 242.7999999999999829, 0.000000000000000000 ) ) ;
#16455=CARTESIAN_POINT ( 'NONE',  ( 12.48663586349064403, 194.9999999999999716, 24.21355016816918493 ) ) ;
#16461=CARTESIAN_POINT ( 'NONE',  ( 27.00000000000000355, 198.9875000012290229, -3.306546357697854128E-15 ) ) ;
#16462=CARTESIAN_POINT ( 'NONE',  ( 18.00000000000000000, 248.6312500012290343, -5.196152422706630247 ) ) ;
#16465=CARTESIAN_POINT ( 'NONE',  ( 18.12178482187499640, 242.5843750006145285, -4.985214923628404904 ) ) ;
#16471=CARTESIAN_POINT ( 'NONE',  ( -27.24356964375000345, 199.4093750006145456, 0.000000000000000000 ) ) ;
#16476=DIRECTION ( 'NONE',  ( 1.000000000000000000, 4.130293990420971855E-17, -0.000000000000000000 ) ) ;
#16481=CARTESIAN_POINT ( 'NONE',  ( -7.234628195640313564, 199.5700961906613884, -27.00000000000000355 ) ) ;
#16485=LINE ( 'NONE', #9852, #29977 ) ;
#16486=CARTESIAN_POINT ( 'NONE',  ( 26.99999999999999645, 240.4187500012290570, -3.464101615137755275 ) ) ;
#16490=CARTESIAN_POINT ( 'NONE',  ( 27.24356964374999279, 198.7718750006145569, -15.72908226750539207 ) ) ;
#16494=CARTESIAN_POINT ( 'NONE',  ( 26.75643035624999655, 240.6718750006145910, -3.323476615752271712 ) ) ;
#16499=EDGE_LOOP ( 'NONE', ( #8798, #25012, #28439, #29053 ) ) ;
#16500=CARTESIAN_POINT ( 'NONE',  ( 26.75643035624999655, 244.5343750006144887, 3.323476615752267715 ) ) ;
#16508=ORIENTED_EDGE ( 'NONE', *, *, #16559, .T. ) ;
#16513=CARTESIAN_POINT ( 'NONE',  ( 15.24356964375000167, 244.8343750006145285, 3.323476615752272600 ) ) ;
#16522=CARTESIAN_POINT ( 'NONE',  ( 26.99999999999999645, 242.5937500012290400, 3.464101615137751278 ) ) ;
#16533=CARTESIAN_POINT ( 'NONE',  ( 5.778771075727756162E-15, 197.7218750006145456, 31.45816453501075927 ) ) ;
#16535=CARTESIAN_POINT ( 'NONE',  ( 22.60769515458672885, 244.0174038105676289, -5.999999999999998224 ) ) ;
#16541=CARTESIAN_POINT ( 'NONE',  ( 24.00000000000000000, 241.2062500012290513, 5.196152422706629359 ) ) ;
#16544=CARTESIAN_POINT ( 'NONE',  ( 27.24356964375000700, 197.2906250006145399, 15.72908226750537075 ) ) ;
#16555=CARTESIAN_POINT ( 'NONE',  ( -13.49999999999998401, 196.4750000000000227, 23.38268590217985476 ) ) ;
#16559=EDGE_CURVE ( 'NONE', #6008, #2166, #32812, .T. ) ;
#16569=LINE ( 'NONE', #1400, #22230 ) ;
#16570=ORIENTED_EDGE ( 'NONE', *, *, #24057, .F. ) ;
#16574=CARTESIAN_POINT ( 'NONE',  ( 22.60769515458674306, 247.4325961894323598, 5.999999999999992895 ) ) ;
#16575=CARTESIAN_POINT ( 'NONE',  ( 13.50000000000001421, 195.3125000012290400, 23.38268590217984055 ) ) ;
#16576=CARTESIAN_POINT ( 'NONE',  ( 20.99999999999999289, 242.6875000000000000, -5.999999999999997335 ) ) ;
#16579=CARTESIAN_POINT ( 'NONE',  ( 23.87821517812499650, 247.0093750006145399, -4.985214923628404904 ) ) ;
#16581=CARTESIAN_POINT ( 'NONE',  ( 18.12178482187500350, 241.3843750006145115, 4.985214923628407568 ) ) ;
#16585=CARTESIAN_POINT ( 'NONE',  ( 15.00000000000000178, 248.7437500012290457, 3.464101615137757051 ) ) ;
#16589=( BOUNDED_CURVE ( )  B_SPLINE_CURVE ( 2, ( #12169, #24497, #18252, #12364, #7070, #21290, #26951, #23934, #18638 ),
 .UNSPECIFIED., .F., .F. ) 
 B_SPLINE_CURVE_WITH_KNOTS ( ( 3, 2, 2, 2, 3 ),
 ( 0.3541666666666666852, 0.3611111111111111049, 0.3750000000000000000, 0.3888888888888888951, 0.3958333333333333703 ),
 .UNSPECIFIED. ) 
 CURVE ( )  GEOMETRIC_REPRESENTATION_ITEM ( )  RATIONAL_B_SPLINE_CURVE ( ( 0.9330127018922194093, 0.9330127018922196314, 1.000000000000000000, 0.8660254037844387076, 1.000000000000000000, 0.8660254037844387076, 1.000000000000000000, 0.9330127018922190762, 0.9330127018922194093 ) ) 
 REPRESENTATION_ITEM ( '' )  );
#16590=CARTESIAN_POINT ( 'NONE',  ( 22.60769515458670753, 240.9236538117966973, -6.000000000000011546 ) ) ;
#16593=EDGE_LOOP ( 'NONE', ( #29093, #19307, #10446, #7170 ) ) ;
#16603=CARTESIAN_POINT ( 'NONE',  ( 14.99999999999954170, 215.9999999999999716, -0.1308996912579681871 ) ) ;
#16605=CARTESIAN_POINT ( 'NONE',  ( 27.00000000000001421, 197.0374999999999943, 15.58845726811988897 ) ) ;
#16610=( BOUNDED_CURVE ( )  B_SPLINE_CURVE ( 2, ( #36457, #22076, #30787, #16390, #13536, #25091, #16575, #17501, #14649 ),
 .UNSPECIFIED., .F., .F. ) 
 B_SPLINE_CURVE_WITH_KNOTS ( ( 3, 2, 2, 2, 3 ),
 ( 0.7708333333333333703, 0.7777777777777777901, 0.7916666666666666297, 0.8055555555555555802, 0.8125000000000000000 ),
 .UNSPECIFIED. ) 
 CURVE ( )  GEOMETRIC_REPRESENTATION_ITEM ( )  RATIONAL_B_SPLINE_CURVE ( ( 0.9330127018922192983, 0.9330127018922198534, 1.000000000000000000, 0.8660254037844387076, 1.000000000000000000, 0.8660254037844387076, 1.000000000000000000, 0.9330127018922194093, 0.9330127018922194093 ) ) 
 REPRESENTATION_ITEM ( '' )  );
#16612=CARTESIAN_POINT ( 'NONE',  ( 27.24356964375000700, 195.9406250006145456, 15.72908226750537075 ) ) ;
#16615=ORIENTED_EDGE ( 'NONE', *, *, #25166, .T. ) ;
#16616=CARTESIAN_POINT ( 'NONE',  ( 24.00000000000000000, 242.1062500012290286, 5.196152422706629359 ) ) ;
#16632=CARTESIAN_POINT ( 'NONE',  ( -1.909035429704832693E-15, 198.5374999999999943, -31.17691453623979214 ) ) ;
#16636=CARTESIAN_POINT ( 'NONE',  ( 15.24356964374999990, 249.3718750006145228, -3.323476615752268604 ) ) ;
#16643=CARTESIAN_POINT ( 'NONE',  ( 15.00000000000000178, 242.3875000000000171, 3.464101615137757051 ) ) ;
#16644=CARTESIAN_POINT ( 'NONE',  ( 13.06157021329630474, 195.0015827616130650, 23.91706345632494646 ) ) ;
#16648=CARTESIAN_POINT ( 'NONE',  ( 26.99999999999999645, 196.7750000012290741, -15.58845726811990495 ) ) ;
#16652=CARTESIAN_POINT ( 'NONE',  ( 23.87821517812499650, 243.8593750006145342, -4.985214923628404904 ) ) ;
#16658=CARTESIAN_POINT ( 'NONE',  ( 27.24356964375000700, 198.6968750006145115, 15.72908226750537075 ) ) ;
#16665=CYLINDRICAL_SURFACE ( 'NONE', #6684, 5.999999999999999112 ) ;
#16668=CARTESIAN_POINT ( 'NONE',  ( 20.99999999999999645, 242.4625000000000057, 5.999999999999998224 ) ) ;
#16674=CARTESIAN_POINT ( 'NONE',  ( 3.306546357697853733E-15, 210.0000000000000284, 27.00000000000000000 ) ) ;
#16675=EDGE_LOOP ( 'NONE', ( #2723, #33505, #9938, #22280, #1331 ) ) ;
#16678=CARTESIAN_POINT ( 'NONE',  ( -1.926257025242585782E-15, 197.0468750006145342, -31.45816453501076637 ) ) ;
#16682=CARTESIAN_POINT ( 'NONE',  ( 26.75643035624999655, 240.5968750006145456, 3.323476615752267715 ) ) ;
#16683=DIRECTION ( 'NONE',  ( -1.000000000000000000, -6.123233995736766036E-17, -0.000000000000000000 ) ) ;
#16688=VERTEX_POINT ( 'NONE', #27131 ) ;
#16689=CARTESIAN_POINT ( 'NONE',  ( 18.12178482187499640, 245.6218750006145228, -4.985214923628404904 ) ) ;
#16700=CARTESIAN_POINT ( 'NONE',  ( 23.87821517812499650, 245.0968750006145171, -4.985214923628404904 ) ) ;
#16701=AXIS2_PLACEMENT_3D ( 'NONE', #3787, #12325, #32602 ) ;
#16714=CARTESIAN_POINT ( 'NONE',  ( 26.99999999999999645, 245.8187500012290627, -3.464101615137755275 ) ) ;
#16716=FACE_OUTER_BOUND ( 'NONE', #28957, .T. ) ;
#16720=CARTESIAN_POINT ( 'NONE',  ( 19.39230484541326049, 242.3138461906613657, -5.999999999999997335 ) ) ;
#16721=CARTESIAN_POINT ( 'NONE',  ( -1.926257025242585782E-15, 197.0468750006145626, -31.45816453501075927 ) ) ;
#16726=ORIENTED_EDGE ( 'NONE', *, *, #33451, .T. ) ;
#16727=CARTESIAN_POINT ( 'NONE',  ( 15.00000000000000000, 241.9187500012290570, -3.464101615137752166 ) ) ;
#16732=EDGE_LOOP ( 'NONE', ( #30715, #3795, #9517 ) ) ;
#16737=DIRECTION ( 'NONE',  ( -0.000000000000000000, 1.000000000000000000, -0.000000000000000000 ) ) ;
#16744=CARTESIAN_POINT ( 'NONE',  ( -7.794140580174272692, 220.1661346705901678, -2.888490404254253185 ) ) ;
#16751=CARTESIAN_POINT ( 'NONE',  ( 19.95811783012822005, 240.0005236131589754, -5.908847734042844912 ) ) ;
#16760=CARTESIAN_POINT ( 'NONE',  ( 23.87821517812499650, 248.8093750006145228, -4.985214923628404904 ) ) ;
#16762=CARTESIAN_POINT ( 'NONE',  ( 23.87821517812499650, 241.1593750006145171, -4.985214923628404904 ) ) ;
#16763=VERTEX_POINT ( 'NONE', #29593 ) ;
#16767=CARTESIAN_POINT ( 'NONE',  ( 21.00000000000000000, 247.9187500012290570, 6.928203230275506996 ) ) ;
#16780=CARTESIAN_POINT ( 'NONE',  ( 20.99999999999999645, 185.0294372515228645, 0.000000000000000000 ) ) ;
#16781=CARTESIAN_POINT ( 'NONE',  ( 15.24356964374999990, 249.7468750006145228, 0.000000000000000000 ) ) ;
#16784=EDGE_CURVE ( 'NONE', #37177, #30702, #15586, .T. ) ;
#16785=CARTESIAN_POINT ( 'NONE',  ( 15.04813726045348687, 225.8716339721264319, 0.7835069059938112312 ) ) ;
#16787=CYLINDRICAL_SURFACE ( 'NONE', #32323, 5.999999999999999112 ) ;
#16792=ADVANCED_FACE ( 'NONE', ( #4932 ), #19371, .F. ) ;
#16794=CARTESIAN_POINT ( 'NONE',  ( 13.62178482187501416, 195.4531250006145342, 23.59362340125806767 ) ) ;
#16812=CARTESIAN_POINT ( 'NONE',  ( 15.00000000000000178, 249.1375000000000171, 3.464101615137757051 ) ) ;
#16814=CARTESIAN_POINT ( 'NONE',  ( -27.00000000000000355, 198.6125000000000398, -15.58845726811989429 ) ) ;
#16818=DIRECTION ( 'NONE',  ( 1.000000000000000000, 0.000000000000000000, 0.000000000000000000 ) ) ;
#16825=CARTESIAN_POINT ( 'NONE',  ( 26.99999999999999645, 243.5124999999999602, -3.464101615137755275 ) ) ;
#16826=CARTESIAN_POINT ( 'NONE',  ( -7.234628195640302017, 198.7424038105676800, 27.00000000000000711 ) ) ;
#16830=CARTESIAN_POINT ( 'NONE',  ( 27.00000000000001066, 196.2500000012290116, 15.58845726811988897 ) ) ;
#16835=CARTESIAN_POINT ( 'NONE',  ( 15.24356964374999990, 244.0093750006145399, 0.000000000000000000 ) ) ;
#16837=AXIS2_PLACEMENT_3D ( 'NONE', #25200, #19350, #4544 ) ;
#16842=ADVANCED_FACE ( 'NONE', ( #28061 ), #30731, .T. ) ;
#16845=CARTESIAN_POINT ( 'NONE',  ( -27.24356964375000345, 197.6093750006145342, 0.000000000000000000 ) ) ;
#16847=EDGE_CURVE ( 'NONE', #30367, #16244, #10480, .T. ) ;
#16859=CARTESIAN_POINT ( 'NONE',  ( 26.99999999999999645, 248.9125000000000227, -3.464101615137755275 ) ) ;
#16860=CARTESIAN_POINT ( 'NONE',  ( 3.306546357697853733E-15, 210.0000000000000284, 27.00000000000000000 ) ) ;
#16864=CARTESIAN_POINT ( 'NONE',  ( -27.24356964375000345, 195.8093750006145513, 0.000000000000000000 ) ) ;
#16868=CARTESIAN_POINT ( 'NONE',  ( 18.12178482187499640, 239.8843750006145115, -4.985214923628404904 ) ) ;
#16869=CARTESIAN_POINT ( 'NONE',  ( 27.24356964374999279, 199.1656250006145399, -15.72908226750539207 ) ) ;
#16873=VERTEX_POINT ( 'NONE', #13291 ) ;
#16875=CARTESIAN_POINT ( 'NONE',  ( 15.24356964375000167, 245.2843750006144887, 3.323476615752272600 ) ) ;
#16886=CARTESIAN_POINT ( 'NONE',  ( 26.75643035624999655, 243.6718750006145058, -7.049594010296217766E-16 ) ) ;
#16887=CARTESIAN_POINT ( 'NONE',  ( -3.253724281355068545E-15, 197.3000000012290229, -27.00000000000000000 ) ) ;
#16895=CARTESIAN_POINT ( 'NONE',  ( 20.99999999999999289, 244.5437500012290570, -5.999999999999997335 ) ) ;
#16905=CARTESIAN_POINT ( 'NONE',  ( 13.62178482187499640, 195.6593750006145456, -23.59362340125807123 ) ) ;
#16911=ORIENTED_EDGE ( 'NONE', *, *, #211, .T. ) ;
#16913=CARTESIAN_POINT ( 'NONE',  ( 18.00000000000000355, 241.1312500012290343, 5.196152422706632912 ) ) ;
#16918=EDGE_CURVE ( 'NONE', #16688, #8056, #28414, .T. ) ;
#16925=CARTESIAN_POINT ( 'NONE',  ( -10.06240783497716862, 195.0000000000000000, 25.33096707650729584 ) ) ;
#16930=LINE ( 'NONE', #20145, #27013 ) ;
#16944=CYLINDRICAL_SURFACE ( 'NONE', #12203, 5.999999999999999112 ) ;
#16945=CARTESIAN_POINT ( 'NONE',  ( 19.39230484541326760, 240.2486538117967427, 5.999999999999999112 ) ) ;
#16946=CARTESIAN_POINT ( 'NONE',  ( 26.75643035624999655, 246.9718750006145740, -3.323476615752271712 ) ) ;
#16948=CARTESIAN_POINT ( 'NONE',  ( 15.24356964374999990, 241.7593750006145399, 0.000000000000000000 ) ) ;
#16952=CARTESIAN_POINT ( 'NONE',  ( 21.00000000000000000, 249.2687500012290229, 6.928203230275506996 ) ) ;
#16956=DIRECTION ( 'NONE',  ( -0.000000000000000000, -0.000000000000000000, 1.000000000000000000 ) ) ;
#16959=ORIENTED_EDGE ( 'NONE', *, *, #15502, .F. ) ;
#16964=CARTESIAN_POINT ( 'NONE',  ( 22.60769515458672885, 248.0674038105676402, -6.000000000000000000 ) ) ;
#16965=CARTESIAN_POINT ( 'NONE',  ( 26.75643035624999655, 249.4843750006145058, 3.323476615752267715 ) ) ;
#16969=CARTESIAN_POINT ( 'NONE',  ( 15.80103094669415498, 223.8639174754799797, 3.001545256183678401 ) ) ;
#16994=CARTESIAN_POINT ( 'NONE',  ( -13.49999999999998401, 198.7250000000000227, 23.38268590217985476 ) ) ;
#16995=LINE ( 'NONE', #10557, #15981 ) ;
#16998=CARTESIAN_POINT ( 'NONE',  ( 26.75643035624999655, 249.1468750006145001, 3.323476615752267271 ) ) ;
#16999=ORIENTED_EDGE ( 'NONE', *, *, #13446, .T. ) ;
#17005=CARTESIAN_POINT ( 'NONE',  ( 18.00000000000000355, 243.3250000000000171, 5.196152422706632912 ) ) ;
#17011=CARTESIAN_POINT ( 'NONE',  ( -27.00000000000000355, 196.9625000012290172, 0.000000000000000000 ) ) ;
#17016=CARTESIAN_POINT ( 'NONE',  ( 23.87821517812499650, 242.0593750006145228, -4.985214923628404904 ) ) ;
#17024=CARTESIAN_POINT ( 'NONE',  ( 26.94731760015625355, 195.0000000000000284, -2.887353354705169739 ) ) ;
#17025=CARTESIAN_POINT ( 'NONE',  ( -13.62178482187498396, 197.2343750006145626, 23.59362340125808188 ) ) ;
#17027=VERTEX_POINT ( 'NONE', #17821 ) ;
#17028=( BOUNDED_CURVE ( )  B_SPLINE_CURVE ( 2, ( #1432, #18139, #1622, #33463, #13193, #12812, #24009, #24381, #12439 ),
 .UNSPECIFIED., .F., .F. ) 
 B_SPLINE_CURVE_WITH_KNOTS ( ( 3, 2, 2, 2, 3 ),
 ( 0.4791666666666666852, 0.4861111111111111049, 0.5000000000000000000, 0.5138888888888888395, 0.5208333333333333703 ),
 .UNSPECIFIED. ) 
 CURVE ( )  GEOMETRIC_REPRESENTATION_ITEM ( )  RATIONAL_B_SPLINE_CURVE ( ( 0.9330127018922194093, 0.9330127018922196314, 1.000000000000000000, 0.8660254037844387076, 1.000000000000000000, 0.8660254037844387076, 1.000000000000000000, 0.9330127018922187432, 0.9330127018922192983 ) ) 
 REPRESENTATION_ITEM ( '' )  );
#17031=EDGE_CURVE ( 'NONE', #19996, #35202, #6391, .T. ) ;
#17046=CARTESIAN_POINT ( 'NONE',  ( 27.24356964374999279, 195.1718750006145342, -15.72908226750539207 ) ) ;
#17050=CARTESIAN_POINT ( 'NONE',  ( 23.99999999999999645, 249.8499999999999943, -5.196152422706631135 ) ) ;
#17051=CARTESIAN_POINT ( 'NONE',  ( -1.926257025242585782E-15, 197.4406250006145740, -31.45816453501076637 ) ) ;
#17057=CARTESIAN_POINT ( 'NONE',  ( 21.00000000000000000, 241.3093750006145228, 6.646953231504538984 ) ) ;
#17067=CARTESIAN_POINT ( 'NONE',  ( 18.12178482187499640, 243.8218750006145399, -4.985214923628404904 ) ) ;
#17074=CARTESIAN_POINT ( 'NONE',  ( -3.253724281355068545E-15, 197.6374999999999602, -27.00000000000000355 ) ) ;
#17086=( BOUNDED_CURVE ( )  B_SPLINE_CURVE ( 2, ( #11300, #20026, #2758, #31571, #5594, #7717, #22689, #17180, #30838 ),
 .UNSPECIFIED., .F., .T. ) 
 B_SPLINE_CURVE_WITH_KNOTS ( ( 3, 2, 2, 2, 3 ),
 ( 0.5978260869565217295, 0.6014492753623188470, 0.6086956521739130821, 0.6159420289855072062, 0.6195652173913043237 ),
 .UNSPECIFIED. ) 
 CURVE ( )  GEOMETRIC_REPRESENTATION_ITEM ( )  RATIONAL_B_SPLINE_CURVE ( ( 0.9330127018922194093, 0.9330127018922194093, 1.000000000000000000, 0.8660254037844387076, 1.000000000000000000, 0.8660254037844387076, 1.000000000000000000, 0.9330127018922194093, 0.9330127018922194093 ) ) 
 REPRESENTATION_ITEM ( '' )  );
#17090=CARTESIAN_POINT ( 'NONE',  ( 18.00000000000000000, 242.3312500012290513, -5.196152422706630247 ) ) ;
#17091=CARTESIAN_POINT ( 'NONE',  ( -13.62178482187498396, 196.3343750006145285, 23.59362340125808188 ) ) ;
#17093=FACE_OUTER_BOUND ( 'NONE', #29440, .T. ) ;
#17097=ORIENTED_EDGE ( 'NONE', *, *, #18060, .F. ) ;
#17098=CARTESIAN_POINT ( 'NONE',  ( 18.12178482187500350, 249.3718750006145228, 4.985214923628407568 ) ) ;
#17113=VECTOR ( 'NONE', #23614, 1000.000000000000000 ) ;
#17116=ORIENTED_EDGE ( 'NONE', *, *, #2844, .T. ) ;
#17117=CARTESIAN_POINT ( 'NONE',  ( 10.49999999999999822, 222.9518338469886203, 2.500000000000000000 ) ) ;
#17126=VERTEX_POINT ( 'NONE', #6432 ) ;
#17133=CARTESIAN_POINT ( 'NONE',  ( 15.00000000000000178, 240.1937500012290627, 3.464101615137757051 ) ) ;
#17134=CARTESIAN_POINT ( 'NONE',  ( 26.75643035624999655, 245.5843750006145285, -7.049594010296217766E-16 ) ) ;
#17136=CARTESIAN_POINT ( 'NONE',  ( 26.75643035624999655, 241.9468750006145399, 3.323476615752267271 ) ) ;
#17140=CARTESIAN_POINT ( 'NONE',  ( 15.00000000000000000, 249.1562500012290400, 0.000000000000000000 ) ) ;
#17148=ORIENTED_EDGE ( 'NONE', *, *, #1109, .F. ) ;
#17157=CARTESIAN_POINT ( 'NONE',  ( 21.00000000000005329, 209.9999999999999716, -5.999999999999996447 ) ) ;
#17166=CARTESIAN_POINT ( 'NONE',  ( 1.069080835302379631E-14, 196.6250000012290400, 27.00000000000000000 ) ) ;
#17169=ORIENTED_EDGE ( 'NONE', *, *, #16559, .F. ) ;
#17180=CARTESIAN_POINT ( 'NONE',  ( 19.39230484541326049, 243.2138461906613713, -5.999999999999997335 ) ) ;
#17182=CARTESIAN_POINT ( 'NONE',  ( 27.00000000000000355, 198.4250000000000114, -3.306546357697854128E-15 ) ) ;
#17185=CARTESIAN_POINT ( 'NONE',  ( 23.87821517812499650, 249.2593750006145399, -4.985214923628404904 ) ) ;
#17192=CARTESIAN_POINT ( 'NONE',  ( 15.00000000000000178, 243.2874999999999943, 3.464101615137757051 ) ) ;
#17194=AXIS2_PLACEMENT_3D ( 'NONE', #34236, #36703, #19110 ) ;
#17196=ORIENTED_EDGE ( 'NONE', *, *, #27094, .T. ) ;
#17199=CARTESIAN_POINT ( 'NONE',  ( 13.50000000000001421, 196.2125000012290172, 23.38268590217984055 ) ) ;
#17203=CARTESIAN_POINT ( 'NONE',  ( 21.00000000000000000, 243.4468750006145683, -6.646953231504538984 ) ) ;
#17210=CARTESIAN_POINT ( 'NONE',  ( 23.54001937024031577, 195.0000000000001421, 13.61873700199885029 ) ) ;
#17211=CARTESIAN_POINT ( 'NONE',  ( 13.62178482187501416, 196.8593750006145342, 23.59362340125806767 ) ) ;
#17215=AXIS2_PLACEMENT_3D ( 'NONE', #16047, #4651, #19645 ) ;
#17218=CYLINDRICAL_SURFACE ( 'NONE', #9878, 27.00000000000000000 ) ;
#17233=CYLINDRICAL_SURFACE ( 'NONE', #16258, 5.999999999999999112 ) ;
#17236=CARTESIAN_POINT ( 'NONE',  ( 23.87821517812500005, 240.5593750006145228, 4.985214923628404016 ) ) ;
#17237=CARTESIAN_POINT ( 'NONE',  ( -27.24356964374999279, 198.0406250006145399, 15.72908226750539384 ) ) ;
#17240=EDGE_LOOP ( 'NONE', ( #19261, #19317, #24451, #35782 ) ) ;
#17241=ORIENTED_EDGE ( 'NONE', *, *, #31285, .T. ) ;
#17242=CARTESIAN_POINT ( 'NONE',  ( -27.24356964374999990, 197.5156250006145626, -15.72908226750537786 ) ) ;
#17243=CARTESIAN_POINT ( 'NONE',  ( 23.87821517812499650, 242.3968750006145285, -4.985214923628404904 ) ) ;
#17244=DIRECTION ( 'NONE',  ( 0.000000000000000000, -1.000000000000000000, 0.000000000000000000 ) ) ;
#17253=CARTESIAN_POINT ( 'NONE',  ( 15.24356964375000167, 240.7843750006145171, 3.323476615752272600 ) ) ;
#17259=CARTESIAN_POINT ( 'NONE',  ( 26.99999999999999645, 239.9687500012290116, -3.464101615137755275 ) ) ;
#17265=CARTESIAN_POINT ( 'NONE',  ( 23.99999999999999645, 244.5062500012290627, -5.196152422706631135 ) ) ;
#17267=VECTOR ( 'NONE', #35348, 1000.000000000000000 ) ;
#17270=ORIENTED_EDGE ( 'NONE', *, *, #2452, .F. ) ;
#17273=CARTESIAN_POINT ( 'NONE',  ( 26.99999999999999645, 243.9437500012290911, 3.464101615137751278 ) ) ;
#17274=CARTESIAN_POINT ( 'NONE',  ( 20.99999999999999645, 185.0294372515228645, 5.999999999999999112 ) ) ;
#17275=CARTESIAN_POINT ( 'NONE',  ( 27.24356964374999635, 196.5218750006145569, -15.72908226750539029 ) ) ;
#17276=CARTESIAN_POINT ( 'NONE',  ( 23.99999999999999645, 246.2500000000000000, -5.196152422706631135 ) ) ;
#17277=DIRECTION ( 'NONE',  ( -0.000000000000000000, 1.000000000000000000, -0.000000000000000000 ) ) ;
#17282=CARTESIAN_POINT ( 'NONE',  ( 18.12178482187500350, 248.4718750006145171, 4.985214923628407568 ) ) ;
#17287=ORIENTED_EDGE ( 'NONE', *, *, #33340, .F. ) ;
#17291=EDGE_CURVE ( 'NONE', #20196, #27300, #36369, .T. ) ;
#17295=CARTESIAN_POINT ( 'NONE',  ( -23.86618284116000410, 194.9999999999999147, 12.98668072022443987 ) ) ;
#17300=ORIENTED_EDGE ( 'NONE', *, *, #19209, .F. ) ;
#17301=CARTESIAN_POINT ( 'NONE',  ( 5.438367727407757144E-14, 197.7500000012290400, -27.00000000000000000 ) ) ;
#17313=CARTESIAN_POINT ( 'NONE',  ( 15.00000000000000000, 250.0000000000000000, 0.000000000000000000 ) ) ;
#17317=CARTESIAN_POINT ( 'NONE',  ( 21.00000000000000000, 246.1468750006145285, -6.646953231504538984 ) ) ;
#17319=CARTESIAN_POINT ( 'NONE',  ( 23.87821517812499650, 240.7093750006145285, -4.985214923628404904 ) ) ;
#17323=CARTESIAN_POINT ( 'NONE',  ( 24.00000000000000000, 247.0562500012290457, 5.196152422706629359 ) ) ;
#17331=ORIENTED_EDGE ( 'NONE', *, *, #11394, .F. ) ;
#17337=CARTESIAN_POINT ( 'NONE',  ( 26.75643035624999655, 246.8218750006145115, -7.049594010296217766E-16 ) ) ;
#17342=CARTESIAN_POINT ( 'NONE',  ( 18.18132103106268715, 212.8186789689449654, -5.491377079880368939 ) ) ;
#17355=CARTESIAN_POINT ( 'NONE',  ( 26.99999999999999645, 242.1812500012290457, -7.347880794884117764E-16 ) ) ;
#17366=CARTESIAN_POINT ( 'NONE',  ( 1.069080835302379631E-14, 195.6124999999999829, 27.00000000000000000 ) ) ;
#17368=CARTESIAN_POINT ( 'NONE',  ( 13.62178482187499640, 199.7093750006145285, -23.59362340125807123 ) ) ;
#17371=LINE ( 'NONE', #13789, #28828 ) ;
#17378=CARTESIAN_POINT ( 'NONE',  ( 21.00000000000000000, 241.5625000000000000, 6.928203230275506996 ) ) ;
#17386=CARTESIAN_POINT ( 'NONE',  ( -26.99999999999998934, 195.6500000012290457, 15.58845726811991561 ) ) ;
#17392=CARTESIAN_POINT ( 'NONE',  ( 15.24356964374999990, 240.8593750006145342, 0.000000000000000000 ) ) ;
#17401=CARTESIAN_POINT ( 'NONE',  ( -13.62178482187500528, 197.0843750006145285, -23.59362340125807123 ) ) ;
#17403=ORIENTED_EDGE ( 'NONE', *, *, #37465, .F. ) ;
#17412=FACE_OUTER_BOUND ( 'NONE', #18513, .T. ) ;
#17413=CARTESIAN_POINT ( 'NONE',  ( 0.000000000000000000, 210.0000000000000284, 0.000000000000000000 ) ) ;
#17415=CARTESIAN_POINT ( 'NONE',  ( 26.99999999999999645, 249.7375000000000114, 3.464101615137751278 ) ) ;
#17417=ORIENTED_EDGE ( 'NONE', *, *, #33554, .F. ) ;
#17420=CARTESIAN_POINT ( 'NONE',  ( 13.62178482187499640, 195.6593750006145456, -23.59362340125807123 ) ) ;
#17424=CARTESIAN_POINT ( 'NONE',  ( 18.00000000000000000, 249.4749999999999943, -5.196152422706630247 ) ) ;
#17425=CARTESIAN_POINT ( 'NONE',  ( 27.24356964375000700, 197.7406250006145285, 15.72908226750537075 ) ) ;
#17430=CARTESIAN_POINT ( 'NONE',  ( 27.24356964375000345, 197.7781250006145228, -3.336375036156643733E-15 ) ) ;
#17431=CARTESIAN_POINT ( 'NONE',  ( 18.12178482187499640, 243.3718750006145228, -4.985214923628404904 ) ) ;
#17434=CARTESIAN_POINT ( 'NONE',  ( 23.87821517812500005, 246.8593750006145342, 4.985214923628404016 ) ) ;
#17439=CARTESIAN_POINT ( 'NONE',  ( 20.99999999999999645, 240.8593750006145342, 6.646953231504538984 ) ) ;
#17445=DIRECTION ( 'NONE',  ( 2.335191374515007749E-05, 0.9999999997188656620, -4.117873977262775813E-06 ) ) ;
#17446=CARTESIAN_POINT ( 'NONE',  ( 10.49999999999999467, 222.9518338469886203, 12.50000000000000000 ) ) ;
#17450=DIRECTION ( 'NONE',  ( 0.000000000000000000, 0.000000000000000000, 1.000000000000000000 ) ) ;
#17455=CARTESIAN_POINT ( 'NONE',  ( 26.75643035624999655, 242.7718750006145001, -7.049594010296217766E-16 ) ) ;
#17460=CARTESIAN_POINT ( 'NONE',  ( -29.00000000000002487, 210.0000000000000000, -8.000000000000000000 ) ) ;
#17462=CARTESIAN_POINT ( 'NONE',  ( 13.62178482187499640, 195.2093750006145569, -23.59362340125807123 ) ) ;
#17468=EDGE_LOOP ( 'NONE', ( #27260, #8815, #18701, #35872 ) ) ;
#17470=CARTESIAN_POINT ( 'NONE',  ( 15.24356964375000167, 248.4343750006145228, 3.323476615752272600 ) ) ;
#17483=CARTESIAN_POINT ( 'NONE',  ( 18.12178482187499640, 249.6718750006145342, -4.985214923628404904 ) ) ;
#17484=CARTESIAN_POINT ( 'NONE',  ( -25.79889966451204586, 194.9999999999999147, 8.394779565232020957 ) ) ;
#17488=ORIENTED_EDGE ( 'NONE', *, *, #1909, .T. ) ;
#17489=CARTESIAN_POINT ( 'NONE',  ( -26.99999999999999645, 197.9000000012290457, 15.58845726811991561 ) ) ;
#17501=CARTESIAN_POINT ( 'NONE',  ( 7.234628195640322446, 195.2950961906613827, 26.99999999999999645 ) ) ;
#17504=CARTESIAN_POINT ( 'NONE',  ( 23.87821517812500005, 246.4093750006145171, 4.985214923628404016 ) ) ;
#17506=FACE_OUTER_BOUND ( 'NONE', #31717, .T. ) ;
#17510=CARTESIAN_POINT ( 'NONE',  ( 21.00000000000000000, 247.4687500012290684, 6.928203230275506996 ) ) ;
#17524=CARTESIAN_POINT ( 'NONE',  ( 26.75643035624999655, 246.4093750006145171, -3.323476615752271712 ) ) ;
#17528=CARTESIAN_POINT ( 'NONE',  ( 18.90563079128943968, 210.7853884532671884, -5.961323472697883652 ) ) ;
#17530=( BOUNDED_CURVE ( )  B_SPLINE_CURVE ( 2, ( #12651, #27424, #35197, #21384, #1081, #18162, #32737, #9433, #9621 ),
 .UNSPECIFIED., .F., .F. ) 
 B_SPLINE_CURVE_WITH_KNOTS ( ( 3, 2, 2, 2, 3 ),
 ( 0.8586956521739130821, 0.8623188405797101996, 0.8695652173913043237, 0.8768115942028985588, 0.8804347826086956763 ),
 .UNSPECIFIED. ) 
 CURVE ( )  GEOMETRIC_REPRESENTATION_ITEM ( )  RATIONAL_B_SPLINE_CURVE ( ( 0.9330127018922194093, 0.9330127018922194093, 1.000000000000000000, 0.8660254037844387076, 1.000000000000000000, 0.8660254037844387076, 1.000000000000000000, 0.9330127018922194093, 0.9330127018922194093 ) ) 
 REPRESENTATION_ITEM ( '' )  );
#17550=DIRECTION ( 'NONE',  ( -0.000000000000000000, -1.000000000000000000, -0.000000000000000000 ) ) ;
#17554=CARTESIAN_POINT ( 'NONE',  ( 26.99999999999999645, 195.7625000000000171, -15.58845726811990495 ) ) ;
#17557=CARTESIAN_POINT ( 'NONE',  ( 18.12178482187499640, 246.6343750006145115, -4.985214923628404904 ) ) ;
#17565=CARTESIAN_POINT ( 'NONE',  ( 15.00000000000000000, 241.9000000000000057, 0.000000000000000000 ) ) ;
#17571=EDGE_CURVE ( 'NONE', #2674, #14431, #12052, .T. ) ;
#17573=CARTESIAN_POINT ( 'NONE',  ( -27.00000000000000355, 196.5125000012290570, 0.000000000000000000 ) ) ;
#17577=CARTESIAN_POINT ( 'NONE',  ( 22.60769515458673595, 249.4174038105677198, -5.999999999999999112 ) ) ;
#17578=CARTESIAN_POINT ( 'NONE',  ( 26.75643035624999655, 240.1468750006145285, 3.323476615752267715 ) ) ;
#17587=DIRECTION ( 'NONE',  ( -0.000000000000000000, -1.000000000000000000, -0.000000000000000000 ) ) ;
#17588=CARTESIAN_POINT ( 'NONE',  ( 27.24356964375000345, 195.5843750006145285, -3.336375036156643733E-15 ) ) ;
#17594=CARTESIAN_POINT ( 'NONE',  ( 20.99999999999997868, 210.0000000000000000, 5.999999999999999112 ) ) ;
#17601=CARTESIAN_POINT ( 'NONE',  ( 21.00000000000000000, 249.4375000000000568, -5.999999999999998224 ) ) ;
#17611=CARTESIAN_POINT ( 'NONE',  ( -1.926257025242585782E-15, 195.2468750006145513, -31.45816453501076637 ) ) ;
#17615=CARTESIAN_POINT ( 'NONE',  ( 24.00000000000000000, 248.3499999999999943, 5.196152422706629359 ) ) ;
#17616=CARTESIAN_POINT ( 'NONE',  ( 13.62178482187499640, 199.2031250006145342, -23.59362340125807123 ) ) ;
#17621=ORIENTED_EDGE ( 'NONE', *, *, #29538, .T. ) ;
#17622=CARTESIAN_POINT ( 'NONE',  ( -1.926257025242585782E-15, 196.9906250006145569, -31.45816453501075927 ) ) ;
#17623=CARTESIAN_POINT ( 'NONE',  ( 15.24356964374999990, 242.0968750006145171, 0.000000000000000000 ) ) ;
#17626=CARTESIAN_POINT ( 'NONE',  ( 21.00000000000000000, 246.5968750006145456, -6.646953231504538984 ) ) ;
#17630=CARTESIAN_POINT ( 'NONE',  ( 26.75643035624999655, 241.8343750006145285, 3.323476615752267271 ) ) ;
#17638=CARTESIAN_POINT ( 'NONE',  ( 20.99999999999995381, 241.1687500012290570, 5.999999999999998224 ) ) ;
#17646=CARTESIAN_POINT ( 'NONE',  ( 18.12178482187499640, 242.0218750006145001, -4.985214923628404904 ) ) ;
#17651=DIRECTION ( 'NONE',  ( -0.000000000000000000, 1.000000000000000000, -0.000000000000000000 ) ) ;
#17652=CARTESIAN_POINT ( 'NONE',  ( -27.24356964375000345, 194.9093750006145456, 0.000000000000000000 ) ) ;
#17654=DIRECTION ( 'NONE',  ( -0.000000000000000000, -1.000000000000000000, -0.000000000000000000 ) ) ;
#17657=VERTEX_POINT ( 'NONE', #29105 ) ;
#17659=CARTESIAN_POINT ( 'NONE',  ( 23.99999999999999645, 240.0062500012290627, -5.196152422706631135 ) ) ;
#17664=CARTESIAN_POINT ( 'NONE',  ( 26.99999999999999645, 247.9749999999999943, -7.347880794884117764E-16 ) ) ;
#17671=CARTESIAN_POINT ( 'NONE',  ( 26.75643035624999655, 248.6593750006145171, -3.323476615752271268 ) ) ;
#17677=CARTESIAN_POINT ( 'NONE',  ( 21.00000000000000000, 241.6187500012290457, 5.999999999999998224 ) ) ;
#17680=VECTOR ( 'NONE', #30698, 1000.000000000000000 ) ;
#17686=CARTESIAN_POINT ( 'NONE',  ( 19.39230484541326049, 242.2575961894323200, -5.999999999999997335 ) ) ;
#17693=CARTESIAN_POINT ( 'NONE',  ( 15.24356964374999990, 246.2218750006145456, -3.323476615752268604 ) ) ;
#17695=VERTEX_POINT ( 'NONE', #2961 ) ;
#17697=CARTESIAN_POINT ( 'NONE',  ( 15.00000000000000000, 247.3562500012290570, 0.000000000000000000 ) ) ;
#17700=CARTESIAN_POINT ( 'NONE',  ( 7.234628195640337545, 198.1799038117967200, -26.99999999999999289 ) ) ;
#17705=ORIENTED_EDGE ( 'NONE', *, *, #175, .T. ) ;
#17708=CARTESIAN_POINT ( 'NONE',  ( 23.87821517812500005, 247.1968750006145115, 4.985214923628404016 ) ) ;
#17731=EDGE_CURVE ( 'NONE', #7355, #23955, #29633, .T. ) ;
#17735=AXIS2_PLACEMENT_3D ( 'NONE', #21606, #21979, #24805 ) ;
#17738=CARTESIAN_POINT ( 'NONE',  ( 27.00000000000001066, 196.5875000000000341, 15.58845726811988897 ) ) ;
#17739=CARTESIAN_POINT ( 'NONE',  ( 18.91622499444735439, 240.0135471875693725, -5.725135169889072451 ) ) ;
#17741=CARTESIAN_POINT ( 'NONE',  ( 23.87821517812499650, 247.0093750006145399, -4.985214923628404904 ) ) ;
#17748=CARTESIAN_POINT ( 'NONE',  ( 15.00000000000000000, 241.0000000000000000, 0.000000000000000000 ) ) ;
#17756=CARTESIAN_POINT ( 'NONE',  ( 7.234628195640363302, 195.3674038105676800, -26.99999999999996803 ) ) ;
#17761=CARTESIAN_POINT ( 'NONE',  ( 26.75643035624999655, 240.1843750006145513, -7.049594010296217766E-16 ) ) ;
#17769=CARTESIAN_POINT ( 'NONE',  ( 26.81003669216458718, 195.0000000000000000, 4.277059241843740978 ) ) ;
#17770=CARTESIAN_POINT ( 'NONE',  ( -13.62178482187498396, 195.4343750006145228, 23.59362340125808188 ) ) ;
#17775=CARTESIAN_POINT ( 'NONE',  ( -4.500000000000001776, 227.8255434699758837, -2.500000000000000000 ) ) ;
#17776=CARTESIAN_POINT ( 'NONE',  ( 7.234628195640322446, 198.7825961894323257, 26.99999999999999645 ) ) ;
#17784=CARTESIAN_POINT ( 'NONE',  ( 23.99999999999999645, 245.7999999999999829, -5.196152422706631135 ) ) ;
#17788=CARTESIAN_POINT ( 'NONE',  ( -27.00000000000000355, 195.0500000000000114, 0.000000000000000000 ) ) ;
#17796=CARTESIAN_POINT ( 'NONE',  ( 18.00000000000000000, 248.5749999999999886, -5.196152422706630247 ) ) ;
#17797=CARTESIAN_POINT ( 'NONE',  ( 27.24356964375000700, 195.0406250006145399, 15.72908226750537075 ) ) ;
#17803=CARTESIAN_POINT ( 'NONE',  ( -27.24356964374999635, 195.3406250006145513, 15.72908226750539384 ) ) ;
#17804=CARTESIAN_POINT ( 'NONE',  ( 23.87821517812499650, 241.4968750006144944, -4.985214923628404904 ) ) ;
#17808=CARTESIAN_POINT ( 'NONE',  ( 26.75643035624999655, 248.7343750006145342, -7.049594010296217766E-16 ) ) ;
#17810=CIRCLE ( 'NONE', #13558, 10.00000000000000888 ) ;
#17813=ADVANCED_FACE ( 'NONE', ( #21165 ), #24001, .F. ) ;
#17815=VECTOR ( 'NONE', #30247, 1000.000000000000000 ) ;
#17819=CARTESIAN_POINT ( 'NONE',  ( 15.24356964375000167, 241.6843750006145513, 3.323476615752272600 ) ) ;
#17821=CARTESIAN_POINT ( 'NONE',  ( 1.120210788295102201E-13, 197.1875000000000568, -27.00000000000000711 ) ) ;
#17824=EDGE_CURVE ( 'NONE', #3383, #29774, #7616, .T. ) ;
#17825=( BOUNDED_CURVE ( )  B_SPLINE_CURVE ( 2, ( #18924, #35767, #13226, #29902, #9811, #32930, #27622, #21761, #10184 ),
 .UNSPECIFIED., .F., .F. ) 
 B_SPLINE_CURVE_WITH_KNOTS ( ( 3, 2, 2, 2, 3 ),
 ( 0.1041666666666666713, 0.1111111111111111049, 0.1250000000000000000, 0.1388888888888888951, 0.1458333333333333426 ),
 .UNSPECIFIED. ) 
 CURVE ( )  GEOMETRIC_REPRESENTATION_ITEM ( )  RATIONAL_B_SPLINE_CURVE ( ( 0.9330127018922194093, 0.9330127018922194093, 1.000000000000000000, 0.8660254037844387076, 1.000000000000000000, 0.8660254037844387076, 1.000000000000000000, 0.9330127018922194093, 0.9330127018922194093 ) ) 
 REPRESENTATION_ITEM ( '' )  );
#17828=CARTESIAN_POINT ( 'NONE',  ( 19.39230484541323918, 240.9638461906613998, -5.999999999999987566 ) ) ;
#17834=CARTESIAN_POINT ( 'NONE',  ( 15.00000000000000000, 247.7687500012291082, -3.464101615137752610 ) ) ;
#17837=CARTESIAN_POINT ( 'NONE',  ( 23.87821517812500005, 241.3468750006145171, 4.985214923628404016 ) ) ;
#17838=EDGE_LOOP ( 'NONE', ( #12911, #6967, #22932, #5351, #27310, #15646, #17116, #18398, #4478, #25665, #15783, #4599, #10322, #27867, #28492, #27261, #32787, #8884, #12886, #2496, #3662, #34384, #16726, #26500, #26359 ) ) ;
#17843=FACE_OUTER_BOUND ( 'NONE', #30000, .T. ) ;
#17849=CARTESIAN_POINT ( 'NONE',  ( 15.00000000000000178, 239.7437500012290457, 3.464101615137757051 ) ) ;
#17860=CARTESIAN_POINT ( 'NONE',  ( 26.75643035624999655, 249.0343750006144887, 3.323476615752267271 ) ) ;
#17861=CARTESIAN_POINT ( 'NONE',  ( -15.87381995262718704, 194.9999999999999716, 22.12161802415705480 ) ) ;
#17866=CARTESIAN_POINT ( 'NONE',  ( -28.69006028236768913, 203.2074086957352108, 4.234161556416165872 ) ) ;
#17879=CARTESIAN_POINT ( 'NONE',  ( 15.00000000000000000, 249.9296875003072387, 0.000000000000000000 ) ) ;
#17882=CARTESIAN_POINT ( 'NONE',  ( 23.87821517812500005, 242.8093750006145228, 4.985214923628404016 ) ) ;
#17887=CARTESIAN_POINT ( 'NONE',  ( 23.99999999999999645, 247.2062500012290229, -5.196152422706631135 ) ) ;
#17896=VERTEX_POINT ( 'NONE', #24374 ) ;
#17899=CARTESIAN_POINT ( 'NONE',  ( 15.24356964374999990, 246.5968750006145171, 0.000000000000000000 ) ) ;
#17904=SURFACE_STYLE_USAGE ( .BOTH. , #12200 ) ;
#17917=CARTESIAN_POINT ( 'NONE',  ( 19.39230484541326760, 243.3424038105676743, 5.999999999999999112 ) ) ;
#17925=CARTESIAN_POINT ( 'NONE',  ( 20.99999999999999289, 241.3937500012289945, -5.999999999999997335 ) ) ;
#17929=CARTESIAN_POINT ( 'NONE',  ( 18.12178482187499640, 247.5343750006145456, -4.985214923628404904 ) ) ;
#17932=CARTESIAN_POINT ( 'NONE',  ( 20.99999999999997513, 244.9937500012290457, -5.999999999999999112 ) ) ;
#17936=CARTESIAN_POINT ( 'NONE',  ( 26.99999999999999645, 240.3250000000000171, -7.347880794884117764E-16 ) ) ;
#17943=CARTESIAN_POINT ( 'NONE',  ( 22.60769515458672529, 246.7174038105676743, -6.000000000000004441 ) ) ;
#17949=EDGE_CURVE ( 'NONE', #7130, #32512, #18132, .T. ) ;
#17951=CARTESIAN_POINT ( 'NONE',  ( 21.00000000000000000, 240.0718750006145399, 6.646953231504538984 ) ) ;
#17953=CARTESIAN_POINT ( 'NONE',  ( -4.499999999999999112, 226.9729365756407731, 2.499999999999999112 ) ) ;
#17960=CARTESIAN_POINT ( 'NONE',  ( 26.99999999999999645, 247.1125000000000114, -3.464101615137755275 ) ) ;
#17961=CARTESIAN_POINT ( 'NONE',  ( 27.24356964374999635, 196.5218750006145569, -15.72908226750539029 ) ) ;
#17966=CARTESIAN_POINT ( 'NONE',  ( 26.99999999999999645, 245.3687500012290457, -3.464101615137755275 ) ) ;
#17970=DIRECTION ( 'NONE',  ( 0.000000000000000000, 0.000000000000000000, -1.000000000000000000 ) ) ;
#17981=CARTESIAN_POINT ( 'NONE',  ( -13.50000000000000533, 195.5375000012290343, -23.38268590217984411 ) ) ;
#17987=CARTESIAN_POINT ( 'NONE',  ( 21.00000000000000000, 248.3124999999999716, 6.928203230275506996 ) ) ;
#17988=CARTESIAN_POINT ( 'NONE',  ( 13.62178482187501416, 195.4531250006145342, 23.59362340125806767 ) ) ;
#17992=CARTESIAN_POINT ( 'NONE',  ( -13.62178482187498396, 194.9281250006145569, 23.59362340125808188 ) ) ;
#17993=CARTESIAN_POINT ( 'NONE',  ( 20.00041244883536606, 239.7473985345926053, -5.668978318349186196 ) ) ;
#17995=EDGE_CURVE ( 'NONE', #24114, #26868, #26832, .T. ) ;
#17998=CARTESIAN_POINT ( 'NONE',  ( 26.75643035624999655, 247.8343750006145285, -7.049594010296217766E-16 ) ) ;
#18000=EDGE_CURVE ( 'NONE', #8445, #36238, #7950, .T. ) ;
#18004=CARTESIAN_POINT ( 'NONE',  ( 23.87821517812499650, 242.3968750006145285, -4.985214923628404904 ) ) ;
#18006=DIRECTION ( 'NONE',  ( -1.000000000000000000, 0.000000000000000000, 0.000000000000000000 ) ) ;
#18015=PLANE ( 'NONE',  #2495 ) ;
#18021=CARTESIAN_POINT ( 'NONE',  ( 26.75643035624999655, 241.8718750006145228, -7.049594010296217766E-16 ) ) ;
#18025=ADVANCED_FACE ( 'NONE', ( #12432, #35547 ), #9592, .F. ) ;
#18026=CARTESIAN_POINT ( 'NONE',  ( -13.62178482187498396, 199.0343750006145456, 23.59362340125808188 ) ) ;
#18028=FACE_OUTER_BOUND ( 'NONE', #10357, .T. ) ;
#18035=CARTESIAN_POINT ( 'NONE',  ( 15.24356964374999990, 246.5593750006144944, -3.323476615752268604 ) ) ;
#18040=CARTESIAN_POINT ( 'NONE',  ( 10.49999999999999822, 210.0000000000000284, 2.500000000000000000 ) ) ;
#18050=CARTESIAN_POINT ( 'NONE',  ( 18.12178482187500350, 249.3718750006145228, 4.985214923628407568 ) ) ;
#18051=CARTESIAN_POINT ( 'NONE',  ( 7.234628195640363302, 196.7174038105676459, -26.99999999999996803 ) ) ;
#18059=CARTESIAN_POINT ( 'NONE',  ( 15.00000000000000178, 249.1937500012290343, 3.464101615137757051 ) ) ;
#18060=EDGE_CURVE ( 'NONE', #24643, #36194, #10971, .T. ) ;
#18065=ORIENTED_EDGE ( 'NONE', *, *, #31699, .F. ) ;
#18077=ORIENTED_EDGE ( 'NONE', *, *, #22157, .F. ) ;
#18079=CARTESIAN_POINT ( 'NONE',  ( 21.00000000000000000, 243.1937500012290627, -6.928203230275506996 ) ) ;
#18082=CARTESIAN_POINT ( 'NONE',  ( 18.00000000000000355, 246.9250000000000114, 5.196152422706632912 ) ) ;
#18086=ORIENTED_EDGE ( 'NONE', *, *, #5692, .T. ) ;
#18091=CARTESIAN_POINT ( 'NONE',  ( 23.87821517812499650, 245.9968750006145228, -4.985214923628404904 ) ) ;
#18105=DIRECTION ( 'NONE',  ( -0.000000000000000000, 1.000000000000000000, -0.000000000000000000 ) ) ;
#18113=CYLINDRICAL_SURFACE ( 'NONE', #31106, 27.00000000000000000 ) ;
#18115=CARTESIAN_POINT ( 'NONE',  ( 26.99999999999999645, 195.7625000000000171, -15.58845726811990495 ) ) ;
#18119=CARTESIAN_POINT ( 'NONE',  ( 26.75643035624999655, 245.5843750006145285, -7.049594010296217766E-16 ) ) ;
#18120=EDGE_LOOP ( 'NONE', ( #18065, #23114, #32511, #23525 ) ) ;
#18126=CARTESIAN_POINT ( 'NONE',  ( 15.00000000000000178, 241.0374999999999943, 3.464101615137757051 ) ) ;
#18132=LINE ( 'NONE', #29674, #20646 ) ;
#18135=CARTESIAN_POINT ( 'NONE',  ( 15.00000000000000000, 248.1625000000000227, -3.464101615137752610 ) ) ;
#18139=CARTESIAN_POINT ( 'NONE',  ( -7.234628195640328663, 197.3924038105676857, 26.99999999999999289 ) ) ;
#18140=CARTESIAN_POINT ( 'NONE',  ( 26.75643035624999655, 241.5343750006145456, -7.049594010296217766E-16 ) ) ;
#18148=CARTESIAN_POINT ( 'NONE',  ( 20.99999999999997513, 247.1875000000000284, -5.999999999999999112 ) ) ;
#18150=CARTESIAN_POINT ( 'NONE',  ( 13.62178482187501416, 197.7031250006145342, 23.59362340125806767 ) ) ;
#18153=ORIENTED_EDGE ( 'NONE', *, *, #12470, .F. ) ;
#18159=DIRECTION ( 'NONE',  ( 0.000000000000000000, -1.000000000000000000, 0.000000000000000000 ) ) ;
#18162=CARTESIAN_POINT ( 'NONE',  ( 15.00000000000000000, 240.5687500012290343, -3.464101615137752610 ) ) ;
#18163=CARTESIAN_POINT ( 'NONE',  ( 26.99999999999999645, 244.7874999999999943, 3.464101615137751278 ) ) ;
#18175=CARTESIAN_POINT ( 'NONE',  ( 24.00000000000000000, 249.2500000000000000, 5.196152422706629359 ) ) ;
#18176=CARTESIAN_POINT ( 'NONE',  ( 27.24356964375000700, 195.9406250006145456, 15.72908226750537075 ) ) ;
#18177=EDGE_CURVE ( 'NONE', #8033, #36288, #19259, .T. ) ;
#18181=CARTESIAN_POINT ( 'NONE',  ( -20.86978604919638869, 194.8026013911397740, -17.51182792271053046 ) ) ;
#18182=CARTESIAN_POINT ( 'NONE',  ( 23.87821517812500005, 240.8968750006145285, 4.985214923628404016 ) ) ;
#18185=CARTESIAN_POINT ( 'NONE',  ( 15.24356964375000167, 246.7468750006145228, 3.323476615752272600 ) ) ;
#18193=CARTESIAN_POINT ( 'NONE',  ( 0.000000000000000000, 210.0000000000000284, 0.000000000000000000 ) ) ;
#18195=CARTESIAN_POINT ( 'NONE',  ( 2.999999999999997780, 244.5000000000000000, -2.500000000000000000 ) ) ;
#18210=CARTESIAN_POINT ( 'NONE',  ( 26.75643035624999655, 241.4218750006145058, -7.049594010296217766E-16 ) ) ;
#18215=EDGE_CURVE ( 'NONE', #3975, #2189, #14366, .T. ) ;
#18216=CARTESIAN_POINT ( 'NONE',  ( 13.62178482187499640, 199.7093750006145285, -23.59362340125807123 ) ) ;
#18224=ORIENTED_EDGE ( 'NONE', *, *, #18646, .F. ) ;
#18225=CARTESIAN_POINT ( 'NONE',  ( 23.87821517812499650, 245.9968750006145228, -4.985214923628404904 ) ) ;
#18231=ORIENTED_EDGE ( 'NONE', *, *, #18215, .F. ) ;
#18236=CARTESIAN_POINT ( 'NONE',  ( 20.99999999999999645, 248.2843750006145171, -6.646953231504538984 ) ) ;
#18238=CARTESIAN_POINT ( 'NONE',  ( -7.234628195640302017, 199.3049038117967200, 27.00000000000000711 ) ) ;
#18240=DIRECTION ( 'NONE',  ( 0.000000000000000000, 1.000000000000000000, 0.000000000000000000 ) ) ;
#18243=CARTESIAN_POINT ( 'NONE',  ( 20.99999999999999289, 241.8437500012290400, -5.999999999999997335 ) ) ;
#18252=CARTESIAN_POINT ( 'NONE',  ( 13.49999999999999645, 197.7125000012290172, -23.38268590217984766 ) ) ;
#18259=CARTESIAN_POINT ( 'NONE',  ( -27.00000000000000355, 200.0000000000000000, 0.000000000000000000 ) ) ;
#18262=DIRECTION ( 'NONE',  ( -0.000000000000000000, -1.000000000000000000, -0.000000000000000000 ) ) ;
#18263=ORIENTED_EDGE ( 'NONE', *, *, #28378, .T. ) ;
#18264=CARTESIAN_POINT ( 'NONE',  ( 18.00000000000000000, 244.5812500012290513, -5.196152422706630247 ) ) ;
#18267=CARTESIAN_POINT ( 'NONE',  ( -13.62178482187498396, 199.4281250006145569, 23.59362340125808188 ) ) ;
#18271=VERTEX_POINT ( 'NONE', #7246 ) ;
#18275=CARTESIAN_POINT ( 'NONE',  ( 21.00000000000000000, 244.6843750006144944, -6.646953231504538984 ) ) ;
#18282=EDGE_CURVE ( 'NONE', #35202, #22557, #23120, .T. ) ;
#18294=CARTESIAN_POINT ( 'NONE',  ( 20.99999999999998579, 248.3124999999999716, 5.999999999999998224 ) ) ;
#18301=CARTESIAN_POINT ( 'NONE',  ( 20.99999999999999645, 185.0294372515228645, 0.000000000000000000 ) ) ;
#18305=CARTESIAN_POINT ( 'NONE',  ( 18.12178482187499640, 249.7843750006145456, -4.985214923628404904 ) ) ;
#18307=CARTESIAN_POINT ( 'NONE',  ( 20.99999999999999645, 246.5968750006145456, -6.646953231504538984 ) ) ;
#18316=CARTESIAN_POINT ( 'NONE',  ( -11.18916359670908989, 217.4947517841555680, 4.100269900002030177 ) ) ;
#18319=ORIENTED_EDGE ( 'NONE', *, *, #28562, .F. ) ;
#18320=CARTESIAN_POINT ( 'NONE',  ( -27.00000000000000355, 195.9500000000000171, 0.000000000000000000 ) ) ;
#18321=CARTESIAN_POINT ( 'NONE',  ( 20.99999999999997513, 244.9937500012290457, -5.999999999999999112 ) ) ;
#18322=CARTESIAN_POINT ( 'NONE',  ( 19.39230484541326049, 248.1075961894323711, -5.999999999999994671 ) ) ;
#18326=CARTESIAN_POINT ( 'NONE',  ( 24.00000000000000000, 243.4562500012290513, 5.196152422706629359 ) ) ;
#18327=CARTESIAN_POINT ( 'NONE',  ( 18.90563079128947166, 210.7853884532676432, 5.961323472697788617 ) ) ;
#18329=CYLINDRICAL_SURFACE ( 'NONE', #1668, 27.00000000000000000 ) ;
#18334=CARTESIAN_POINT ( 'NONE',  ( 22.60769515458672529, 247.1674038105676630, -6.000000000000004441 ) ) ;
#18335=CARTESIAN_POINT ( 'NONE',  ( 13.62178482187501416, 199.0531250006145285, 23.59362340125806767 ) ) ;
#18340=CARTESIAN_POINT ( 'NONE',  ( -4.500000000000002665, 227.3990362376858627, -2.500000000000000000 ) ) ;
#18353=FACE_OUTER_BOUND ( 'NONE', #299, .T. ) ;
#18355=DIRECTION ( 'NONE',  ( -0.000000000000000000, 1.000000000000000000, -0.000000000000000000 ) ) ;
#18356=CARTESIAN_POINT ( 'NONE',  ( 20.99999999999997868, 244.7687500012290513, 5.999999999999999112 ) ) ;
#18361=CARTESIAN_POINT ( 'NONE',  ( 15.00000000000000000, 245.9499999999999886, 0.000000000000000000 ) ) ;
#18362=VECTOR ( 'NONE', #19702, 1000.000000000000000 ) ;
#18363=CARTESIAN_POINT ( 'NONE',  ( 5.778771075727756162E-15, 195.4156250006145399, 31.45816453501076637 ) ) ;
#18368=CARTESIAN_POINT ( 'NONE',  ( -13.62178482187498396, 195.3781250006145171, 23.59362340125808188 ) ) ;
#18372=CARTESIAN_POINT ( 'NONE',  ( 26.75643035624999655, 245.6218750006145513, -3.323476615752271712 ) ) ;
#18379=CARTESIAN_POINT ( 'NONE',  ( 18.12178482187500350, 240.3718750006145228, 4.985214923628407568 ) ) ;
#18381=( GEOMETRIC_REPRESENTATION_CONTEXT ( 3 ) GLOBAL_UNCERTAINTY_ASSIGNED_CONTEXT ( ( #12742 ) ) GLOBAL_UNIT_ASSIGNED_CONTEXT ( ( #3858, #20942, #12014 ) ) REPRESENTATION_CONTEXT ( 'NONE', 'WORKASPACE' ) );
#18385=DIRECTION ( 'NONE',  ( 0.000000000000000000, 0.000000000000000000, 1.000000000000000000 ) ) ;
#18393=DIRECTION ( 'NONE',  ( 0.000000000000000000, 0.000000000000000000, 1.000000000000000000 ) ) ;
#18397=CARTESIAN_POINT ( 'NONE',  ( 26.75643035624999655, 240.5218750006145001, -7.049594010296217766E-16 ) ) ;
#18398=ORIENTED_EDGE ( 'NONE', *, *, #8236, .T. ) ;
#18403=DIRECTION ( 'NONE',  ( -0.000000000000000000, 1.000000000000000000, -0.000000000000000000 ) ) ;
#18404=CYLINDRICAL_SURFACE ( 'NONE', #4724, 27.00000000000000000 ) ;
#18413=CARTESIAN_POINT ( 'NONE',  ( 26.75643035624999655, 245.9593750006145001, -3.323476615752271712 ) ) ;
#18428=CARTESIAN_POINT ( 'NONE',  ( 26.75643035624999655, 246.3343750006145285, 3.323476615752267271 ) ) ;
#18430=EDGE_CURVE ( 'NONE', #5908, #26373, #34714, .T. ) ;
#18436=CARTESIAN_POINT ( 'NONE',  ( 15.00000000000000000, 248.6125000000000114, -3.464101615137752610 ) ) ;
#18441=AXIS2_PLACEMENT_3D ( 'NONE', #3992, #21453, #21266 ) ;
#18452=CARTESIAN_POINT ( 'NONE',  ( 13.49999999999999645, 195.3500000000000227, -23.38268590217984766 ) ) ;
#18457=CARTESIAN_POINT ( 'NONE',  ( 0.000000000000000000, 210.0000000000000284, 0.000000000000000000 ) ) ;
#18459=CARTESIAN_POINT ( 'NONE',  ( 15.00000000000000000, 242.8562500012290286, 0.000000000000000000 ) ) ;
#18467=VERTEX_POINT ( 'NONE', #19381 ) ;
#18469=CARTESIAN_POINT ( 'NONE',  ( 21.00000000000000000, 244.9093750006145456, 6.646953231504538984 ) ) ;
#18484=CARTESIAN_POINT ( 'NONE',  ( 7.234628195640312676, 199.8674038105676800, -27.00000000000000711 ) ) ;
#18489=ORIENTED_EDGE ( 'NONE', *, *, #29560, .T. ) ;
#18500=CARTESIAN_POINT ( 'NONE',  ( 26.75643035624999655, 243.7468750006145228, 3.323476615752267271 ) ) ;
#18503=CARTESIAN_POINT ( 'NONE',  ( 15.00000000000000000, 245.1062500012290286, 0.000000000000000000 ) ) ;
#18513=EDGE_LOOP ( 'NONE', ( #32193, #33166, #18086, #11598 ) ) ;
#18517=CARTESIAN_POINT ( 'NONE',  ( 18.00000000000000000, 248.1250000000000000, -5.196152422706630247 ) ) ;
#18522=CARTESIAN_POINT ( 'NONE',  ( 8.278277990406262887, 214.7706457535967104, 3.659938751168453130 ) ) ;
#18532=CARTESIAN_POINT ( 'NONE',  ( -1.926257025242585782E-15, 199.6906250006145456, -31.45816453501075927 ) ) ;
#18535=ORIENTED_EDGE ( 'NONE', *, *, #14038, .F. ) ;
#18550=CARTESIAN_POINT ( 'NONE',  ( -1.909035429704832693E-15, 199.8875000000000171, -31.17691453623979214 ) ) ;
#18551=CARTESIAN_POINT ( 'NONE',  ( 15.24356964374999990, 249.8593750006145342, 0.000000000000000000 ) ) ;
#18559=CARTESIAN_POINT ( 'NONE',  ( 23.99999999999999645, 247.1500000000000057, -5.196152422706631135 ) ) ;
#18560=CARTESIAN_POINT ( 'NONE',  ( -27.24356964375000345, 196.2031250006145342, 0.000000000000000000 ) ) ;
#18567=CARTESIAN_POINT ( 'NONE',  ( -27.24356964374999635, 194.8906250006145342, 15.72908226750539384 ) ) ;
#18568=CARTESIAN_POINT ( 'NONE',  ( 26.75643035624999655, 240.9718750006145171, -7.049594010296217766E-16 ) ) ;
#18571=CARTESIAN_POINT ( 'NONE',  ( 21.00000000000000000, 244.3468750006145171, -6.646953231504538984 ) ) ;
#18587=CARTESIAN_POINT ( 'NONE',  ( 18.00000000000000355, 244.2249999999999943, 5.196152422706632912 ) ) ;
#18592=CARTESIAN_POINT ( 'NONE',  ( 26.75643035624999655, 240.0718750006145399, -7.049594010296217766E-16 ) ) ;
#18601=CARTESIAN_POINT ( 'NONE',  ( 23.87821517812500005, 242.3593750006145342, 4.985214923628404016 ) ) ;
#18607=CARTESIAN_POINT ( 'NONE',  ( 15.24356964375000167, 246.1843750006145513, 3.323476615752272600 ) ) ;
#18613=FACE_OUTER_BOUND ( 'NONE', #31787, .T. ) ;
#18621=CARTESIAN_POINT ( 'NONE',  ( 18.12178482187499640, 246.9718750006145171, -4.985214923628404904 ) ) ;
#18627=EDGE_CURVE ( 'NONE', #14808, #18936, #27422, .T. ) ;
#18629=ORIENTED_EDGE ( 'NONE', *, *, #24986, .T. ) ;
#18637=VERTEX_POINT ( 'NONE', #11937 ) ;
#18638=CARTESIAN_POINT ( 'NONE',  ( -4.694659320240884604E-14, 197.5250000012290172, 27.00000000000000000 ) ) ;
#18644=CARTESIAN_POINT ( 'NONE',  ( 27.00000000000001066, 195.6875000000000000, 15.58845726811988897 ) ) ;
#18646=EDGE_CURVE ( 'NONE', #25890, #18678, #35161, .T. ) ;
#18650=CARTESIAN_POINT ( 'NONE',  ( 15.00000000000000000, 244.1687500012290570, -3.464101615137752166 ) ) ;
#18653=CARTESIAN_POINT ( 'NONE',  ( 3.253724281355069334E-15, 199.5500000012290513, -27.00000000000000355 ) ) ;
#18658=CIRCLE ( 'NONE', #16837, 7.500000000000000000 ) ;
#18659=DIRECTION ( 'NONE',  ( -0.000000000000000000, -1.000000000000000000, -0.000000000000000000 ) ) ;
#18660=CARTESIAN_POINT ( 'NONE',  ( 15.24356964375000167, 243.9343750006145228, 3.323476615752272600 ) ) ;
#18664=CARTESIAN_POINT ( 'NONE',  ( 0.3500000000000069722, 244.5000000000000000, 2.500000000000000000 ) ) ;
#18668=VECTOR ( 'NONE', #11716, 1000.000000000000000 ) ;
#18678=VERTEX_POINT ( 'NONE', #20486 ) ;
#18679=VECTOR ( 'NONE', #14017, 1000.000000000000000 ) ;
#18684=CARTESIAN_POINT ( 'NONE',  ( 22.60769515458672885, 247.6174038105676516, -6.000000000000000000 ) ) ;
#18688=CARTESIAN_POINT ( 'NONE',  ( 15.24356964374999990, 249.3718750006145228, -3.323476615752268604 ) ) ;
#18690=CARTESIAN_POINT ( 'NONE',  ( 20.99999999999999645, 243.6718750006145058, 6.646953231504538984 ) ) ;
#18692=FACE_OUTER_BOUND ( 'NONE', #14009, .T. ) ;
#18699=ORIENTED_EDGE ( 'NONE', *, *, #34367, .T. ) ;
#18701=ORIENTED_EDGE ( 'NONE', *, *, #2517, .F. ) ;
#18702=VECTOR ( 'NONE', #12457, 1000.000000000000000 ) ;
#18705=CARTESIAN_POINT ( 'NONE',  ( 1.120210788295102201E-13, 195.0500000012290513, -27.00000000000000711 ) ) ;
#18707=CARTESIAN_POINT ( 'NONE',  ( 20.99999999999999645, 185.0294372515228645, -5.999999999999999112 ) ) ;
#18713=CARTESIAN_POINT ( 'NONE',  ( 14.04484906357221341, 216.9551509364261790, 0.1802446458343258673 ) ) ;
#18715=DIRECTION ( 'NONE',  ( 0.000000000000000000, 0.000000000000000000, -1.000000000000000000 ) ) ;
#18722=CARTESIAN_POINT ( 'NONE',  ( -1.926257025242585782E-15, 197.4406250006145740, -31.45816453501075927 ) ) ;
#18727=CARTESIAN_POINT ( 'NONE',  ( -13.50000000000000533, 197.6750000000000114, -23.38268590217984411 ) ) ;
#18734=CARTESIAN_POINT ( 'NONE',  ( 1.069080835302379631E-14, 198.8750000012290400, 27.00000000000000000 ) ) ;
#18738=CARTESIAN_POINT ( 'NONE',  ( -27.00000000000000355, 199.5124999999999886, -15.58845726811989429 ) ) ;
#18741=ORIENTED_EDGE ( 'NONE', *, *, #2507, .T. ) ;
#18748=CARTESIAN_POINT ( 'NONE',  ( 21.00000000000000000, 245.1625000000000227, 6.928203230275506996 ) ) ;
#18754=CARTESIAN_POINT ( 'NONE',  ( 27.00000000000001066, 198.0500000012290513, 15.58845726811988897 ) ) ;
#18755=CARTESIAN_POINT ( 'NONE',  ( -7.234628195640263826, 196.7575961894323484, -27.00000000000003553 ) ) ;
#18758=CARTESIAN_POINT ( 'NONE',  ( 21.00000000000000000, 246.3718750006145228, 6.646953231504538984 ) ) ;
#18766=CARTESIAN_POINT ( 'NONE',  ( 15.24356964375000167, 240.3343750006145285, 3.323476615752272600 ) ) ;
#18773=CYLINDRICAL_SURFACE ( 'NONE', #23770, 5.999999999999999112 ) ;
#18778=LINE ( 'NONE', #27470, #679 ) ;
#18782=CARTESIAN_POINT ( 'NONE',  ( 20.99999999999999289, 248.9874999999999829, -5.999999999999997335 ) ) ;
#18783=CARTESIAN_POINT ( 'NONE',  ( 26.75643035624999655, 240.9343750006144944, 3.323476615752267715 ) ) ;
#18790=CARTESIAN_POINT ( 'NONE',  ( 15.24356964374999990, 241.7593750006145399, 0.000000000000000000 ) ) ;
#18795=ORIENTED_EDGE ( 'NONE', *, *, #425, .F. ) ;
#18797=CARTESIAN_POINT ( 'NONE',  ( 23.87821517812500005, 246.2968750006145058, 4.985214923628404016 ) ) ;
#18802=ORIENTED_EDGE ( 'NONE', *, *, #3340, .T. ) ;
#18804=ORIENTED_EDGE ( 'NONE', *, *, #8505, .F. ) ;
#18810=CARTESIAN_POINT ( 'NONE',  ( 23.87821517812499650, 246.4468750006145115, -4.985214923628404904 ) ) ;
#18816=VERTEX_POINT ( 'NONE', #10030 ) ;
#18823=ORIENTED_EDGE ( 'NONE', *, *, #14956, .F. ) ;
#18829=CARTESIAN_POINT ( 'NONE',  ( 3.551475717527324030E-15, 210.0000000000000284, 28.99999999999999645 ) ) ;
#18830=CARTESIAN_POINT ( 'NONE',  ( -1.926257025242585782E-15, 197.4968750006145513, -31.45816453501075927 ) ) ;
#18832=CARTESIAN_POINT ( 'NONE',  ( 26.99999999999999645, 243.9250000000000114, -7.347880794884117764E-16 ) ) ;
#18836=CARTESIAN_POINT ( 'NONE',  ( 21.00000000000000000, 244.3187500012290627, 6.928203230275506996 ) ) ;
#18842=AXIS2_PLACEMENT_3D ( 'NONE', #7979, #13856, #16327 ) ;
#18845=CARTESIAN_POINT ( 'NONE',  ( 21.00000000000000000, 245.3593750006145342, 6.646953231504538984 ) ) ;
#18857=CARTESIAN_POINT ( 'NONE',  ( 20.99999999999999645, 185.0294372515228645, 0.000000000000000000 ) ) ;
#18861=CARTESIAN_POINT ( 'NONE',  ( -28.26183920611484979, 205.3333679525152888, -6.503129933765640303 ) ) ;
#18863=ORIENTED_EDGE ( 'NONE', *, *, #37125, .F. ) ;
#18867=DIRECTION ( 'NONE',  ( 1.000000000000000000, 0.000000000000000000, 0.000000000000000000 ) ) ;
#18873=CARTESIAN_POINT ( 'NONE',  ( 26.75643035624999655, 245.0968750006145456, 3.323476615752267271 ) ) ;
#18887=CARTESIAN_POINT ( 'NONE',  ( 20.99999999999999645, 185.0294372515228645, -5.999999999999999112 ) ) ;
#18895=CARTESIAN_POINT ( 'NONE',  ( 17.03503949639500448, 220.5732280096259217, 4.520320870633568688 ) ) ;
#18905=CARTESIAN_POINT ( 'NONE',  ( -27.24356964375000345, 199.8031250006145285, 0.000000000000000000 ) ) ;
#18912=LINE ( 'NONE', #33110, #18702 ) ;
#18919=CARTESIAN_POINT ( 'NONE',  ( 15.00000000000000000, 246.3625000000000114, -3.464101615137752610 ) ) ;
#18924=CARTESIAN_POINT ( 'NONE',  ( 1.255007937094097924E-14, 199.4375000000000284, -27.00000000000000000 ) ) ;
#18931=CARTESIAN_POINT ( 'NONE',  ( 26.99999999999999645, 245.7624999999999886, -3.464101615137755275 ) ) ;
#18936=VERTEX_POINT ( 'NONE', #6255 ) ;
#18937=CARTESIAN_POINT ( 'NONE',  ( -27.00000000000000355, 198.7250000012290059, -15.58845726811989429 ) ) ;
#18942=CARTESIAN_POINT ( 'NONE',  ( 18.12178482187500350, 245.8843750006145115, 4.985214923628407568 ) ) ;
#18949=CARTESIAN_POINT ( 'NONE',  ( 5.438367727407757144E-14, 198.0875000000000057, -27.00000000000000000 ) ) ;
#18953=CARTESIAN_POINT ( 'NONE',  ( 1.069080835302379631E-14, 196.9624999999999773, 27.00000000000000000 ) ) ;
#18960=EDGE_CURVE ( 'NONE', #1148, #7787, #32507, .T. ) ;
#18963=CARTESIAN_POINT ( 'NONE',  ( 20.00041297495057080, 239.7473985277379143, -5.668978411116884608 ) ) ;
#18967=CARTESIAN_POINT ( 'NONE',  ( -27.24356964374999279, 197.1968750006145115, 15.72908226750539384 ) ) ;
#18969=CARTESIAN_POINT ( 'NONE',  ( 0.000000000000000000, 210.0000000000000284, 0.000000000000000000 ) ) ;
#18970=CARTESIAN_POINT ( 'NONE',  ( 18.12178482187499640, 243.0343750006145456, -4.985214923628404904 ) ) ;
#18975=CARTESIAN_POINT ( 'NONE',  ( 18.12178482187500350, 243.5218750006145001, 4.985214923628407568 ) ) ;
#18977=EDGE_CURVE ( 'NONE', #30621, #21071, #36386, .T. ) ;
#18985=VERTEX_POINT ( 'NONE', #6443 ) ;
#18992=CARTESIAN_POINT ( 'NONE',  ( 15.24356964374999990, 246.1468750006145285, 0.000000000000000000 ) ) ;
#18998=CARTESIAN_POINT ( 'NONE',  ( -27.24356964375000345, 199.8593750006145342, 0.000000000000000000 ) ) ;
#19009=FACE_OUTER_BOUND ( 'NONE', #12548, .T. ) ;
#19013=CARTESIAN_POINT ( 'NONE',  ( -27.24356964375000345, 198.5093750006145399, 0.000000000000000000 ) ) ;
#19015=CARTESIAN_POINT ( 'NONE',  ( 15.00000000000000000, 249.9625000000000057, -3.464101615137752610 ) ) ;
#19017=CARTESIAN_POINT ( 'NONE',  ( 23.99999999999999645, 242.1999999999999886, -5.196152422706631135 ) ) ;
#19020=CARTESIAN_POINT ( 'NONE',  ( 21.00000000000000000, 240.4937500012290457, -6.928203230275506996 ) ) ;
#19023=CARTESIAN_POINT ( 'NONE',  ( -1.926257025242585782E-15, 199.6906250006145456, -31.45816453501075927 ) ) ;
#19050=( BOUNDED_CURVE ( )  B_SPLINE_CURVE ( 2, ( #6420, #24970, #22150, #7553, #10203, #13052, #16462, #4512, #7367 ),
 .UNSPECIFIED., .F., .F. ) 
 B_SPLINE_CURVE_WITH_KNOTS ( ( 3, 2, 2, 2, 3 ),
 ( 0.07608695652173913526, 0.07971014492753622505, 0.08695652173913043237, 0.09420289855072463969, 0.09782608695652174335 ),
 .UNSPECIFIED. ) 
 CURVE ( )  GEOMETRIC_REPRESENTATION_ITEM ( )  RATIONAL_B_SPLINE_CURVE ( ( 0.9330127018922192983, 0.9330127018922194093, 1.000000000000000000, 0.8660254037844387076, 1.000000000000000000, 0.8660254037844387076, 1.000000000000000000, 0.9330127018922194093, 0.9330127018922194093 ) ) 
 REPRESENTATION_ITEM ( '' )  );
#19059=CARTESIAN_POINT ( 'NONE',  ( 18.12178482187499640, 247.5343750006145456, -4.985214923628404904 ) ) ;
#19061=CARTESIAN_POINT ( 'NONE',  ( 18.12178482187499640, 243.4843750006145342, -4.985214923628404904 ) ) ;
#19072=VERTEX_POINT ( 'NONE', #16668 ) ;
#19075=CARTESIAN_POINT ( 'NONE',  ( 1.069080835302379631E-14, 199.3250000012290286, 27.00000000000000000 ) ) ;
#19081=CARTESIAN_POINT ( 'NONE',  ( 16.34449471652106567, 214.6555052834588935, 4.429144169335408776 ) ) ;
#19089=CARTESIAN_POINT ( 'NONE',  ( -27.24356964375000345, 195.3031250006145285, 0.000000000000000000 ) ) ;
#19093=VECTOR ( 'NONE', #18262, 1000.000000000000000 ) ;
#19094=FACE_OUTER_BOUND ( 'NONE', #32004, .T. ) ;
#19109=CARTESIAN_POINT ( 'NONE',  ( -27.00000000000000355, 199.9625000000000341, -15.58845726811989429 ) ) ;
#19110=DIRECTION ( 'NONE',  ( 0.000000000000000000, 0.000000000000000000, 1.000000000000000000 ) ) ;
#19113=LINE ( 'NONE', #16262, #24010 ) ;
#19118=CARTESIAN_POINT ( 'NONE',  ( 23.99999999999999645, 245.7999999999999829, -5.196152422706631135 ) ) ;
#19126=CARTESIAN_POINT ( 'NONE',  ( -27.00000000000000355, 197.3750000012290400, -15.58845726811989429 ) ) ;
#19131=AXIS2_PLACEMENT_3D ( 'NONE', #8430, #14116, #25299 ) ;
#19132=CARTESIAN_POINT ( 'NONE',  ( 15.24356964374999990, 244.9093750006145171, 0.000000000000000000 ) ) ;
#19138=CARTESIAN_POINT ( 'NONE',  ( -13.62178482187498396, 198.1343750006145399, 23.59362340125808188 ) ) ;
#19153=CARTESIAN_POINT ( 'NONE',  ( 15.24356964374999990, 240.2968750006145342, 0.000000000000000000 ) ) ;
#19157=CARTESIAN_POINT ( 'NONE',  ( 27.24356964375000345, 198.7343750006145626, -3.336375036156643733E-15 ) ) ;
#19161=DIRECTION ( 'NONE',  ( -0.000000000000000000, -1.000000000000000000, -0.000000000000000000 ) ) ;
#19162=CARTESIAN_POINT ( 'NONE',  ( 26.75643035624999655, 243.2968750006145342, 3.323476615752267715 ) ) ;
#19167=CARTESIAN_POINT ( 'NONE',  ( 21.00000000000000000, 244.9093750006145456, 6.646953231504538984 ) ) ;
#19182=CARTESIAN_POINT ( 'NONE',  ( 15.24356964374999990, 245.2468750006145228, 0.000000000000000000 ) ) ;
#19191=VECTOR ( 'NONE', #17445, 1000.000000000000000 ) ;
#19202=CARTESIAN_POINT ( 'NONE',  ( 18.00000000000000000, 244.9749999999999943, -5.196152422706630247 ) ) ;
#19203=CARTESIAN_POINT ( 'NONE',  ( 13.62178482187499640, 198.3593750006145342, -23.59362340125807123 ) ) ;
#19204=CARTESIAN_POINT ( 'NONE',  ( 20.99999999999999289, 249.8874999999999886, -5.999999999999997335 ) ) ;
#19209=EDGE_CURVE ( 'NONE', #28635, #24921, #4728, .T. ) ;
#19211=CARTESIAN_POINT ( 'NONE',  ( 26.99999999999999645, 242.1437500012290513, 3.464101615137751278 ) ) ;
#19214=CARTESIAN_POINT ( 'NONE',  ( -1.926257025242585782E-15, 199.2406250006145285, -31.45816453501075927 ) ) ;
#19239=CARTESIAN_POINT ( 'NONE',  ( -28.94388556517004929, 202.2057090852030399, -1.821689022226129051 ) ) ;
#19245=CARTESIAN_POINT ( 'NONE',  ( 26.99999999999999645, 247.5625000000000000, -3.464101615137755275 ) ) ;
#19246=CARTESIAN_POINT ( 'NONE',  ( 20.99999999999999645, 185.0294372515228645, -5.999999999999999112 ) ) ;
#19250=CARTESIAN_POINT ( 'NONE',  ( 18.12178482187499640, 247.0843750006145285, -4.985214923628404904 ) ) ;
#19252=CARTESIAN_POINT ( 'NONE',  ( 15.24356964375000167, 243.1468750006145285, 3.323476615752272600 ) ) ;
#19253=ORIENTED_EDGE ( 'NONE', *, *, #15680, .T. ) ;
#19254=CARTESIAN_POINT ( 'NONE',  ( 20.99999999999999289, 249.4937500012290457, -5.999999999999998224 ) ) ;
#19255=CARTESIAN_POINT ( 'NONE',  ( 18.00000000000000000, 249.5312500012290684, -5.196152422706630247 ) ) ;
#19259=( BOUNDED_CURVE ( )  B_SPLINE_CURVE ( 2, ( #21286, #6675, #12553, #18059, #24307, #15402, #3639, #30174, #26567 ),
 .UNSPECIFIED., .F., .F. ) 
 B_SPLINE_CURVE_WITH_KNOTS ( ( 3, 2, 2, 2, 3 ),
 ( 0.03260869565217391908, 0.03623188405797101580, 0.04347826086956521618, 0.05072463768115942351, 0.05434782608695652717 ),
 .UNSPECIFIED. ) 
 CURVE ( )  GEOMETRIC_REPRESENTATION_ITEM ( )  RATIONAL_B_SPLINE_CURVE ( ( 0.9330127018922192983, 0.9330127018922194093, 1.000000000000000000, 0.8660254037844387076, 1.000000000000000000, 0.8660254037844387076, 1.000000000000000000, 0.9330127018922192983, 0.9330127018922194093 ) ) 
 REPRESENTATION_ITEM ( '' )  );
#19261=ORIENTED_EDGE ( 'NONE', *, *, #13347, .F. ) ;
#19269=CARTESIAN_POINT ( 'NONE',  ( 26.75643035624999655, 249.1093750006145058, -3.323476615752271712 ) ) ;
#19273=CARTESIAN_POINT ( 'NONE',  ( 14.20575797956217734, 216.7942420204455232, -0.4629122958956893297 ) ) ;
#19280=( BOUNDED_CURVE ( )  B_SPLINE_CURVE ( 2, ( #6165, #35151, #3133, #31574, #15075, #34971, #5597, #17739, #23420 ),
 .UNSPECIFIED., .F., .F. ) 
 B_SPLINE_CURVE_WITH_KNOTS ( ( 3, 2, 2, 2, 3 ),
 ( 0.9456521739130434590, 0.9492753623188405765, 0.9565217391304348116, 0.9637681159420289356, 0.9662082973083874204 ),
 .UNSPECIFIED. ) 
 CURVE ( )  GEOMETRIC_REPRESENTATION_ITEM ( )  RATIONAL_B_SPLINE_CURVE ( ( 0.9330127018922194093, 0.9330127018922194093, 1.000000000000000000, 0.8660254037844387076, 1.000000000000000000, 0.8660254037844387076, 1.000000000000000000, 0.9548847207714155072, 0.9401541335272467492 ) ) 
 REPRESENTATION_ITEM ( '' )  );
#19283=CARTESIAN_POINT ( 'NONE',  ( 27.24356964375000345, 197.3281250006145342, -3.336375036156643733E-15 ) ) ;
#19284=AXIS2_PLACEMENT_3D ( 'NONE', #13127, #7999, #7442 ) ;
#19302=CARTESIAN_POINT ( 'NONE',  ( -26.99999999999998934, 198.6875000000000284, 15.58845726811991561 ) ) ;
#19303=CLOSED_SHELL ( 'NONE', ( #28817, #22699, #9125, #24105, #28247, #34689, #10527, #27897, #13114, #14120, #11063, #29122, #25455, #4128, #32530, #3585, #8016, #37211, #146, #4996, #33343, #22387, #27643, #11086, #20374, #22614, #7295, #34734, #21533, #36905, #15385, #6421, #7326, #6118, #17813, #25126, #31041, #8663, #24699, #120, #4844, #31412, #4674, #9035, #22476, #31826, #9248, #20240, #15065, #4761, #35498, #1579, #9711, #37428, #819, #16096, #2461, #13398, #30087, #2903, #3790, #24728, #35808, #13528, #13657, #1621, #21654, #20052, #35650, #35085, #25784, #10813, #37420, #24696, #29392, #18025, #21406, #35302, #29589, #26345, #21939, #13878, #32121, #24880, #37049, #28443, #9501, #36928, #16842, #36959, #6324, #14804, #29648, #24271, #25105, #31425, #6589, #16792, #557, #23698, #33034, #2183, #6455, #32343, #32858, #35641 ) ) ;
#19306=CARTESIAN_POINT ( 'NONE',  ( 15.00000000000000178, 241.9375000000000000, 3.464101615137757051 ) ) ;
#19307=ORIENTED_EDGE ( 'NONE', *, *, #16918, .T. ) ;
#19309=CARTESIAN_POINT ( 'NONE',  ( 20.99999999999999645, 247.4687500012290400, 5.999999999999998224 ) ) ;
#19312=CARTESIAN_POINT ( 'NONE',  ( 18.00000000000000000, 243.1750000000000114, -5.196152422706630247 ) ) ;
#19316=ORIENTED_EDGE ( 'NONE', *, *, #10646, .F. ) ;
#19317=ORIENTED_EDGE ( 'NONE', *, *, #23727, .T. ) ;
#19318=CARTESIAN_POINT ( 'NONE',  ( -13.50000000000000533, 198.2375000012290229, -23.38268590217984411 ) ) ;
#19323=CARTESIAN_POINT ( 'NONE',  ( 15.24356964374999990, 242.6593750006145171, 0.000000000000000000 ) ) ;
#19325=DIRECTION ( 'NONE',  ( -0.000000000000000000, 1.000000000000000000, -0.000000000000000000 ) ) ;
#19329=CARTESIAN_POINT ( 'NONE',  ( -1.926257025242585782E-15, 197.9468750006145399, -31.45816453501075927 ) ) ;
#19333=CARTESIAN_POINT ( 'NONE',  ( 20.99999999999997513, 245.3875000000000455, -5.999999999999999112 ) ) ;
#19347=CARTESIAN_POINT ( 'NONE',  ( -13.62178482187500528, 198.4343750006145228, -23.59362340125807123 ) ) ;
#19348=FACE_OUTER_BOUND ( 'NONE', #30284, .T. ) ;
#19350=DIRECTION ( 'NONE',  ( 0.000000000000000000, 0.000000000000000000, -1.000000000000000000 ) ) ;
#19351=CARTESIAN_POINT ( 'NONE',  ( 20.00041297495047843, 239.8598985277378972, -5.668978411116867733 ) ) ;
#19357=CARTESIAN_POINT ( 'NONE',  ( 18.12178482187499640, 245.1718750006145058, -4.985214923628404904 ) ) ;
#19370=CARTESIAN_POINT ( 'NONE',  ( 18.12178482187499640, 245.1718750006145058, -4.985214923628404904 ) ) ;
#19371=CYLINDRICAL_SURFACE ( 'NONE', #7930, 10.00000000000000000 ) ;
#19381=CARTESIAN_POINT ( 'NONE',  ( 19.95811093400027403, 239.6067736145540152, -5.908846518073574750 ) ) ;
#19391=CARTESIAN_POINT ( 'NONE',  ( 13.62178482187501416, 199.1093750006145342, 23.59362340125806767 ) ) ;
#19396=ORIENTED_EDGE ( 'NONE', *, *, #21864, .T. ) ;
#19397=CARTESIAN_POINT ( 'NONE',  ( 26.99999999999999645, 242.1812500012290457, -7.347880794884117764E-16 ) ) ;
#19400=CARTESIAN_POINT ( 'NONE',  ( 13.62178482187501416, 197.7031250006145342, 23.59362340125806767 ) ) ;
#19426=CARTESIAN_POINT ( 'NONE',  ( 5.000000000000127010, 225.9999999999999432, -7.999999999999940492 ) ) ;
#19427=CARTESIAN_POINT ( 'NONE',  ( 20.99999999999999645, 245.6125000000000114, 5.999999999999998224 ) ) ;
#19429=CARTESIAN_POINT ( 'NONE',  ( 21.00000000000000000, 247.9468750006145399, -6.646953231504538984 ) ) ;
#19431=CARTESIAN_POINT ( 'NONE',  ( 15.24356964374999990, 242.6218750006145228, -3.323476615752268604 ) ) ;
#19436=CARTESIAN_POINT ( 'NONE',  ( 26.99999999999999645, 248.4437500012290343, 3.464101615137751278 ) ) ;
#19444=ORIENTED_EDGE ( 'NONE', *, *, #35164, .T. ) ;
#19445=ORIENTED_EDGE ( 'NONE', *, *, #10047, .F. ) ;
#19449=CARTESIAN_POINT ( 'NONE',  ( 7.234628195640269155, 195.1825961894323598, 27.00000000000003197 ) ) ;
#19450=CARTESIAN_POINT ( 'NONE',  ( 18.12178482187500350, 248.4718750006145171, 4.985214923628407568 ) ) ;
#19455=CARTESIAN_POINT ( 'NONE',  ( 15.61591388112560530, 224.3575629836672931, 2.655215585728335714 ) ) ;
#19461=EDGE_CURVE ( 'NONE', #11819, #14431, #37152, .T. ) ;
#19464=CARTESIAN_POINT ( 'NONE',  ( -13.62178482187498396, 196.2781250006145228, 23.59362340125808188 ) ) ;
#19481=CARTESIAN_POINT ( 'NONE',  ( -26.99999999999998934, 196.8875000000000171, 15.58845726811991561 ) ) ;
#19482=FACE_OUTER_BOUND ( 'NONE', #16311, .T. ) ;
#19486=ORIENTED_EDGE ( 'NONE', *, *, #23681, .F. ) ;
#19493=CARTESIAN_POINT ( 'NONE',  ( 26.99999999999999645, 243.8875000000000171, 3.464101615137751278 ) ) ;
#19499=CARTESIAN_POINT ( 'NONE',  ( -27.00000000000000355, 198.2750000012290741, -15.58845726811989429 ) ) ;
#19503=CARTESIAN_POINT ( 'NONE',  ( 18.12178482187499640, 243.4843750006145342, -4.985214923628404904 ) ) ;
#19510=CARTESIAN_POINT ( 'NONE',  ( 27.24356964375000700, 199.5968750006145456, 15.72908226750537075 ) ) ;
#19515=CARTESIAN_POINT ( 'NONE',  ( 26.99999999999999645, 245.3125000000000000, -3.464101615137755275 ) ) ;
#19524=CARTESIAN_POINT ( 'NONE',  ( 17.54540804174073187, 195.0000000000000000, -20.52215039046394907 ) ) ;
#19529=CARTESIAN_POINT ( 'NONE',  ( -27.24356964375000345, 197.1218750006145513, -15.72908226750537786 ) ) ;
#19532=CARTESIAN_POINT ( 'NONE',  ( 23.87821517812499650, 241.1593750006145171, -4.985214923628404904 ) ) ;
#19539=CARTESIAN_POINT ( 'NONE',  ( 23.87821517812499650, 244.6468750006145285, -4.985214923628404904 ) ) ;
#19551=CARTESIAN_POINT ( 'NONE',  ( 26.75643035624999655, 244.1593750006145171, -3.323476615752271268 ) ) ;
#19566=CYLINDRICAL_SURFACE ( 'NONE', #34279, 5.999999999999999112 ) ;
#19570=CARTESIAN_POINT ( 'NONE',  ( 27.24356964375000345, 196.9343750006145228, -3.336375036156643733E-15 ) ) ;
#19572=CARTESIAN_POINT ( 'NONE',  ( 26.99999999999999645, 242.1250000000000000, -7.347880794884117764E-16 ) ) ;
#19577=CARTESIAN_POINT ( 'NONE',  ( 24.00000000000000000, 242.1062500012290286, 5.196152422706629359 ) ) ;
#19582=AXIS2_PLACEMENT_3D ( 'NONE', #4850, #2006, #4294 ) ;
#19586=EDGE_CURVE ( 'NONE', #12999, #31898, #11241, .T. ) ;
#19591=DIRECTION ( 'NONE',  ( 0.000000000000000000, 0.000000000000000000, 1.000000000000000000 ) ) ;
#19606=CARTESIAN_POINT ( 'NONE',  ( 27.00000000000000355, 198.9875000012290229, -3.306546357697854128E-15 ) ) ;
#19613=DIRECTION ( 'NONE',  ( 0.000000000000000000, 0.000000000000000000, 1.000000000000000000 ) ) ;
#19614=DIRECTION ( 'NONE',  ( 0.000000000000000000, 0.000000000000000000, 1.000000000000000000 ) ) ;
#19617=CARTESIAN_POINT ( 'NONE',  ( 26.75643035624999655, 247.3468750006145171, 3.323476615752267715 ) ) ;
#19619=CARTESIAN_POINT ( 'NONE',  ( 23.87821517812500005, 241.4593750006145285, 4.985214923628404016 ) ) ;
#19623=CARTESIAN_POINT ( 'NONE',  ( -13.50000000000000533, 199.9250000000000114, -23.38268590217984411 ) ) ;
#19625=EDGE_CURVE ( 'NONE', #21259, #32891, #2072, .T. ) ;
#19638=CARTESIAN_POINT ( 'NONE',  ( 15.24356964374999990, 247.9093750006145171, -3.323476615752268604 ) ) ;
#19639=EDGE_CURVE ( 'NONE', #19072, #15380, #34500, .T. ) ;
#19643=CARTESIAN_POINT ( 'NONE',  ( 5.128366027876307243, 215.9518627395465273, 0.7835069059936695668 ) ) ;
#19645=DIRECTION ( 'NONE',  ( 1.000000000000000000, 0.000000000000000000, 0.000000000000000000 ) ) ;
#19651=CARTESIAN_POINT ( 'NONE',  ( 5.778771075727756162E-15, 197.2156250006145513, 31.45816453501075927 ) ) ;
#19654=ORIENTED_EDGE ( 'NONE', *, *, #33451, .F. ) ;
#19655=CARTESIAN_POINT ( 'NONE',  ( 26.99999999999999645, 242.2187500012290684, -3.464101615137755275 ) ) ;
#19667=CARTESIAN_POINT ( 'NONE',  ( 18.00000000000000355, 249.1750000000000114, 5.196152422706632912 ) ) ;
#19669=CARTESIAN_POINT ( 'NONE',  ( -1.909035429704832693E-15, 197.1875000000000284, -31.17691453623979214 ) ) ;
#19673=CARTESIAN_POINT ( 'NONE',  ( 26.75643035624999655, 249.5968750006145171, 3.323476615752267271 ) ) ;
#19674=VERTEX_POINT ( 'NONE', #11797 ) ;
#19680=CARTESIAN_POINT ( 'NONE',  ( 15.00000000000000000, 244.1500000000000057, 0.000000000000000000 ) ) ;
#19681=CARTESIAN_POINT ( 'NONE',  ( -14.50000000000000000, 215.7563705986615901, 5.555555555555558023 ) ) ;
#19685=B_SPLINE_CURVE_WITH_KNOTS ( 'NONE', 3,
 ( #21551, #17953, #29684, #35178, #15100, #9414, #6378, #27403 ),
 .UNSPECIFIED., .F., .F.,
 ( 4, 2, 2, 4 ),
 ( 0.000000000000000000, 0.002521202642312846305, 0.003781803963469229125, 0.005042405284625611946 ),
 .UNSPECIFIED. ) ;
#19686=CARTESIAN_POINT ( 'NONE',  ( -13.49999999999998401, 194.7875000012290343, 23.38268590217985476 ) ) ;
#19690=CARTESIAN_POINT ( 'NONE',  ( 23.87821517812500005, 242.3593750006145342, 4.985214923628404016 ) ) ;
#19697=CARTESIAN_POINT ( 'NONE',  ( 27.24356964375000700, 197.7968750006145342, 15.72908226750537075 ) ) ;
#19702=DIRECTION ( 'NONE',  ( -1.000000000000000000, -0.000000000000000000, -0.000000000000000000 ) ) ;
#19714=CARTESIAN_POINT ( 'NONE',  ( 23.99999999999999645, 240.4562500012290513, -5.196152422706631135 ) ) ;
#19718=CARTESIAN_POINT ( 'NONE',  ( 13.62178482187501416, 195.9593750006145569, 23.59362340125806767 ) ) ;
#19722=CARTESIAN_POINT ( 'NONE',  ( 23.87821517812499650, 241.6093750006145342, -4.985214923628404904 ) ) ;
#19723=DIRECTION ( 'NONE',  ( -0.000000000000000000, -1.000000000000000000, -0.000000000000000000 ) ) ;
#19725=( BOUNDED_CURVE ( )  B_SPLINE_CURVE ( 2, ( #18148, #18334, #15486, #17960, #27040, #1066, #12637, #27227, #20805 ),
 .UNSPECIFIED., .F., .F. ) 
 B_SPLINE_CURVE_WITH_KNOTS ( ( 3, 2, 2, 2, 3 ),
 ( 0.2717391304347825942, 0.2753623188405797118, 0.2826086956521738913, 0.2898550724637681264, 0.2934782608695652439 ),
 .UNSPECIFIED. ) 
 CURVE ( )  GEOMETRIC_REPRESENTATION_ITEM ( )  RATIONAL_B_SPLINE_CURVE ( ( 0.9330127018922191873, 0.9330127018922187432, 1.000000000000000000, 0.8660254037844387076, 1.000000000000000000, 0.8660254037844387076, 1.000000000000000000, 0.9330127018922188542, 0.9330127018922194093 ) ) 
 REPRESENTATION_ITEM ( '' )  );
#19728=B_SPLINE_CURVE_WITH_KNOTS ( 'NONE', 3,
 ( #13988, #25357, #4887, #2229 ),
 .UNSPECIFIED., .F., .F.,
 ( 4, 4 ),
 ( 0.000000000000000000, 1.000000000000000000 ),
 .UNSPECIFIED. ) ;
#19731=CARTESIAN_POINT ( 'NONE',  ( 26.75643035624999655, 243.7093750006145285, -3.323476615752271712 ) ) ;
#19742=CARTESIAN_POINT ( 'NONE',  ( 15.24356964374999990, 243.8593750006145342, -3.323476615752268604 ) ) ;
#19750=CARTESIAN_POINT ( 'NONE',  ( -26.99999999999999645, 199.5875000000000341, 15.58845726811991561 ) ) ;
#19762=FACE_OUTER_BOUND ( 'NONE', #11863, .T. ) ;
#19763=CARTESIAN_POINT ( 'NONE',  ( -13.62178482187500528, 196.1843750006145228, -23.59362340125807123 ) ) ;
#19770=CARTESIAN_POINT ( 'NONE',  ( 26.99999999999999645, 241.7312500012290570, -7.347880794884117764E-16 ) ) ;
#19778=CARTESIAN_POINT ( 'NONE',  ( 18.00000000000000355, 246.0812500012290513, 5.196152422706632912 ) ) ;
#19786=ORIENTED_EDGE ( 'NONE', *, *, #37261, .T. ) ;
#19801=CARTESIAN_POINT ( 'NONE',  ( 0.000000000000000000, 210.0000000000000284, 0.000000000000000000 ) ) ;
#19805=CARTESIAN_POINT ( 'NONE',  ( 15.24356964374999990, 247.5718750006145399, -3.323476615752268604 ) ) ;
#19807=CARTESIAN_POINT ( 'NONE',  ( 18.12178482187500350, 242.7343750006145342, 4.985214923628407568 ) ) ;
#19812=CARTESIAN_POINT ( 'NONE',  ( 23.99999999999999645, 249.4562500012290229, -5.196152422706631135 ) ) ;
#19824=CARTESIAN_POINT ( 'NONE',  ( 23.87821517812500005, 248.5468750006145058, 4.985214923628404016 ) ) ;
#19827=CARTESIAN_POINT ( 'NONE',  ( 15.53186252112510779, 224.5816999436668766, -2.477503916096131409 ) ) ;
#19835=CARTESIAN_POINT ( 'NONE',  ( 20.99999999999999645, 243.3624999999999829, 5.999999999999998224 ) ) ;
#19851=CARTESIAN_POINT ( 'NONE',  ( -13.50000000000000533, 198.1250000000000284, -23.38268590217984411 ) ) ;
#19855=CARTESIAN_POINT ( 'NONE',  ( 20.99999999999999645, 248.6218750006145228, 6.646953231504538984 ) ) ;
#19856=ORIENTED_EDGE ( 'NONE', *, *, #23504, .T. ) ;
#19862=CARTESIAN_POINT ( 'NONE',  ( 18.00000000000000000, 243.6250000000000000, -5.196152422706630247 ) ) ;
#19867=CARTESIAN_POINT ( 'NONE',  ( 13.50000000000001421, 196.6625000012290343, 23.38268590217984055 ) ) ;
#19868=CARTESIAN_POINT ( 'NONE',  ( -7.234628195640302017, 196.6049038117967029, 27.00000000000000711 ) ) ;
#19871=CARTESIAN_POINT ( 'NONE',  ( 15.24356964374999990, 243.0718750006145115, -3.323476615752268604 ) ) ;
#19880=CARTESIAN_POINT ( 'NONE',  ( 25.01286569224582834, 195.0000000000000000, -10.34054035972909169 ) ) ;
#19881=CARTESIAN_POINT ( 'NONE',  ( 27.24356964375000345, 197.3843750006145399, -3.336375036156643733E-15 ) ) ;
#19894=DIRECTION ( 'NONE',  ( 4.130293990420971239E-17, -1.000000000000000000, 0.000000000000000000 ) ) ;
#19896=ORIENTED_EDGE ( 'NONE', *, *, #12423, .F. ) ;
#19900=CARTESIAN_POINT ( 'NONE',  ( -1.926257025242585782E-15, 195.6968750006145683, -31.45816453501076637 ) ) ;
#19903=PLANE ( 'NONE',  #8384 ) ;
#19904=CARTESIAN_POINT ( 'NONE',  ( 26.75643035624999655, 241.1218750006145228, -3.323476615752271712 ) ) ;
#19905=CARTESIAN_POINT ( 'NONE',  ( 5.778771075727756162E-15, 198.1156250006145285, 31.45816453501076637 ) ) ;
#19910=CARTESIAN_POINT ( 'NONE',  ( 26.75643035624999655, 241.9093750006145171, -3.323476615752271712 ) ) ;
#19916=AXIS2_PLACEMENT_3D ( 'NONE', #31790, #28946, #3168 ) ;
#19921=( BOUNDED_CURVE ( )  B_SPLINE_CURVE ( 2, ( #11352, #3182, #22923, #28771, #14758, #37116, #26301, #23471, #2439 ),
 .UNSPECIFIED., .F., .F. ) 
 B_SPLINE_CURVE_WITH_KNOTS ( ( 3, 2, 2, 2, 3 ),
 ( 0.6875000000000000000, 0.6944444444444444198, 0.7083333333333333703, 0.7222222222222222099, 0.7291666666666667407 ),
 .UNSPECIFIED. ) 
 CURVE ( )  GEOMETRIC_REPRESENTATION_ITEM ( )  RATIONAL_B_SPLINE_CURVE ( ( 0.9330127018922194093, 0.9330127018922194093, 1.000000000000000000, 0.8660254037844387076, 1.000000000000000000, 0.8660254037844387076, 1.000000000000000000, 0.9330127018922187432, 0.9330127018922192983 ) ) 
 REPRESENTATION_ITEM ( '' )  );
#19923=CARTESIAN_POINT ( 'NONE',  ( 18.12178482187500350, 245.3218750006145115, 4.985214923628407568 ) ) ;
#19929=CYLINDRICAL_SURFACE ( 'NONE', #4012, 27.00000000000000000 ) ;
#19930=CARTESIAN_POINT ( 'NONE',  ( 19.39230484541324273, 241.1486538117967200, 5.999999999999987566 ) ) ;
#19937=ORIENTED_EDGE ( 'NONE', *, *, #22077, .T. ) ;
#19942=CARTESIAN_POINT ( 'NONE',  ( 15.00000000000000000, 242.4062500012290400, 0.000000000000000000 ) ) ;
#19943=CARTESIAN_POINT ( 'NONE',  ( 27.24356964374999635, 195.6218750006145228, -15.72908226750539029 ) ) ;
#19944=CARTESIAN_POINT ( 'NONE',  ( 5.903039156993664882, 194.9999999999999716, 26.61078777808395657 ) ) ;
#19949=CARTESIAN_POINT ( 'NONE',  ( 21.00000000000000000, 248.9593750006145285, 6.646953231504538984 ) ) ;
#19960=CARTESIAN_POINT ( 'NONE',  ( -25.28513278367194772, 195.0000000000000284, -9.605453057530283445 ) ) ;
#19965=CARTESIAN_POINT ( 'NONE',  ( -28.98530087525818999, 202.0528329772414224, 1.056834216689858774 ) ) ;
#19966=CARTESIAN_POINT ( 'NONE',  ( 4.999999999999998224, 216.0000000000000000, -3.514718625761428239 ) ) ;
#19972=ORIENTED_EDGE ( 'NONE', *, *, #30346, .F. ) ;
#19980=CARTESIAN_POINT ( 'NONE',  ( 21.00000000000000000, 246.1187500012290457, 5.999999999999998224 ) ) ;
#19981=CARTESIAN_POINT ( 'NONE',  ( 23.87821517812500005, 244.1593750006145171, 4.985214923628404016 ) ) ;
#19983=CARTESIAN_POINT ( 'NONE',  ( 23.87821517812499650, 241.6093750006145342, -4.985214923628404904 ) ) ;
#19986=CARTESIAN_POINT ( 'NONE',  ( 26.99999999999999645, 248.5187500012290798, -3.464101615137755275 ) ) ;
#19987=ORIENTED_EDGE ( 'NONE', *, *, #23373, .T. ) ;
#19996=VERTEX_POINT ( 'NONE', #4208 ) ;
#20003=CARTESIAN_POINT ( 'NONE',  ( 5.205286459874319149, 215.9230175775472276, 0.9779651927393356869 ) ) ;
#20015=CARTESIAN_POINT ( 'NONE',  ( 22.60769515458672885, 242.2736538117966916, -5.999999999999998224 ) ) ;
#20018=CARTESIAN_POINT ( 'NONE',  ( 20.99999999999995026, 243.1375000000000455, -5.999999999999998224 ) ) ;
#20026=CARTESIAN_POINT ( 'NONE',  ( 19.39230484541326760, 243.3986538117966916, 5.999999999999999112 ) ) ;
#20028=CARTESIAN_POINT ( 'NONE',  ( 13.49999999999999645, 198.0500000000000114, -23.38268590217984766 ) ) ;
#20031=CARTESIAN_POINT ( 'NONE',  ( 23.87821517812500005, 248.2093750006145285, 4.985214923628404016 ) ) ;
#20038=CARTESIAN_POINT ( 'NONE',  ( 15.00000000000000178, 244.1875000000000000, 3.464101615137757051 ) ) ;
#20039=CARTESIAN_POINT ( 'NONE',  ( -27.00000000000000355, 198.6125000000000114, -15.58845726811989429 ) ) ;
#20041=( BOUNDED_CURVE ( )  B_SPLINE_CURVE ( 2, ( #23814, #15472, #488, #35550, #6748, #9032, #32333, #30056, #3711 ),
 .UNSPECIFIED., .F., .F. ) 
 B_SPLINE_CURVE_WITH_KNOTS ( ( 3, 2, 2, 2, 3 ),
 ( 0.6630434782608695121, 0.6666666666666666297, 0.6739130434782608647, 0.6811594202898550998, 0.6847826086956522174 ),
 .UNSPECIFIED. ) 
 CURVE ( )  GEOMETRIC_REPRESENTATION_ITEM ( )  RATIONAL_B_SPLINE_CURVE ( ( 0.9330127018922192983, 0.9330127018922182991, 1.000000000000000000, 0.8660254037844387076, 1.000000000000000000, 0.8660254037844387076, 1.000000000000000000, 0.9330127018922182991, 0.9330127018922192983 ) ) 
 REPRESENTATION_ITEM ( '' )  );
#20043=EDGE_LOOP ( 'NONE', ( #13889, #18489, #18319, #28300 ) ) ;
#20046=CARTESIAN_POINT ( 'NONE',  ( 26.99999999999999645, 196.3250000012290570, -15.58845726811990495 ) ) ;
#20049=CARTESIAN_POINT ( 'NONE',  ( 21.00000000000000000, 242.7718750006145854, 6.646953231504538984 ) ) ;
#20052=ADVANCED_FACE ( 'NONE', ( #15593 ), #4021, .F. ) ;
#20058=CARTESIAN_POINT ( 'NONE',  ( 25.58178997548098366, 194.9999999999998863, 9.109611009433765005 ) ) ;
#20059=CARTESIAN_POINT ( 'NONE',  ( -1.926257025242585782E-15, 195.2468750006145513, -31.45816453501075927 ) ) ;
#20072=CARTESIAN_POINT ( 'NONE',  ( 26.99999999999999645, 248.8374999999999773, 3.464101615137751278 ) ) ;
#20073=CARTESIAN_POINT ( 'NONE',  ( 26.99999999999999645, 240.3812500012290343, -7.347880794884117764E-16 ) ) ;
#20077=CARTESIAN_POINT ( 'NONE',  ( 27.24356964374999279, 196.0718750006145399, -15.72908226750539207 ) ) ;
#20082=CARTESIAN_POINT ( 'NONE',  ( 21.00000000000000000, 240.7468750006145228, -6.646953231504538984 ) ) ;
#20083=CARTESIAN_POINT ( 'NONE',  ( 27.24356964375000345, 199.1281250006145171, -3.336375036156643733E-15 ) ) ;
#20088=CARTESIAN_POINT ( 'NONE',  ( -13.62178482187498396, 198.0781250006145342, 23.59362340125808188 ) ) ;
#20089=CARTESIAN_POINT ( 'NONE',  ( 26.75643035624999655, 241.4593750006145285, -3.323476615752271712 ) ) ;
#20090=LINE ( 'NONE', #6746, #2576 ) ;
#20097=CARTESIAN_POINT ( 'NONE',  ( 20.99999999999999645, 241.3093750006145228, 6.646953231504538984 ) ) ;
#20107=CARTESIAN_POINT ( 'NONE',  ( -20.80563922340697403, 195.0000000000000284, -17.20829382900668492 ) ) ;
#20108=CARTESIAN_POINT ( 'NONE',  ( 18.00000000000000000, 241.4312500012290457, -5.196152422706630247 ) ) ;
#20112=DIRECTION ( 'NONE',  ( 0.000000000000000000, -1.000000000000000000, 0.000000000000000000 ) ) ;
#20116=CARTESIAN_POINT ( 'NONE',  ( 22.60769515458672885, 241.1325961894323484, 5.999999999999997335 ) ) ;
#20117=CARTESIAN_POINT ( 'NONE',  ( 20.99999999999999645, 185.0294372515228645, 0.000000000000000000 ) ) ;
#20118=CARTESIAN_POINT ( 'NONE',  ( -27.24356964375000345, 194.8857344423842619, -9.915847606754343957 ) ) ;
#20119=DIRECTION ( 'NONE',  ( 1.000000000000000000, 0.000000000000000000, 0.000000000000000000 ) ) ;
#20120=CARTESIAN_POINT ( 'NONE',  ( 1.120210788295102201E-13, 196.8500000012290343, -27.00000000000000711 ) ) ;
#20126=CARTESIAN_POINT ( 'NONE',  ( 26.75643035624999655, 248.5843750006145001, 3.323476615752267715 ) ) ;
#20132=ORIENTED_EDGE ( 'NONE', *, *, #14224, .F. ) ;
#20141=CIRCLE ( 'NONE', #9860, 27.00000000000000000 ) ;
#20145=CARTESIAN_POINT ( 'NONE',  ( 20.99999999999999645, 185.0294372515228645, 5.999999999999999112 ) ) ;
#20162=CARTESIAN_POINT ( 'NONE',  ( 26.75643035624999655, 246.4843750006145342, -7.049594010296217766E-16 ) ) ;
#20164=CARTESIAN_POINT ( 'NONE',  ( 20.99999999999999645, 240.7468750006145228, -6.646953231504538984 ) ) ;
#20168=CARTESIAN_POINT ( 'NONE',  ( 18.00000000000000355, 245.1812500012290457, 5.196152422706632912 ) ) ;
#20172=CARTESIAN_POINT ( 'NONE',  ( 15.00000000000000000, 246.8125000000000000, -3.464101615137752610 ) ) ;
#20177=ORIENTED_EDGE ( 'NONE', *, *, #17571, .F. ) ;
#20181=CARTESIAN_POINT ( 'NONE',  ( 19.39230484541326049, 241.8638461906614054, -5.999999999999997335 ) ) ;
#20182=CARTESIAN_POINT ( 'NONE',  ( 23.87821517812499650, 246.4468750006145115, -4.985214923628404904 ) ) ;
#20185=CARTESIAN_POINT ( 'NONE',  ( 15.81961138684103929, 215.1803886131357615, -3.965927053044179917 ) ) ;
#20196=VERTEX_POINT ( 'NONE', #5326 ) ;
#20201=VECTOR ( 'NONE', #15218, 1000.000000000000000 ) ;
#20209=CARTESIAN_POINT ( 'NONE',  ( -27.00000000000000355, 196.4000000000000057, 0.000000000000000000 ) ) ;
#20212=CARTESIAN_POINT ( 'NONE',  ( 18.12178482187500350, 249.0343750006145456, 4.985214923628407568 ) ) ;
#20217=CARTESIAN_POINT ( 'NONE',  ( 26.99999999999999645, 243.5124999999999602, -3.464101615137755275 ) ) ;
#20221=CARTESIAN_POINT ( 'NONE',  ( 24.00000000000000000, 241.6000000000000227, 5.196152422706629359 ) ) ;
#20225=ORIENTED_EDGE ( 'NONE', *, *, #11409, .T. ) ;
#20228=CARTESIAN_POINT ( 'NONE',  ( 13.50000000000001421, 195.3125000012290400, 23.38268590217984055 ) ) ;
#20233=CARTESIAN_POINT ( 'NONE',  ( 15.24356964374999990, 240.8218750006145399, -3.323476615752268604 ) ) ;
#20238=CARTESIAN_POINT ( 'NONE',  ( 20.99999999999999289, 249.8874999999999886, -5.999999999999997335 ) ) ;
#20240=ADVANCED_FACE ( 'NONE', ( #19009 ), #2110, .F. ) ;
#20242=CARTESIAN_POINT ( 'NONE',  ( 14.42938872624734259, 195.0000000000000000, 23.12445431839006105 ) ) ;
#20243=CARTESIAN_POINT ( 'NONE',  ( -13.62178482187498396, 194.9843750006145626, 23.59362340125808188 ) ) ;
#20247=ORIENTED_EDGE ( 'NONE', *, *, #15002, .T. ) ;
#20249=CARTESIAN_POINT ( 'NONE',  ( 19.39230484541326049, 240.4575961894323370, -5.999999999999997335 ) ) ;
#20262=CARTESIAN_POINT ( 'NONE',  ( -7.234628195640354420, 195.1424038105676573, 26.99999999999996803 ) ) ;
#20266=CARTESIAN_POINT ( 'NONE',  ( 27.24356964375000345, 196.4843750006145626, -3.336375036156643733E-15 ) ) ;
#20270=CARTESIAN_POINT ( 'NONE',  ( 18.00000000000000000, 247.2249999999999943, -5.196152422706630247 ) ) ;
#20271=CARTESIAN_POINT ( 'NONE',  ( -1.926257025242585782E-15, 197.8906250006145342, -31.45816453501076637 ) ) ;
#20275=ORIENTED_EDGE ( 'NONE', *, *, #25685, .T. ) ;
#20276=ORIENTED_EDGE ( 'NONE', *, *, #14224, .T. ) ;
#20277=CARTESIAN_POINT ( 'NONE',  ( -1.926257025242585782E-15, 197.4406250006145740, -31.45816453501075927 ) ) ;
#20278=CARTESIAN_POINT ( 'NONE',  ( 18.12178482187499640, 242.0218750006145001, -4.985214923628404904 ) ) ;
#20282=CARTESIAN_POINT ( 'NONE',  ( 15.24356964375000167, 247.6468750006145569, 3.323476615752272600 ) ) ;
#20286=CARTESIAN_POINT ( 'NONE',  ( 15.24356964375000167, 243.0343750006144887, 3.323476615752272600 ) ) ;
#20293=CARTESIAN_POINT ( 'NONE',  ( 22.60769515458672885, 240.0236538117966916, -5.999999999999998224 ) ) ;
#20294=CARTESIAN_POINT ( 'NONE',  ( -26.99999999999999645, 198.8000000012290513, 15.58845726811991561 ) ) ;
#20298=EDGE_CURVE ( 'NONE', #37055, #529, #618, .T. ) ;
#20302=CARTESIAN_POINT ( 'NONE',  ( 23.87821517812499650, 242.8468750006145171, -4.985214923628404904 ) ) ;
#20309=CARTESIAN_POINT ( 'NONE',  ( 15.00000000000000000, 246.8687500012290457, -3.464101615137752610 ) ) ;
#20311=CARTESIAN_POINT ( 'NONE',  ( 22.60769515458672529, 246.2674038105676004, -6.000000000000004441 ) ) ;
#20317=CARTESIAN_POINT ( 'NONE',  ( 24.00000000000000000, 239.8562500012290286, 5.196152422706629359 ) ) ;
#20326=CARTESIAN_POINT ( 'NONE',  ( 15.00000000000000000, 245.9687500012290684, -3.464101615137752610 ) ) ;
#20329=CARTESIAN_POINT ( 'NONE',  ( 18.12178482187500350, 248.0218750006145001, 4.985214923628407568 ) ) ;
#20331=CARTESIAN_POINT ( 'NONE',  ( -20.80563922340697403, 195.0000000000000284, -17.20829382900668492 ) ) ;
#20336=ORIENTED_EDGE ( 'NONE', *, *, #26308, .F. ) ;
#20337=CARTESIAN_POINT ( 'NONE',  ( -7.234628195640302017, 197.9549038117966973, 27.00000000000000711 ) ) ;
#20349=CARTESIAN_POINT ( 'NONE',  ( 21.00000000000001066, 247.4124999999999943, 5.999999999999998224 ) ) ;
#20353=CARTESIAN_POINT ( 'NONE',  ( 23.87821517812499650, 245.2093750006145569, -4.985214923628404904 ) ) ;
#20355=CARTESIAN_POINT ( 'NONE',  ( 20.00041297495057435, 239.8598985277378972, -5.668978411116884608 ) ) ;
#20356=ORIENTED_EDGE ( 'NONE', *, *, #37261, .F. ) ;
#20359=CARTESIAN_POINT ( 'NONE',  ( 26.99999999999999645, 245.8187500012290627, -3.464101615137755275 ) ) ;
#20368=ORIENTED_EDGE ( 'NONE', *, *, #30812, .F. ) ;
#20369=VERTEX_POINT ( 'NONE', #28451 ) ;
#20371=CARTESIAN_POINT ( 'NONE',  ( 26.75643035624999655, 245.8843750006145399, 3.323476615752267715 ) ) ;
#20374=ADVANCED_FACE ( 'NONE', ( #4956 ), #4777, .F. ) ;
#20389=CARTESIAN_POINT ( 'NONE',  ( 24.00000000000000000, 240.6999999999999886, 5.196152422706629359 ) ) ;
#20392=CARTESIAN_POINT ( 'NONE',  ( 18.00000000000000000, 243.1750000000000114, -5.196152422706630247 ) ) ;
#20397=CARTESIAN_POINT ( 'NONE',  ( 0.000000000000000000, 210.0000000000000284, -27.00000000000000000 ) ) ;
#20401=CARTESIAN_POINT ( 'NONE',  ( 27.00000000000000355, 196.1750000000000114, -3.306546357697854128E-15 ) ) ;
#20404=CARTESIAN_POINT ( 'NONE',  ( 26.75643035624999655, 247.3843750006145399, -7.049594010296217766E-16 ) ) ;
#20407=CARTESIAN_POINT ( 'NONE',  ( -29.00000000000002487, 216.0000000000000000, 7.347880794884114806E-16 ) ) ;
#20411=CARTESIAN_POINT ( 'NONE',  ( 26.99999999999999645, 241.1875000000000284, 3.464101615137751278 ) ) ;
#20414=VERTEX_POINT ( 'NONE', #14990 ) ;
#20417=CARTESIAN_POINT ( 'NONE',  ( 27.00000000000001066, 195.8000000012290513, 15.58845726811988897 ) ) ;
#20423=CARTESIAN_POINT ( 'NONE',  ( 15.24356964375000167, 240.4468750006145399, 3.323476615752272600 ) ) ;
#20426=CARTESIAN_POINT ( 'NONE',  ( -20.68320042480035426, 195.0000000000000000, -17.35526491262920956 ) ) ;
#20433=CARTESIAN_POINT ( 'NONE',  ( 25.75952191513118095, 195.0000000000000000, 8.586198610466265535 ) ) ;
#20434=CARTESIAN_POINT ( 'NONE',  ( 27.24356964375000345, 196.9343750006145228, -3.336375036156643733E-15 ) ) ;
#20436=ORIENTED_EDGE ( 'NONE', *, *, #18646, .T. ) ;
#20446=CARTESIAN_POINT ( 'NONE',  ( 20.99999999999999645, 185.0294372515228645, 0.000000000000000000 ) ) ;
#20450=CARTESIAN_POINT ( 'NONE',  ( -13.49999999999998401, 195.1250000000000284, 23.38268590217985476 ) ) ;
#20454=CARTESIAN_POINT ( 'NONE',  ( 13.62178482187499640, 196.5593750006145513, -23.59362340125807123 ) ) ;
#20458=CARTESIAN_POINT ( 'NONE',  ( 26.99999999999999645, 249.3625000000000114, -3.464101615137755275 ) ) ;
#20459=CARTESIAN_POINT ( 'NONE',  ( -13.62178482187498396, 197.6281250006145171, 23.59362340125808188 ) ) ;
#20465=CARTESIAN_POINT ( 'NONE',  ( 13.62178482187499640, 198.7531250006145456, -23.59362340125807123 ) ) ;
#20466=CARTESIAN_POINT ( 'NONE',  ( 15.24356964375000167, 242.5843750006145285, 3.323476615752272600 ) ) ;
#20468=( BOUNDED_CURVE ( )  B_SPLINE_CURVE ( 2, ( #13409, #24958, #36145, #30844, #4868, #2023, #21764, #13601, #36706 ),
 .UNSPECIFIED., .F., .F. ) 
 B_SPLINE_CURVE_WITH_KNOTS ( ( 3, 2, 2, 2, 3 ),
 ( 0.1875000000000000000, 0.1944444444444444475, 0.2083333333333333426, 0.2222222222222222099, 0.2291666666666666574 ),
 .UNSPECIFIED. ) 
 CURVE ( )  GEOMETRIC_REPRESENTATION_ITEM ( )  RATIONAL_B_SPLINE_CURVE ( ( 0.9330127018922194093, 0.9330127018922194093, 1.000000000000000000, 0.8660254037844387076, 1.000000000000000000, 0.8660254037844387076, 1.000000000000000000, 0.9330127018922194093, 0.9330127018922194093 ) ) 
 REPRESENTATION_ITEM ( '' )  );
#20470=CARTESIAN_POINT ( 'NONE',  ( 26.75643035624999655, 246.4843750006145342, -7.049594010296217766E-16 ) ) ;
#20474=CARTESIAN_POINT ( 'NONE',  ( 20.99999999999999645, 242.8843750006145399, -6.646953231504538984 ) ) ;
#20486=CARTESIAN_POINT ( 'NONE',  ( 20.99999999999999289, 241.3937500012289945, -5.999999999999997335 ) ) ;
#20490=CARTESIAN_POINT ( 'NONE',  ( 15.24356964374999990, 241.6093750006145058, -3.323476615752268604 ) ) ;
#20497=CARTESIAN_POINT ( 'NONE',  ( 20.99999999999995381, 241.1687500012290570, 5.999999999999998224 ) ) ;
#20506=CARTESIAN_POINT ( 'NONE',  ( 15.24356964374999990, 249.2593750006145115, -3.323476615752268604 ) ) ;
#20512=ORIENTED_EDGE ( 'NONE', *, *, #322, .T. ) ;
#20514=EDGE_LOOP ( 'NONE', ( #18153, #23671, #12191, #33188 ) ) ;
#20518=CARTESIAN_POINT ( 'NONE',  ( 15.24356964374999990, 248.8093750006144944, -3.323476615752268604 ) ) ;
#20524=ORIENTED_EDGE ( 'NONE', *, *, #31868, .T. ) ;
#20535=CARTESIAN_POINT ( 'NONE',  ( 5.649999999999987921, 244.5000000000000000, -2.499999999999999556 ) ) ;
#20537=CARTESIAN_POINT ( 'NONE',  ( 26.99999999999999645, 197.5625000000000000, -15.58845726811990495 ) ) ;
#20539=CARTESIAN_POINT ( 'NONE',  ( 26.75643035624999655, 246.0343750006145456, -7.049594010296217766E-16 ) ) ;
#20541=CARTESIAN_POINT ( 'NONE',  ( 15.24356964375000167, 239.9968750006145228, 3.323476615752272600 ) ) ;
#20544=CARTESIAN_POINT ( 'NONE',  ( 15.00000000000000178, 246.0437500012290570, 3.464101615137757051 ) ) ;
#20552=EDGE_LOOP ( 'NONE', ( #24496, #11253, #20524, #34352 ) ) ;
#20556=CARTESIAN_POINT ( 'NONE',  ( 18.12178482187500350, 246.6718750006145342, 4.985214923628407568 ) ) ;
#20570=ORIENTED_EDGE ( 'NONE', *, *, #18215, .T. ) ;
#20583=CARTESIAN_POINT ( 'NONE',  ( -13.49999999999998401, 195.1250000000000284, 23.38268590217985476 ) ) ;
#20586=CARTESIAN_POINT ( 'NONE',  ( 18.12178482187499640, 246.1843750006145228, -4.985214923628404904 ) ) ;
#20590=CARTESIAN_POINT ( 'NONE',  ( 22.60769515458672885, 243.3825961894323484, 5.999999999999997335 ) ) ;
#20592=CYLINDRICAL_SURFACE ( 'NONE', #5593, 5.999999999999999112 ) ;
#20595=CARTESIAN_POINT ( 'NONE',  ( 18.00000000000000355, 241.9749999999999943, 5.196152422706632912 ) ) ;
#20600=VERTEX_POINT ( 'NONE', #29939 ) ;
#20602=CARTESIAN_POINT ( 'NONE',  ( 26.99999999999999645, 246.6250000000000000, -7.347880794884117764E-16 ) ) ;
#20603=CARTESIAN_POINT ( 'NONE',  ( 1.120210788295102201E-13, 195.3875000000000455, -27.00000000000000711 ) ) ;
#20605=CIRCLE ( 'NONE', #24226, 27.00000000000000000 ) ;
#20609=CARTESIAN_POINT ( 'NONE',  ( 26.75643035624999655, 241.1218750006145228, -3.323476615752271712 ) ) ;
#20611=CARTESIAN_POINT ( 'NONE',  ( 2.999999999999997335, 244.5000000000000000, 5.000000000000000000 ) ) ;
#20617=CARTESIAN_POINT ( 'NONE',  ( 19.61859908393741492, 194.9999999999999432, 18.97589165950046208 ) ) ;
#20618=CARTESIAN_POINT ( 'NONE',  ( -13.62178482187500528, 196.1843750006145228, -23.59362340125807123 ) ) ;
#20621=EDGE_LOOP ( 'NONE', ( #33295, #9854, #7485, #11218 ) ) ;
#20623=CYLINDRICAL_SURFACE ( 'NONE', #14723, 9.999999999999998224 ) ;
#20624=CARTESIAN_POINT ( 'NONE',  ( 26.99999999999999645, 198.9125000000000512, -15.58845726811990495 ) ) ;
#20631=DIRECTION ( 'NONE',  ( -0.000000000000000000, -1.000000000000000000, -0.000000000000000000 ) ) ;
#20632=CARTESIAN_POINT ( 'NONE',  ( 24.00000000000000000, 245.6500000000000057, 5.196152422706629359 ) ) ;
#20641=DIRECTION ( 'NONE',  ( -0.000000000000000000, -1.000000000000000000, -0.000000000000000000 ) ) ;
#20642=CARTESIAN_POINT ( 'NONE',  ( 26.99999999999999645, 249.2874999999999943, 3.464101615137751278 ) ) ;
#20643=CARTESIAN_POINT ( 'NONE',  ( -27.24356964375000345, 199.3531250006145399, 0.000000000000000000 ) ) ;
#20646=VECTOR ( 'NONE', #3708, 1000.000000000000000 ) ;
#20649=CARTESIAN_POINT ( 'NONE',  ( 27.24356964374999635, 195.1156250006145001, -15.72908226750539029 ) ) ;
#20650=CARTESIAN_POINT ( 'NONE',  ( 18.12178482187500350, 243.0718750006145399, 4.985214923628407568 ) ) ;
#20653=CARTESIAN_POINT ( 'NONE',  ( 15.24356964374999990, 248.5093750006145399, 0.000000000000000000 ) ) ;
#20658=CARTESIAN_POINT ( 'NONE',  ( 23.87821517812499650, 241.4968750006144944, -4.985214923628404904 ) ) ;
#20673=CARTESIAN_POINT ( 'NONE',  ( 15.24356964374999990, 242.9593750006145001, -3.323476615752268604 ) ) ;
#20681=CARTESIAN_POINT ( 'NONE',  ( 20.99999999999999645, 245.2187500012290116, 5.999999999999998224 ) ) ;
#20682=CARTESIAN_POINT ( 'NONE',  ( 2.867614517141320096, 194.9999999999999432, 27.09578238708614961 ) ) ;
#20687=CARTESIAN_POINT ( 'NONE',  ( 23.87821517812499650, 249.5968750006145171, -4.985214923628404904 ) ) ;
#20692=CARTESIAN_POINT ( 'NONE',  ( 24.00000000000000000, 247.9000000000000057, 5.196152422706629359 ) ) ;
#20698=( BOUNDED_CURVE ( )  B_SPLINE_CURVE ( 3, ( #9577, #9391, #30230, #20965 ),
 .UNSPECIFIED., .F., .F. ) 
 B_SPLINE_CURVE_WITH_KNOTS ( ( 4, 4 ),
 ( 4.712388980384689674, 7.853981633974482790 ),
 .UNSPECIFIED. ) 
 CURVE ( )  GEOMETRIC_REPRESENTATION_ITEM ( )  RATIONAL_B_SPLINE_CURVE ( ( 1.000000000000000000, 0.3333333333333333703, 0.3333333333333333703, 1.000000000000000000 ) ) 
 REPRESENTATION_ITEM ( '' )  );
#20700=CARTESIAN_POINT ( 'NONE',  ( 26.75643035624999655, 249.5593750006144944, -3.323476615752271268 ) ) ;
#20704=EDGE_CURVE ( 'NONE', #9483, #12534, #9828, .T. ) ;
#20706=ORIENTED_EDGE ( 'NONE', *, *, #30955, .F. ) ;
#20707=CARTESIAN_POINT ( 'NONE',  ( 22.60769515458672885, 248.1236538117966859, -6.000000000000000000 ) ) ;
#20714=ORIENTED_EDGE ( 'NONE', *, *, #16331, .F. ) ;
#20723=CARTESIAN_POINT ( 'NONE',  ( 26.75643035624999655, 245.1343750006145115, -7.049594010296217766E-16 ) ) ;
#20726=ORIENTED_EDGE ( 'NONE', *, *, #33945, .T. ) ;
#20729=CARTESIAN_POINT ( 'NONE',  ( 24.00000000000000000, 246.6062500012290570, 5.196152422706629359 ) ) ;
#20737=VERTEX_POINT ( 'NONE', #369 ) ;
#20742=CARTESIAN_POINT ( 'NONE',  ( 15.24356964375000167, 247.5343750006144887, 3.323476615752272600 ) ) ;
#20773=CARTESIAN_POINT ( 'NONE',  ( 26.75643035624999655, 246.9343750006145228, -7.049594010296217766E-16 ) ) ;
#20777=DIRECTION ( 'NONE',  ( 0.000000000000000000, 0.000000000000000000, 1.000000000000000000 ) ) ;
#20782=CARTESIAN_POINT ( 'NONE',  ( 26.99999999999999645, 241.7125000000000057, -3.464101615137755275 ) ) ;
#20783=CARTESIAN_POINT ( 'NONE',  ( -10.38977131807862975, 218.0044321092237283, 3.786121002044094741 ) ) ;
#20786=ORIENTED_EDGE ( 'NONE', *, *, #21200, .T. ) ;
#20795=CARTESIAN_POINT ( 'NONE',  ( 23.87821517812499650, 240.2593750006145399, -4.985214923628404904 ) ) ;
#20797=B_SPLINE_CURVE_WITH_KNOTS ( 'NONE', 3,
 ( #27110, #24456, #35817, #12891 ),
 .UNSPECIFIED., .F., .F.,
 ( 4, 4 ),
 ( 0.000000000000000000, 1.000000000000000000 ),
 .UNSPECIFIED. ) ;
#20803=AXIS2_PLACEMENT_3D ( 'NONE', #20117, #31850, #2483 ) ;
#20805=CARTESIAN_POINT ( 'NONE',  ( 20.99999999999997868, 246.9625000000000057, 5.999999999999999112 ) ) ;
#20806=CARTESIAN_POINT ( 'NONE',  ( 13.62178482187501416, 196.4093750006145456, 23.59362340125806767 ) ) ;
#20810=ORIENTED_EDGE ( 'NONE', *, *, #24434, .F. ) ;
#20812=DIRECTION ( 'NONE',  ( -0.000000000000000000, -1.000000000000000000, -0.000000000000000000 ) ) ;
#20820=CARTESIAN_POINT ( 'NONE',  ( 22.60769515458672885, 245.6325961894323768, 5.999999999999997335 ) ) ;
#20823=CARTESIAN_POINT ( 'NONE',  ( 1.069080835302379631E-14, 199.3250000012290286, 27.00000000000000000 ) ) ;
#20824=CARTESIAN_POINT ( 'NONE',  ( 20.99999999999999645, 185.0294372515228645, 0.000000000000000000 ) ) ;
#20828=CARTESIAN_POINT ( 'NONE',  ( -27.00000000000000355, 195.5750000012290570, -15.58845726811989429 ) ) ;
#20832=CARTESIAN_POINT ( 'NONE',  ( 23.99999999999999645, 248.9500000000000171, -5.196152422706631135 ) ) ;
#20833=CARTESIAN_POINT ( 'NONE',  ( -1.926257025242585782E-15, 195.1906250006145456, -31.45816453501076637 ) ) ;
#20838=CARTESIAN_POINT ( 'NONE',  ( 27.24356964374999635, 196.0156250006145626, -15.72908226750539029 ) ) ;
#20839=CARTESIAN_POINT ( 'NONE',  ( 15.24356964374999990, 239.8468750006145171, 0.000000000000000000 ) ) ;
#20842=CARTESIAN_POINT ( 'NONE',  ( 18.12178482187500350, 246.7843750006145456, 4.985214923628407568 ) ) ;
#20850=CARTESIAN_POINT ( 'NONE',  ( 23.87821517812500005, 240.8968750006145285, 4.985214923628404016 ) ) ;
#20869=CARTESIAN_POINT ( 'NONE',  ( 15.24356964374999990, 241.1593750006145171, -3.323476615752268604 ) ) ;
#20873=CARTESIAN_POINT ( 'NONE',  ( 27.24356964375000700, 199.1468750006145285, 15.72908226750537075 ) ) ;
#20881=CARTESIAN_POINT ( 'NONE',  ( 23.87821517812499650, 247.3468750006144887, -4.985214923628404904 ) ) ;
#20891=CARTESIAN_POINT ( 'NONE',  ( 18.12178482187500350, 248.4718750006145171, 4.985214923628407568 ) ) ;
#20904=DIRECTION ( 'NONE',  ( -0.000000000000000000, -1.000000000000000000, -0.000000000000000000 ) ) ;
#20914=CARTESIAN_POINT ( 'NONE',  ( 27.00000000000001421, 195.8000000012290513, 15.58845726811988897 ) ) ;
#20918=CARTESIAN_POINT ( 'NONE',  ( 26.75643035624999655, 243.7843750006145456, -7.049594010296217766E-16 ) ) ;
#20920=CARTESIAN_POINT ( 'NONE',  ( 19.00081571707366379, 239.8729221881839067, -5.492723647597353320 ) ) ;
#20922=CARTESIAN_POINT ( 'NONE',  ( 26.99999999999999645, 245.3312500012290513, -7.347880794884117764E-16 ) ) ;
#20925=CARTESIAN_POINT ( 'NONE',  ( 1.069080835302379631E-14, 197.9750000012290343, 27.00000000000000000 ) ) ;
#20929=EDGE_CURVE ( 'NONE', #31515, #20196, #34637, .T. ) ;
#20937=CARTESIAN_POINT ( 'NONE',  ( 26.75643035624999655, 247.3093750006144944, -3.323476615752271712 ) ) ;
#20942=( NAMED_UNIT ( * ) PLANE_ANGLE_UNIT ( ) SI_UNIT ( $, .RADIAN. ) );
#20951=CARTESIAN_POINT ( 'NONE',  ( 20.99999999999995381, 244.7125000000000057, 5.999999999999998224 ) ) ;
#20965=CARTESIAN_POINT ( 'NONE',  ( 20.99999999999997868, 210.0000000000000000, -5.999999999999999112 ) ) ;
#20967=CARTESIAN_POINT ( 'NONE',  ( 15.24356964374999990, 247.1593750006145171, 0.000000000000000000 ) ) ;
#20968=EDGE_LOOP ( 'NONE', ( #7620, #23337 ) ) ;
#20975=CARTESIAN_POINT ( 'NONE',  ( 26.99999999999999645, 242.0875000000000057, 3.464101615137751278 ) ) ;
#20978=ORIENTED_EDGE ( 'NONE', *, *, #15002, .F. ) ;
#20980=CARTESIAN_POINT ( 'NONE',  ( -26.99999999999999645, 195.9875000000000114, 15.58845726811991561 ) ) ;
#20987=CARTESIAN_POINT ( 'NONE',  ( 23.99999999999999645, 249.4000000000000057, -5.196152422706631135 ) ) ;
#20997=CARTESIAN_POINT ( 'NONE',  ( 13.62178482187501416, 198.1531250006145228, 23.59362340125806767 ) ) ;
#21005=CARTESIAN_POINT ( 'NONE',  ( 27.00000000000000355, 198.8750000000000284, -3.306546357697854128E-15 ) ) ;
#21024=CARTESIAN_POINT ( 'NONE',  ( 26.99999999999999645, 247.4875000000000398, 3.464101615137751278 ) ) ;
#21025=CARTESIAN_POINT ( 'NONE',  ( -13.62178482187498396, 197.1781250006145569, 23.59362340125808188 ) ) ;
#21029=CARTESIAN_POINT ( 'NONE',  ( 27.24356964375000345, 196.8781250006145171, -3.336375036156643733E-15 ) ) ;
#21030=CARTESIAN_POINT ( 'NONE',  ( 20.99999999999999645, 185.0294372515228645, 0.000000000000000000 ) ) ;
#21033=CARTESIAN_POINT ( 'NONE',  ( 21.00000000000000000, 247.7218750006145171, 6.646953231504538984 ) ) ;
#21035=ADVANCED_BREP_SHAPE_REPRESENTATION ( '', ( #33379, #17215 ), #29865 ) ;
#21040=CARTESIAN_POINT ( 'NONE',  ( -27.24356964375000345, 199.8593750006145342, 0.000000000000000000 ) ) ;
#21049=AXIS2_PLACEMENT_3D ( 'NONE', #20824, #3562, #28956 ) ;
#21058=CARTESIAN_POINT ( 'NONE',  ( 21.00000000000000000, 242.6593750006145171, 6.646953231504538984 ) ) ;
#21063=EDGE_CURVE ( 'NONE', #16244, #35488, #3502, .T. ) ;
#21065=LINE ( 'NONE', #29758, #24541 ) ;
#21070=VERTEX_POINT ( 'NONE', #31794 ) ;
#21071=VERTEX_POINT ( 'NONE', #34275 ) ;
#21072=CARTESIAN_POINT ( 'NONE',  ( 18.12178482187499640, 246.0718750006145115, -4.985214923628404904 ) ) ;
#21086=CARTESIAN_POINT ( 'NONE',  ( 23.87821517812499650, 249.5968750006145171, -4.985214923628404904 ) ) ;
#21088=PLANE ( 'NONE',  #30876 ) ;
#21091=CARTESIAN_POINT ( 'NONE',  ( -28.16023620420738993, 205.9774825840613346, 6.934657662760876917 ) ) ;
#21100=ORIENTED_EDGE ( 'NONE', *, *, #4954, .T. ) ;
#21109=LINE ( 'NONE', #32648, #14534 ) ;
#21111=CARTESIAN_POINT ( 'NONE',  ( 0.000000000000000000, 210.0000000000000284, -27.00000000000000000 ) ) ;
#21113=CARTESIAN_POINT ( 'NONE',  ( 15.00000000000000000, 243.2687500012290229, -3.464101615137752166 ) ) ;
#21116=CARTESIAN_POINT ( 'NONE',  ( 19.39230484541324273, 242.8924038105677141, 5.999999999999987566 ) ) ;
#21123=CARTESIAN_POINT ( 'NONE',  ( 15.24356964374999990, 244.7968750006145058, 0.000000000000000000 ) ) ;
#21138=CARTESIAN_POINT ( 'NONE',  ( 5.438367727407757775E-14, 198.5374999999999943, -27.00000000000000355 ) ) ;
#21146=FACE_OUTER_BOUND ( 'NONE', #27116, .T. ) ;
#21150=( BOUNDED_CURVE ( )  B_SPLINE_CURVE ( 2, ( #36669, #32895, #30439, #21543, #30246, #30807, #4458, #4273, #15847 ),
 .UNSPECIFIED., .F., .F. ) 
 B_SPLINE_CURVE_WITH_KNOTS ( ( 3, 2, 2, 2, 3 ),
 ( 0.01086956521739129364, 0.01449275362318840597, 0.02173913043478260809, 0.02898550724637681195, 0.03260869565217391908 ),
 .UNSPECIFIED. ) 
 CURVE ( )  GEOMETRIC_REPRESENTATION_ITEM ( )  RATIONAL_B_SPLINE_CURVE ( ( 0.9330127018922194093, 0.9330127018922191873, 1.000000000000000000, 0.8660254037844387076, 1.000000000000000000, 0.8660254037844387076, 1.000000000000000000, 0.9330127018922191873, 0.9330127018922192983 ) ) 
 REPRESENTATION_ITEM ( '' )  );
#21151=CARTESIAN_POINT ( 'NONE',  ( 15.00000000000000000, 247.3187500012290343, -3.464101615137752610 ) ) ;
#21153=CARTESIAN_POINT ( 'NONE',  ( 18.12178482187500350, 247.2343750006145342, 4.985214923628407568 ) ) ;
#21157=LINE ( 'NONE', #291, #15850 ) ;
#21160=FACE_OUTER_BOUND ( 'NONE', #35071, .T. ) ;
#21165=FACE_OUTER_BOUND ( 'NONE', #15406, .T. ) ;
#21174=CARTESIAN_POINT ( 'NONE',  ( 20.28004929560864511, 210.7199507044221320, 5.999999999998711253 ) ) ;
#21176=CARTESIAN_POINT ( 'NONE',  ( 15.00000000000000000, 245.4625000000000057, -3.464101615137752610 ) ) ;
#21184=CARTESIAN_POINT ( 'NONE',  ( -27.24356964374999990, 199.7656250006145342, -15.72908226750537786 ) ) ;
#21191=LINE ( 'NONE', #7154, #12012 ) ;
#21200=EDGE_CURVE ( 'NONE', #36238, #8445, #22174, .T. ) ;
#21207=AXIS2_PLACEMENT_3D ( 'NONE', #6596, #9068, #35586 ) ;
#21211=CARTESIAN_POINT ( 'NONE',  ( 21.00000000000000000, 246.0625000000000000, 6.928203230275506996 ) ) ;
#21212=CARTESIAN_POINT ( 'NONE',  ( -1.926257025242585782E-15, 196.9906250006145001, -31.45816453501076637 ) ) ;
#21217=CARTESIAN_POINT ( 'NONE',  ( -27.00000000000000355, 199.6625000012290343, 0.000000000000000000 ) ) ;
#21218=CARTESIAN_POINT ( 'NONE',  ( 26.75643035624999655, 240.0718750006145399, -7.049594010296217766E-16 ) ) ;
#21222=CARTESIAN_POINT ( 'NONE',  ( 18.12178482187500350, 246.3343750006145285, 4.985214923628407568 ) ) ;
#21239=CARTESIAN_POINT ( 'NONE',  ( 20.99999999999995026, 241.3375000000000341, -5.999999999999998224 ) ) ;
#21240=EDGE_CURVE ( 'NONE', #26868, #18985, #32448, .T. ) ;
#21246=CARTESIAN_POINT ( 'NONE',  ( 15.24356964375000167, 240.7843750006145171, 3.323476615752272600 ) ) ;
#21252=EDGE_CURVE ( 'NONE', #27758, #30367, #16589, .T. ) ;
#21254=CYLINDRICAL_SURFACE ( 'NONE', #31229, 5.999999999999999112 ) ;
#21259=VERTEX_POINT ( 'NONE', #30180 ) ;
#21260=CARTESIAN_POINT ( 'NONE',  ( 26.75643035624999655, 248.1718750006145342, -7.049594010296217766E-16 ) ) ;
#21266=DIRECTION ( 'NONE',  ( 0.000000000000000000, 0.000000000000000000, 1.000000000000000000 ) ) ;
#21274=CARTESIAN_POINT ( 'NONE',  ( 26.75643035624999655, 247.3093750006144944, -3.323476615752271268 ) ) ;
#21280=VERTEX_POINT ( 'NONE', #29608 ) ;
#21281=CARTESIAN_POINT ( 'NONE',  ( -28.51651240191029757, 203.9818979280190092, 5.277347936512516213 ) ) ;
#21286=CARTESIAN_POINT ( 'NONE',  ( 20.99999999999999645, 249.2687500012290513, 5.999999999999998224 ) ) ;
#21289=VERTEX_POINT ( 'NONE', #981 ) ;
#21290=CARTESIAN_POINT ( 'NONE',  ( 27.00000000000001421, 197.6000000012290627, 15.58845726811988897 ) ) ;
#21296=CARTESIAN_POINT ( 'NONE',  ( 5.727106289114498080E-15, 195.6125000000000398, 31.17691453623979214 ) ) ;
#21301=CYLINDRICAL_SURFACE ( 'NONE', #6352, 5.999999999999999112 ) ;
#21302=ORIENTED_EDGE ( 'NONE', *, *, #8088, .T. ) ;
#21303=CARTESIAN_POINT ( 'NONE',  ( 21.00000000000000000, 244.0937500012290400, -6.928203230275506996 ) ) ;
#21310=LINE ( 'NONE', #30198, #28014 ) ;
#21311=CARTESIAN_POINT ( 'NONE',  ( 18.12178482187499640, 244.2718750006145001, -4.985214923628404904 ) ) ;
#21315=VECTOR ( 'NONE', #15924, 1000.000000000000000 ) ;
#21325=AXIS2_PLACEMENT_3D ( 'NONE', #18301, #15071, #32684 ) ;
#21331=FACE_OUTER_BOUND ( 'NONE', #22442, .T. ) ;
#21332=VERTEX_POINT ( 'NONE', #33583 ) ;
#21338=CARTESIAN_POINT ( 'NONE',  ( -13.50000000000000533, 195.4250000000000114, -23.38268590217984411 ) ) ;
#21340=CARTESIAN_POINT ( 'NONE',  ( 23.87821517812500005, 249.5593750006145228, 4.985214923628404016 ) ) ;
#21342=CARTESIAN_POINT ( 'NONE',  ( 23.87821517812499650, 242.9593750006145285, -4.985214923628404904 ) ) ;
#21361=CARTESIAN_POINT ( 'NONE',  ( 26.99999999999999645, 243.4937500012290457, 3.464101615137751278 ) ) ;
#21362=CARTESIAN_POINT ( 'NONE',  ( 14.16903250681090398, 216.8309674931867903, 1.338899061175305771 ) ) ;
#21369=SHAPE_DEFINITION_REPRESENTATION ( #25269, #9842 ) ;
#21371=CARTESIAN_POINT ( 'NONE',  ( -13.62178482187500528, 197.9281250006145569, -23.59362340125807123 ) ) ;
#21384=CARTESIAN_POINT ( 'NONE',  ( 15.00000000000000178, 240.6437500012289945, 3.464101615137757051 ) ) ;
#21386=DIRECTION ( 'NONE',  ( 0.000000000000000000, 0.000000000000000000, 1.000000000000000000 ) ) ;
#21396=CARTESIAN_POINT ( 'NONE',  ( 15.00000000000000000, 245.5000000000000000, 0.000000000000000000 ) ) ;
#21398=CARTESIAN_POINT ( 'NONE',  ( 5.778771075727756162E-15, 196.7656250006145342, 31.45816453501076637 ) ) ;
#21403=CARTESIAN_POINT ( 'NONE',  ( 27.24356964375000345, 195.9781250006145399, -3.336375036156643733E-15 ) ) ;
#21404=CARTESIAN_POINT ( 'NONE',  ( 15.24356964375000167, 240.7843750006145171, 3.323476615752272600 ) ) ;
#21406=ADVANCED_FACE ( 'NONE', ( #16716 ), #36599, .T. ) ;
#21408=CARTESIAN_POINT ( 'NONE',  ( 21.00000000000000000, 244.7968750006145626, -6.646953231504538984 ) ) ;
#21414=CARTESIAN_POINT ( 'NONE',  ( 23.87821517812500005, 239.9968750006144944, 4.985214923628404016 ) ) ;
#21419=AXIS2_PLACEMENT_3D ( 'NONE', #1227, #3893, #27387 ) ;
#21425=CARTESIAN_POINT ( 'NONE',  ( 21.00000000000000000, 244.2624999999999886, 5.999999999999998224 ) ) ;
#21427=LINE ( 'NONE', #32969, #21315 ) ;
#21431=CARTESIAN_POINT ( 'NONE',  ( 20.99999999999997868, 210.0000000000000000, 5.999999999999999112 ) ) ;
#21432=CARTESIAN_POINT ( 'NONE',  ( 26.75643035624999655, 249.6718750006145342, -3.323476615752271712 ) ) ;
#21439=CARTESIAN_POINT ( 'NONE',  ( 17.48528137423856776, 206.4852813742385820, 5.999999999999996447 ) ) ;
#21443=ORIENTED_EDGE ( 'NONE', *, *, #31093, .T. ) ;
#21444=ORIENTED_EDGE ( 'NONE', *, *, #14737, .F. ) ;
#21445=AXIS2_PLACEMENT_3D ( 'NONE', #21531, #4260, #20777 ) ;
#21447=CARTESIAN_POINT ( 'NONE',  ( 21.00000000000000000, 246.9343750006145228, -6.646953231504538984 ) ) ;
#21453=DIRECTION ( 'NONE',  ( -0.000000000000000000, -1.000000000000000000, -0.000000000000000000 ) ) ;
#21456=ORIENTED_EDGE ( 'NONE', *, *, #211, .F. ) ;
#21461=CARTESIAN_POINT ( 'NONE',  ( 26.75643035624999655, 247.7593750006145399, -3.323476615752271268 ) ) ;
#21475=CARTESIAN_POINT ( 'NONE',  ( 15.00000000000000178, 241.4874999999999829, 3.464101615137757051 ) ) ;
#21484=CARTESIAN_POINT ( 'NONE',  ( 15.00000000000000000, 246.9062500012290400, 0.000000000000000000 ) ) ;
#21485=CARTESIAN_POINT ( 'NONE',  ( 13.50000000000001421, 195.2000000000000171, 23.38268590217984055 ) ) ;
#21492=CARTESIAN_POINT ( 'NONE',  ( 18.00000000000000355, 244.7312500012290570, 5.196152422706632912 ) ) ;
#21500=CARTESIAN_POINT ( 'NONE',  ( 21.00000000000000000, 244.0093750006145115, 6.646953231504538984 ) ) ;
#21513=CARTESIAN_POINT ( 'NONE',  ( 13.49999999999999645, 199.8499999999999943, -23.38268590217984766 ) ) ;
#21517=CARTESIAN_POINT ( 'NONE',  ( 15.00000000000000000, 244.2062500012290513, 0.000000000000000000 ) ) ;
#21522=DIRECTION ( 'NONE',  ( -0.000000000000000000, 1.000000000000000000, -0.000000000000000000 ) ) ;
#21527=CARTESIAN_POINT ( 'NONE',  ( 15.24356964374999990, 249.8218750006145399, -3.323476615752268604 ) ) ;
#21529=CARTESIAN_POINT ( 'NONE',  ( 18.12178482187499640, 244.8343750006145285, -4.985214923628404904 ) ) ;
#21531=CARTESIAN_POINT ( 'NONE',  ( 20.99999999999999645, 185.0294372515228645, 0.000000000000000000 ) ) ;
#21533=ADVANCED_FACE ( 'NONE', ( #30745 ), #36784, .F. ) ;
#21536=CYLINDRICAL_SURFACE ( 'NONE', #21419, 27.00000000000000000 ) ;
#21543=CARTESIAN_POINT ( 'NONE',  ( 26.99999999999999645, 249.4187500012290286, -3.464101615137755275 ) ) ;
#21550=AXIS2_PLACEMENT_3D ( 'NONE', #26162, #196, #3417 ) ;
#21551=CARTESIAN_POINT ( 'NONE',  ( -4.500000000000001776, 227.8255434699758837, 2.500000000000000000 ) ) ;
#21559=CARTESIAN_POINT ( 'NONE',  ( 27.24356964375000700, 198.6406250006145058, 15.72908226750537075 ) ) ;
#21585=CARTESIAN_POINT ( 'NONE',  ( 23.99999999999999645, 246.2500000000000000, -5.196152422706631135 ) ) ;
#21592=CARTESIAN_POINT ( 'NONE',  ( -26.99999999999998934, 199.2500000012290116, 15.58845726811991561 ) ) ;
#21595=CARTESIAN_POINT ( 'NONE',  ( 23.87821517812500005, 244.6093750006145342, 4.985214923628404016 ) ) ;
#21606=CARTESIAN_POINT ( 'NONE',  ( 0.000000000000000000, 210.0000000000000284, 0.000000000000000000 ) ) ;
#21610=CARTESIAN_POINT ( 'NONE',  ( -27.00000000000000355, 199.6625000012290343, 0.000000000000000000 ) ) ;
#21612=CARTESIAN_POINT ( 'NONE',  ( 19.39230484541326049, 248.1638461906613884, -5.999999999999994671 ) ) ;
#21614=CARTESIAN_POINT ( 'NONE',  ( 15.24356964375000167, 239.8843750006145399, 3.323476615752272600 ) ) ;
#21623=CARTESIAN_POINT ( 'NONE',  ( 23.87821517812499650, 242.9593750006145285, -4.985214923628404904 ) ) ;
#21628=VERTEX_POINT ( 'NONE', #22402 ) ;
#21629=CARTESIAN_POINT ( 'NONE',  ( 18.12178482187500350, 247.1218750006145228, 4.985214923628407568 ) ) ;
#21641=CARTESIAN_POINT ( 'NONE',  ( 23.87821517812500005, 246.2968750006145058, 4.985214923628404016 ) ) ;
#21643=CARTESIAN_POINT ( 'NONE',  ( 1.120210788295102201E-13, 196.7375000000000398, -27.00000000000000711 ) ) ;
#21647=ORIENTED_EDGE ( 'NONE', *, *, #6091, .F. ) ;
#21654=ADVANCED_FACE ( 'NONE', ( #7992 ), #19566, .F. ) ;
#21662=CARTESIAN_POINT ( 'NONE',  ( 15.00000000000000000, 245.0124999999999602, -3.464101615137752610 ) ) ;
#21663=CARTESIAN_POINT ( 'NONE',  ( 27.24356964375000700, 198.2468750006145513, 15.72908226750537075 ) ) ;
#21665=CARTESIAN_POINT ( 'NONE',  ( 20.99999999999999289, 244.0374999999999943, -5.999999999999997335 ) ) ;
#21668=CARTESIAN_POINT ( 'NONE',  ( 15.00000000000000000, 245.0687500012290627, -3.464101615137752166 ) ) ;
#21677=CARTESIAN_POINT ( 'NONE',  ( 15.24356964374999990, 245.2468750006145228, 0.000000000000000000 ) ) ;
#21690=DIRECTION ( 'NONE',  ( -0.000000000000000000, -1.000000000000000000, -0.000000000000000000 ) ) ;
#21693=CARTESIAN_POINT ( 'NONE',  ( 0.000000000000000000, 210.0000000000000284, 0.000000000000000000 ) ) ;
#21710=CARTESIAN_POINT ( 'NONE',  ( 26.75643035624999655, 244.2343750006145342, -7.049594010296217766E-16 ) ) ;
#21712=CARTESIAN_POINT ( 'NONE',  ( 15.00000000000000000, 249.5687500012290627, -3.464101615137752610 ) ) ;
#21724=DIRECTION ( 'NONE',  ( 1.000000000000000000, -0.000000000000000000, -0.000000000000000000 ) ) ;
#21732=CARTESIAN_POINT ( 'NONE',  ( 15.00000000000000000, 243.7187500012290968, -3.464101615137752610 ) ) ;
#21734=CARTESIAN_POINT ( 'NONE',  ( 20.99999999999999645, 185.0294372515228645, 0.000000000000000000 ) ) ;
#21739=EDGE_CURVE ( 'NONE', #7058, #32512, #5810, .T. ) ;
#21742=CARTESIAN_POINT ( 'NONE',  ( -27.24356964375000345, 198.4531250006145342, 0.000000000000000000 ) ) ;
#21748=CARTESIAN_POINT ( 'NONE',  ( -4.694659320240884604E-14, 197.8625000000000114, 27.00000000000000000 ) ) ;
#21761=CARTESIAN_POINT ( 'NONE',  ( 7.234628195640322446, 199.2325961894323711, 26.99999999999999645 ) ) ;
#21764=CARTESIAN_POINT ( 'NONE',  ( 13.50000000000001421, 198.4625000012290172, 23.38268590217984055 ) ) ;
#21765=ORIENTED_EDGE ( 'NONE', *, *, #26065, .T. ) ;
#21769=CARTESIAN_POINT ( 'NONE',  ( 23.99999999999999645, 244.9000000000000057, -5.196152422706631135 ) ) ;
#21770=CARTESIAN_POINT ( 'NONE',  ( 3.306546357697853733E-15, 202.0000000000000000, 27.00000000000000000 ) ) ;
#21774=VERTEX_POINT ( 'NONE', #37158 ) ;
#21776=CARTESIAN_POINT ( 'NONE',  ( -27.00000000000000355, 197.8250000012290286, -15.58845726811989429 ) ) ;
#21780=CARTESIAN_POINT ( 'NONE',  ( 23.87821517812500005, 245.0593750006145228, 4.985214923628404016 ) ) ;
#21786=CARTESIAN_POINT ( 'NONE',  ( 13.62178482187499640, 199.7093750006145285, -23.59362340125807123 ) ) ;
#21802=CARTESIAN_POINT ( 'NONE',  ( 15.24356964374999990, 240.7468750006144944, 0.000000000000000000 ) ) ;
#21806=CARTESIAN_POINT ( 'NONE',  ( 13.62178482187499640, 197.4593750006145285, -23.59362340125807123 ) ) ;
#21809=CARTESIAN_POINT ( 'NONE',  ( 18.12178482187500350, 242.7343750006145342, 4.985214923628407568 ) ) ;
#21815=CARTESIAN_POINT ( 'NONE',  ( 26.75643035624999655, 243.6343750006145115, 3.323476615752267715 ) ) ;
#21821=ORIENTED_EDGE ( 'NONE', *, *, #15154, .T. ) ;
#21829=CARTESIAN_POINT ( 'NONE',  ( 23.87821517812500005, 246.7468750006145228, 4.985214923628404016 ) ) ;
#21830=CARTESIAN_POINT ( 'NONE',  ( 26.99999999999999645, 240.3250000000000171, -7.347880794884117764E-16 ) ) ;
#21840=CARTESIAN_POINT ( 'NONE',  ( 23.99999999999999645, 242.7062500012290513, -5.196152422706631135 ) ) ;
#21843=ORIENTED_EDGE ( 'NONE', *, *, #2504, .F. ) ;
#21846=DIRECTION ( 'NONE',  ( 0.000000000000000000, 0.000000000000000000, 1.000000000000000000 ) ) ;
#21850=CARTESIAN_POINT ( 'NONE',  ( 27.24356964375000700, 198.6968750006145115, 15.72908226750537075 ) ) ;
#21852=CARTESIAN_POINT ( 'NONE',  ( 26.99999999999999645, 243.9625000000000057, -3.464101615137755275 ) ) ;
#21855=CARTESIAN_POINT ( 'NONE',  ( 15.00000000000000178, 244.6937500012290627, 3.464101615137757051 ) ) ;
#21864=EDGE_CURVE ( 'NONE', #25338, #21070, #33296, .T. ) ;
#21872=CARTESIAN_POINT ( 'NONE',  ( -13.45723662585736591, 216.2569280196711645, -5.070466603772765701 ) ) ;
#21880=CARTESIAN_POINT ( 'NONE',  ( -28.88589706552147263, 202.4236885276250746, -2.582340647126037059 ) ) ;
#21887=DIRECTION ( 'NONE',  ( -0.000000000000000000, 1.000000000000000000, -0.000000000000000000 ) ) ;
#21891=CARTESIAN_POINT ( 'NONE',  ( 26.75643035624999655, 247.7968750006145342, 3.323476615752267715 ) ) ;
#21893=CARTESIAN_POINT ( 'NONE',  ( 15.24356964374999990, 243.5218750006145569, -3.323476615752268604 ) ) ;
#21908=LINE ( 'NONE', #18887, #6829 ) ;
#21909=CARTESIAN_POINT ( 'NONE',  ( 20.99999999999997868, 245.1625000000000227, 5.999999999999999112 ) ) ;
#21911=CIRCLE ( 'NONE', #32171, 28.99999999999999645 ) ;
#21915=CARTESIAN_POINT ( 'NONE',  ( 19.06670604969872329, 215.1554505341390211, 5.693556627485715893 ) ) ;
#21923=( BOUNDED_SURFACE ( )  B_SPLINE_SURFACE ( 1, 2, ( 
 ( #16781, #25486, #28326, #2364, #33649, #36480, #25301, #16965, #10522, #25672, #8250, #4831, #36853, #22100, #13937, #22660, #7688, #19269, #37226, #30809, #11272, #16411, #13755, #22285, #1989, #36672, #22843, #31361, #8062, #13561, #34205, #25114, #19824, #33839, #19450, #7876, #31544, #5385, #28508, #31000, #5019, #28143, #34389, #2551, #10897, #22469, #2173, #34017, #14118, #19638, #5569, #26042, #11822, #31731, #2915, #443, #11635, #23392, #23580, #20742, #6131, #5759, #32284, #34572, #5945, #20937, #23767, #26596, #17708, #14671, #3102, #8612, #26221, #35124, #34939, #6328, #69, #8984, #17337, #14486, #12008, #23209, #20556, #9173, #17899, #29249, #28881, #29443, #20182, #17524, #32471, #35308, #34758, #29631, #3290, #6516, #257, #3667, #627, #8801, #18091, #25856, #37405, #20371, #29059, #11455, #3479, #15048, #12195, #31915, #23024, #9362, #32099, #14862, #26409, #3852, #15237, #18845, #35501, #26787, #21677, #12765, #26977, #33231, #1383, #9549, #7269, #12955, #33043, #18469, #27167, #4040, #21123, #30390, #30010, #18275, #4412, #15995, #24333, #35874, #4226, #35687, #24145, #9917, #1003, #9740, #21311, #15612, #32847, #818, #1190, #23958, #24515, #21500, #7090, #18660, #30199, #32662, #27542, #15803, #36064, #12389, #6703, #29817, #6894, #27353, #15428, #10107, #12578, #15358, #34684, #749, #26912, #12320, #11569, #26340, #34874, #23142, #11755, #23893, #6448, #20673, #8729, #560, #20302, #23701, #17455, #32029, #3033, #21058, #12126, #35244, #31843, #29752, #6059, #14605, #32408, #9106, #5876, #3783, #23512, #35058, #28992, #29373, #9482, #26156, #17646, #189, #23323, #6636, #18021, #3222, #26717, #32596, #32221, #6260, #8915, #20490, #29180, #14794, #376, #11943, #18210, #29566, #17837, #3411, #14980, #26529, #9297, #20869, #3603, #35434, #15169, #10227, #1689, #18783, #35623, #30701, #13078, #21246, #21802, #1502, #24267, #4166, #24450, #21990, #18397, #940, #33165, #36000, #27476, #7390, #19153, #24632, #9669, #29946, #32786, #36182, #18592, #3974, #10037, #36368, #13264, #21614, #10415, #6821, #32972, #1129, #18963 ),
 ( #4348, #1317, #12885, #33354, #27665, #21432, #27286, #33537, #16113, #30517, #15927, #7577, #7211, #30323, #12695, #4537, #24816, #7025, #12514, #4721, #15547, #27105, #16298, #24078, #30135, #35811, #9853, #15736, #722, #6424, #17808, #9083, #29350, #32199, #28973, #29727, #20653, #11734, #15334, #26886, #26505, #12102, #29541, #14773, #3197, #919, #3013, #355, #12487, #26693, #3580, #9456, #26318, #35600, #17998, #8892, #35038, #21033, #32009, #20282, #3760, #14583, #31822, #32570, #14959, #6039, #6611, #12295, #23867, #35407, #15142, #3389, #6234, #536, #23676, #26135, #24054, #35221, #23306, #5857, #17434, #9271, #20842, #18185, #11920, #23487, #32384, #17626, #169, #34852, #20470, #29155, #24973, #18758, #21222, #16091, #15905, #36160, #27452, #13056, #6798, #27826, #35978, #27642, #13425, #36345, #18942, #15526, #10015, #9645, #4326, #24611, #32761, #18372, #10390, #29919, #21966, #3951, #24429, #32947, #27081, #9830, #33512, #4517, #30300, #1106, #10206, #12674, #21780, #24242, #30113, #35788, #19132, #33330, #7370, #21408, #1856, #4143, #7556, #1481, #21595, #33145, #7002, #7189, #30494, #1671, #13245, #18571, #24794, #15715, #27266, #30679, #1291, #4698, #16279, #12863, #16835, #4885, #5434, #7739, #16652, #31596, #34440, #13620, #2782, #13985, #5619, #25355, #14355, #11322, #19503, #17203, #36532, #28742, #25723, #8480, #2597, #22892, #36723, #37089, #2041, #19871, #34069, #10576, #22154, #10949, #22523, #33701, #28376, #20049, #30860, #5071, #19323, #28009, #16465, #31415, #28196, #14168, #25171, #8118, #19690, #10764, #22335, #7929, #33887, #36901, #31050, #2226, #17016, #13806, #31230, #5258, #2413, #25537, #11137, #22714, #37276, #34257, #8300, #28556, #6188, #23073, #18140, #493, #8664, #35175, #26459, #11688, #29110, #11871, #9412, #5811, #25909, #20609, #23440, #14910, #32338, #6565, #12059, #34619, #17392, #20233, #23633, #5998, #28933, #34993, #23819, #26648, #9037, #35361, #31776, #20423, #26092, #6376, #8849, #9222, #20795, #23261, #17761, #17578, #34805, #17951, #29302, #26273, #306, #29494, #15098, #31967, #14725 ) ),
 .UNSPECIFIED., .F., .F., .F. ) 
 B_SPLINE_SURFACE_WITH_KNOTS ( ( 2, 2 ),
 ( 3, 2, 2, 2, 2, 2, 2, 2, 2, 2, 2, 2, 2, 2, 2, 2, 2, 2, 2, 2, 2, 2, 2, 2, 2, 2, 2, 2, 2, 2, 2, 2, 2, 2, 2, 2, 2, 2, 2, 2, 2, 2, 2, 2, 2, 2, 2, 2, 2, 2, 2, 2, 2, 2, 2, 2, 2, 2, 2, 2, 2, 2, 2, 2, 2, 2, 2, 2, 2, 2, 2, 2, 2, 2, 2, 2, 2, 2, 2, 2, 2, 2, 2, 2, 2, 2, 2, 2, 2, 2, 2, 2, 2, 2, 2, 2, 2, 2, 2, 2, 2, 2, 2, 2, 2, 2, 2, 2, 2, 2, 2, 2, 2, 2, 2, 2, 2, 2, 2, 2, 2, 2, 2, 2, 2, 2, 2, 2, 2, 2, 2, 2, 2, 2, 3 ),
 ( 0.000000000000000000, 1.000000000000000000 ),
 ( 0.000000000000000000, 0.007246376811594202987, 0.01449275362318840597, 0.02173913043478260809, 0.02898550724637681195, 0.03623188405797101580, 0.04347826086956521618, 0.05072463768115942351, 0.05797101449275362389, 0.06521739130434782428, 0.07246376811594203160, 0.07971014492753622505, 0.08695652173913043237, 0.09420289855072463969, 0.1014492753623188470, 0.1086956521739130405, 0.1159420289855072478, 0.1231884057971014551, 0.1304347826086956486, 0.1376811594202898559, 0.1449275362318840632, 0.1521739130434782705, 0.1594202898550724501, 0.1666666666666666574, 0.1739130434782608647, 0.1811594202898550721, 0.1884057971014492794, 0.1956521739130434867, 0.2028985507246376940, 0.2101449275362318736, 0.2173913043478260809, 0.2246376811594202882, 0.2318840579710144956, 0.2391304347826087029, 0.2463768115942029102, 0.2536231884057971175, 0.2608695652173912971, 0.2681159420289855322, 0.2753623188405797118, 0.2826086956521738913, 0.2898550724637681264, 0.2971014492753623060, 0.3043478260869565410, 0.3115942028985507206, 0.3188405797101449002, 0.3260869565217391353, 0.3333333333333333148, 0.3405797101449275499, 0.3478260869565217295, 0.3550724637681159646, 0.3623188405797101441, 0.3695652173913043237, 0.3768115942028985588, 0.3840579710144927383, 0.3913043478260869734, 0.3985507246376811530, 0.4057971014492753881, 0.4130434782608695676, 0.4202898550724637472, 0.4275362318840579823, 0.4347826086956521618, 0.4420289855072463969, 0.4492753623188405765, 0.4565217391304347561, 0.4637681159420289911, 0.4710144927536231707, 0.4782608695652174058, 0.4855072463768115854, 0.4927536231884058204, 0.5000000000000000000, 0.5072463768115942351, 0.5144927536231883591, 0.5217391304347825942, 0.5289855072463768293, 0.5362318840579710644, 0.5434782608695651884, 0.5507246376811594235, 0.5579710144927536586, 0.5652173913043477826, 0.5724637681159420177, 0.5797101449275362528, 0.5869565217391304879, 0.5942028985507246119, 0.6014492753623188470, 0.6086956521739130821, 0.6159420289855072062, 0.6231884057971014412, 0.6304347826086956763, 0.6376811594202898004, 0.6449275362318840354, 0.6521739130434782705, 0.6594202898550725056, 0.6666666666666666297, 0.6739130434782608647, 0.6811594202898550998, 0.6884057971014492239, 0.6956521739130434590, 0.7028985507246376940, 0.7101449275362319291, 0.7173913043478260532, 0.7246376811594202882, 0.7318840579710145233, 0.7391304347826086474, 0.7463768115942028825, 0.7536231884057971175, 0.7608695652173913526, 0.7681159420289854767, 0.7753623188405797118, 0.7826086956521739468, 0.7898550724637680709, 0.7971014492753623060, 0.8043478260869565410, 0.8115942028985507761, 0.8188405797101449002, 0.8260869565217391353, 0.8333333333333333703, 0.8405797101449274944, 0.8478260869565217295, 0.8550724637681159646, 0.8623188405797101996, 0.8695652173913043237, 0.8768115942028985588, 0.8840579710144927938, 0.8913043478260869179, 0.8985507246376811530, 0.9057971014492753881, 0.9130434782608695121, 0.9202898550724637472, 0.9275362318840579823, 0.9347826086956522174, 0.9420289855072463414, 0.9492753623188405765, 0.9565217391304348116, 0.9637681159420289356, 0.9662082973083875315 ),
 .UNSPECIFIED. ) 
 GEOMETRIC_REPRESENTATION_ITEM ( )  RATIONAL_B_SPLINE_SURFACE ( (
 ( 1.000000000000000000, 0.8660254037844387076, 1.000000000000000000, 0.8660254037844387076, 1.000000000000000000, 0.8660254037844387076, 1.000000000000000000, 0.8660254037844387076, 1.000000000000000000, 0.8660254037844387076, 1.000000000000000000, 0.8660254037844387076, 1.000000000000000000, 0.8660254037844387076, 1.000000000000000000, 0.8660254037844387076, 1.000000000000000000, 0.8660254037844387076, 1.000000000000000000, 0.8660254037844387076, 1.000000000000000000, 0.8660254037844387076, 1.000000000000000000, 0.8660254037844387076, 1.000000000000000000, 0.8660254037844387076, 1.000000000000000000, 0.8660254037844387076, 1.000000000000000000, 0.8660254037844387076, 1.000000000000000000, 0.8660254037844387076, 1.000000000000000000, 0.8660254037844387076, 1.000000000000000000, 0.8660254037844387076, 1.000000000000000000, 0.8660254037844387076, 1.000000000000000000, 0.8660254037844387076, 1.000000000000000000, 0.8660254037844387076, 1.000000000000000000, 0.8660254037844387076, 1.000000000000000000, 0.8660254037844387076, 1.000000000000000000, 0.8660254037844387076, 1.000000000000000000, 0.8660254037844387076, 1.000000000000000000, 0.8660254037844387076, 1.000000000000000000, 0.8660254037844387076, 1.000000000000000000, 0.8660254037844387076, 1.000000000000000000, 0.8660254037844387076, 1.000000000000000000, 0.8660254037844387076, 1.000000000000000000, 0.8660254037844387076, 1.000000000000000000, 0.8660254037844387076, 1.000000000000000000, 0.8660254037844387076, 1.000000000000000000, 0.8660254037844387076, 1.000000000000000000, 0.8660254037844387076, 1.000000000000000000, 0.8660254037844387076, 1.000000000000000000, 0.8660254037844387076, 1.000000000000000000, 0.8660254037844387076, 1.000000000000000000, 0.8660254037844387076, 1.000000000000000000, 0.8660254037844387076, 1.000000000000000000, 0.8660254037844387076, 1.000000000000000000, 0.8660254037844387076, 1.000000000000000000, 0.8660254037844387076, 1.000000000000000000, 0.8660254037844387076, 1.000000000000000000, 0.8660254037844387076, 1.000000000000000000, 0.8660254037844387076, 1.000000000000000000, 0.8660254037844387076, 1.000000000000000000, 0.8660254037844387076, 1.000000000000000000, 0.8660254037844387076, 1.000000000000000000, 0.8660254037844387076, 1.000000000000000000, 0.8660254037844387076, 1.000000000000000000, 0.8660254037844387076, 1.000000000000000000, 0.8660254037844387076, 1.000000000000000000, 0.8660254037844387076, 1.000000000000000000, 0.8660254037844387076, 1.000000000000000000, 0.8660254037844387076, 1.000000000000000000, 0.8660254037844387076, 1.000000000000000000, 0.8660254037844387076, 1.000000000000000000, 0.8660254037844387076, 1.000000000000000000, 0.8660254037844387076, 1.000000000000000000, 0.8660254037844387076, 1.000000000000000000, 0.8660254037844387076, 1.000000000000000000, 0.8660254037844387076, 1.000000000000000000, 0.8660254037844387076, 1.000000000000000000, 0.8660254037844387076, 1.000000000000000000, 0.8660254037844387076, 1.000000000000000000, 0.8660254037844387076, 1.000000000000000000, 0.8660254037844387076, 1.000000000000000000, 0.8660254037844387076, 1.000000000000000000, 0.8660254037844387076, 1.000000000000000000, 0.8660254037844387076, 1.000000000000000000, 0.8660254037844387076, 1.000000000000000000, 0.8660254037844387076, 1.000000000000000000, 0.8660254037844387076, 1.000000000000000000, 0.8660254037844387076, 1.000000000000000000, 0.8660254037844387076, 1.000000000000000000, 0.8660254037844387076, 1.000000000000000000, 0.8660254037844387076, 1.000000000000000000, 0.8660254037844387076, 1.000000000000000000, 0.8660254037844387076, 1.000000000000000000, 0.8660254037844387076, 1.000000000000000000, 0.8660254037844387076, 1.000000000000000000, 0.8660254037844387076, 1.000000000000000000, 0.8660254037844387076, 1.000000000000000000, 0.8660254037844387076, 1.000000000000000000, 0.8660254037844387076, 1.000000000000000000, 0.8660254037844387076, 1.000000000000000000, 0.8660254037844387076, 1.000000000000000000, 0.8660254037844387076, 1.000000000000000000, 0.8660254037844387076, 1.000000000000000000, 0.8660254037844387076, 1.000000000000000000, 0.8660254037844387076, 1.000000000000000000, 0.8660254037844387076, 1.000000000000000000, 0.8660254037844387076, 1.000000000000000000, 0.8660254037844387076, 1.000000000000000000, 0.8660254037844387076, 1.000000000000000000, 0.8660254037844387076, 1.000000000000000000, 0.8660254037844387076, 1.000000000000000000, 0.8660254037844387076, 1.000000000000000000, 0.8660254037844387076, 1.000000000000000000, 0.8660254037844387076, 1.000000000000000000, 0.8660254037844387076, 1.000000000000000000, 0.8660254037844387076, 1.000000000000000000, 0.8660254037844387076, 1.000000000000000000, 0.8660254037844387076, 1.000000000000000000, 0.8660254037844387076, 1.000000000000000000, 0.8660254037844387076, 1.000000000000000000, 0.8660254037844387076, 1.000000000000000000, 0.8660254037844387076, 1.000000000000000000, 0.8660254037844387076, 1.000000000000000000, 0.8660254037844387076, 1.000000000000000000, 0.8660254037844387076, 1.000000000000000000, 0.8660254037844387076, 1.000000000000000000, 0.8660254037844387076, 1.000000000000000000, 0.8660254037844387076, 1.000000000000000000, 0.8660254037844387076, 1.000000000000000000, 0.8660254037844387076, 1.000000000000000000, 0.8660254037844387076, 1.000000000000000000, 0.8660254037844387076, 1.000000000000000000, 0.8660254037844387076, 1.000000000000000000, 0.8660254037844387076, 1.000000000000000000, 0.8660254037844387076, 1.000000000000000000, 0.8660254037844387076, 1.000000000000000000, 0.8660254037844387076, 1.000000000000000000, 0.8660254037844387076, 1.000000000000000000, 0.8660254037844387076, 1.000000000000000000, 0.8660254037844387076, 1.000000000000000000, 0.8660254037844387076, 1.000000000000000000, 0.8660254037844387076, 1.000000000000000000, 0.8660254037844387076, 1.000000000000000000, 0.8660254037844387076, 1.000000000000000000, 0.8660254037844387076, 1.000000000000000000, 0.8660254037844387076, 1.000000000000000000, 0.9548847207714133978, 0.9401541335272454170),
 ( 1.000000000000000000, 0.8660254037844387076, 1.000000000000000000, 0.8660254037844387076, 1.000000000000000000, 0.8660254037844387076, 1.000000000000000000, 0.8660254037844387076, 1.000000000000000000, 0.8660254037844387076, 1.000000000000000000, 0.8660254037844387076, 1.000000000000000000, 0.8660254037844387076, 1.000000000000000000, 0.8660254037844387076, 1.000000000000000000, 0.8660254037844387076, 1.000000000000000000, 0.8660254037844387076, 1.000000000000000000, 0.8660254037844387076, 1.000000000000000000, 0.8660254037844387076, 1.000000000000000000, 0.8660254037844387076, 1.000000000000000000, 0.8660254037844387076, 1.000000000000000000, 0.8660254037844387076, 1.000000000000000000, 0.8660254037844387076, 1.000000000000000000, 0.8660254037844387076, 1.000000000000000000, 0.8660254037844387076, 1.000000000000000000, 0.8660254037844387076, 1.000000000000000000, 0.8660254037844387076, 1.000000000000000000, 0.8660254037844387076, 1.000000000000000000, 0.8660254037844387076, 1.000000000000000000, 0.8660254037844387076, 1.000000000000000000, 0.8660254037844387076, 1.000000000000000000, 0.8660254037844387076, 1.000000000000000000, 0.8660254037844387076, 1.000000000000000000, 0.8660254037844387076, 1.000000000000000000, 0.8660254037844387076, 1.000000000000000000, 0.8660254037844387076, 1.000000000000000000, 0.8660254037844387076, 1.000000000000000000, 0.8660254037844387076, 1.000000000000000000, 0.8660254037844387076, 1.000000000000000000, 0.8660254037844387076, 1.000000000000000000, 0.8660254037844387076, 1.000000000000000000, 0.8660254037844387076, 1.000000000000000000, 0.8660254037844387076, 1.000000000000000000, 0.8660254037844387076, 1.000000000000000000, 0.8660254037844387076, 1.000000000000000000, 0.8660254037844387076, 1.000000000000000000, 0.8660254037844387076, 1.000000000000000000, 0.8660254037844387076, 1.000000000000000000, 0.8660254037844387076, 1.000000000000000000, 0.8660254037844387076, 1.000000000000000000, 0.8660254037844387076, 1.000000000000000000, 0.8660254037844387076, 1.000000000000000000, 0.8660254037844387076, 1.000000000000000000, 0.8660254037844387076, 1.000000000000000000, 0.8660254037844387076, 1.000000000000000000, 0.8660254037844387076, 1.000000000000000000, 0.8660254037844387076, 1.000000000000000000, 0.8660254037844387076, 1.000000000000000000, 0.8660254037844387076, 1.000000000000000000, 0.8660254037844387076, 1.000000000000000000, 0.8660254037844387076, 1.000000000000000000, 0.8660254037844387076, 1.000000000000000000, 0.8660254037844387076, 1.000000000000000000, 0.8660254037844387076, 1.000000000000000000, 0.8660254037844387076, 1.000000000000000000, 0.8660254037844387076, 1.000000000000000000, 0.8660254037844387076, 1.000000000000000000, 0.8660254037844387076, 1.000000000000000000, 0.8660254037844387076, 1.000000000000000000, 0.8660254037844387076, 1.000000000000000000, 0.8660254037844387076, 1.000000000000000000, 0.8660254037844387076, 1.000000000000000000, 0.8660254037844387076, 1.000000000000000000, 0.8660254037844387076, 1.000000000000000000, 0.8660254037844387076, 1.000000000000000000, 0.8660254037844387076, 1.000000000000000000, 0.8660254037844387076, 1.000000000000000000, 0.8660254037844387076, 1.000000000000000000, 0.8660254037844387076, 1.000000000000000000, 0.8660254037844387076, 1.000000000000000000, 0.8660254037844387076, 1.000000000000000000, 0.8660254037844387076, 1.000000000000000000, 0.8660254037844387076, 1.000000000000000000, 0.8660254037844387076, 1.000000000000000000, 0.8660254037844387076, 1.000000000000000000, 0.8660254037844387076, 1.000000000000000000, 0.8660254037844387076, 1.000000000000000000, 0.8660254037844387076, 1.000000000000000000, 0.8660254037844387076, 1.000000000000000000, 0.8660254037844387076, 1.000000000000000000, 0.8660254037844387076, 1.000000000000000000, 0.8660254037844387076, 1.000000000000000000, 0.8660254037844387076, 1.000000000000000000, 0.8660254037844387076, 1.000000000000000000, 0.8660254037844387076, 1.000000000000000000, 0.8660254037844387076, 1.000000000000000000, 0.8660254037844387076, 1.000000000000000000, 0.8660254037844387076, 1.000000000000000000, 0.8660254037844387076, 1.000000000000000000, 0.8660254037844387076, 1.000000000000000000, 0.8660254037844387076, 1.000000000000000000, 0.8660254037844387076, 1.000000000000000000, 0.8660254037844387076, 1.000000000000000000, 0.8660254037844387076, 1.000000000000000000, 0.8660254037844387076, 1.000000000000000000, 0.8660254037844387076, 1.000000000000000000, 0.8660254037844387076, 1.000000000000000000, 0.8660254037844387076, 1.000000000000000000, 0.8660254037844387076, 1.000000000000000000, 0.8660254037844387076, 1.000000000000000000, 0.8660254037844387076, 1.000000000000000000, 0.8660254037844387076, 1.000000000000000000, 0.8660254037844387076, 1.000000000000000000, 0.8660254037844387076, 1.000000000000000000, 0.8660254037844387076, 1.000000000000000000, 0.8660254037844387076, 1.000000000000000000, 0.8660254037844387076, 1.000000000000000000, 0.8660254037844387076, 1.000000000000000000, 0.8660254037844387076, 1.000000000000000000, 0.8660254037844387076, 1.000000000000000000, 0.8660254037844387076, 1.000000000000000000, 0.8660254037844387076, 1.000000000000000000, 0.8660254037844387076, 1.000000000000000000, 0.8660254037844387076, 1.000000000000000000, 0.8660254037844387076, 1.000000000000000000, 0.8660254037844387076, 1.000000000000000000, 0.8660254037844387076, 1.000000000000000000, 0.8660254037844387076, 1.000000000000000000, 0.8660254037844387076, 1.000000000000000000, 0.8660254037844387076, 1.000000000000000000, 0.8660254037844387076, 1.000000000000000000, 0.8660254037844387076, 1.000000000000000000, 0.8660254037844387076, 1.000000000000000000, 0.8660254037844387076, 1.000000000000000000, 0.8660254037844387076, 1.000000000000000000, 0.8660254037844387076, 1.000000000000000000, 0.8660254037844387076, 1.000000000000000000, 0.8660254037844387076, 1.000000000000000000, 0.8660254037844387076, 1.000000000000000000, 0.8660254037844387076, 1.000000000000000000, 0.9548847207714133978, 0.9401541335272454170) ) ) 
 REPRESENTATION_ITEM ( '' )  SURFACE ( )  );
#21926=CARTESIAN_POINT ( 'NONE',  ( -13.62178482187498396, 195.8281250006145342, 23.59362340125808188 ) ) ;
#21939=ADVANCED_FACE ( 'NONE', ( #27993 ), #4309, .F. ) ;
#21942=CYLINDRICAL_SURFACE ( 'NONE', #23724, 27.00000000000000000 ) ;
#21950=CARTESIAN_POINT ( 'NONE',  ( 3.306546357697853733E-15, 210.0000000000000284, 27.00000000000000000 ) ) ;
#21955=CARTESIAN_POINT ( 'NONE',  ( 18.00000000000000355, 246.9250000000000114, 5.196152422706632912 ) ) ;
#21962=CARTESIAN_POINT ( 'NONE',  ( -13.49999999999998401, 197.4875000012290229, 23.38268590217985476 ) ) ;
#21966=CARTESIAN_POINT ( 'NONE',  ( 23.87821517812500005, 245.5093750006145399, 4.985214923628404016 ) ) ;
#21970=EDGE_CURVE ( 'NONE', #32379, #14644, #33495, .T. ) ;
#21975=CARTESIAN_POINT ( 'NONE',  ( -27.24356964375000345, 198.5093750006145399, 0.000000000000000000 ) ) ;
#21979=DIRECTION ( 'NONE',  ( -0.000000000000000000, -1.000000000000000000, -0.000000000000000000 ) ) ;
#21990=CARTESIAN_POINT ( 'NONE',  ( 26.75643035624999655, 240.5593750006145513, -3.323476615752271712 ) ) ;
#21994=CARTESIAN_POINT ( 'NONE',  ( 13.62178482187501416, 198.6593750006145456, 23.59362340125806767 ) ) ;
#21997=CARTESIAN_POINT ( 'NONE',  ( 26.75643035624999655, 241.9468750006145683, 3.323476615752267715 ) ) ;
#22000=ORIENTED_EDGE ( 'NONE', *, *, #27303, .T. ) ;
#22002=CARTESIAN_POINT ( 'NONE',  ( 26.75643035624999655, 244.1218750006145228, -7.049594010296217766E-16 ) ) ;
#22003=LINE ( 'NONE', #37129, #15936 ) ;
#22016=CARTESIAN_POINT ( 'NONE',  ( 15.24356964374999990, 245.6968750006145115, 0.000000000000000000 ) ) ;
#22022=ORIENTED_EDGE ( 'NONE', *, *, #26383, .F. ) ;
#22037=CARTESIAN_POINT ( 'NONE',  ( 27.24356964375000345, 198.2843750006145456, -3.336375036156643733E-15 ) ) ;
#22040=CARTESIAN_POINT ( 'NONE',  ( 20.99999999999999289, 242.2374999999999545, -5.999999999999997335 ) ) ;
#22043=ORIENTED_EDGE ( 'NONE', *, *, #19586, .F. ) ;
#22044=CARTESIAN_POINT ( 'NONE',  ( 23.99999999999999645, 240.4562500012290513, -5.196152422706631135 ) ) ;
#22047=CARTESIAN_POINT ( 'NONE',  ( -13.62178482187500528, 198.3781250006145171, -23.59362340125807123 ) ) ;
#22066=LINE ( 'NONE', #33617, #31663 ) ;
#22070=CARTESIAN_POINT ( 'NONE',  ( -27.99288911131838731, 207.4183503646231941, -7.576574741737489127 ) ) ;
#22075=CARTESIAN_POINT ( 'NONE',  ( 20.99999999999998579, 247.6374999999999886, -5.999999999999997335 ) ) ;
#22076=CARTESIAN_POINT ( 'NONE',  ( 7.234628195640363302, 195.4799038117967029, -26.99999999999996803 ) ) ;
#22077=EDGE_CURVE ( 'NONE', #22146, #11399, #22899, .T. ) ;
#22078=FACE_OUTER_BOUND ( 'NONE', #29860, .T. ) ;
#22080=CARTESIAN_POINT ( 'NONE',  ( 15.24356964374999990, 246.6718750006145342, -3.323476615752268604 ) ) ;
#22082=CARTESIAN_POINT ( 'NONE',  ( 15.24356964374999990, 245.3218750006145399, -3.323476615752268604 ) ) ;
#22083=EDGE_CURVE ( 'NONE', #12855, #15992, #19113, .T. ) ;
#22084=ORIENTED_EDGE ( 'NONE', *, *, #27303, .F. ) ;
#22085=CARTESIAN_POINT ( 'NONE',  ( 19.39230484541326049, 249.5138461906614111, -5.999999999999995559 ) ) ;
#22086=CARTESIAN_POINT ( 'NONE',  ( 26.99999999999999645, 249.3437500012290400, 3.464101615137751278 ) ) ;
#22090=CARTESIAN_POINT ( 'NONE',  ( 22.60769515458672885, 240.7388461906613770, 5.999999999999997335 ) ) ;
#22099=CARTESIAN_POINT ( 'NONE',  ( 20.99999999999999645, 185.0294372515228645, -5.999999999999999112 ) ) ;
#22100=CARTESIAN_POINT ( 'NONE',  ( 15.24356964374999990, 249.2593750006145115, -3.323476615752268604 ) ) ;
#22104=CARTESIAN_POINT ( 'NONE',  ( 14.06542688028853405, 216.9345731196990243, 0.01200585063896637480 ) ) ;
#22106=CARTESIAN_POINT ( 'NONE',  ( 7.234628195640363302, 197.1674038105676914, -26.99999999999996803 ) ) ;
#22111=EDGE_CURVE ( 'NONE', #11470, #3008, #20468, .T. ) ;
#22113=CARTESIAN_POINT ( 'NONE',  ( 13.62178482187499640, 195.1531250006145513, -23.59362340125807123 ) ) ;
#22131=CARTESIAN_POINT ( 'NONE',  ( -7.234628195640316228, 198.6700961906613543, -27.00000000000000000 ) ) ;
#22133=CARTESIAN_POINT ( 'NONE',  ( -27.00000000000000355, 199.0999999999999943, 0.000000000000000000 ) ) ;
#22137=DIRECTION ( 'NONE',  ( -0.000000000000000000, -1.000000000000000000, -0.000000000000000000 ) ) ;
#22142=CARTESIAN_POINT ( 'NONE',  ( 26.99999999999999645, 244.3750000000000000, -7.347880794884117764E-16 ) ) ;
#22146=VERTEX_POINT ( 'NONE', #24411 ) ;
#22148=AXIS2_PLACEMENT_3D ( 'NONE', #23707, #17651, #9302 ) ;
#22149=CARTESIAN_POINT ( 'NONE',  ( -27.00000000000000355, 198.7625000012290286, 0.000000000000000000 ) ) ;
#22150=CARTESIAN_POINT ( 'NONE',  ( 18.00000000000000355, 248.7812500012290400, 5.196152422706632912 ) ) ;
#22153=VECTOR ( 'NONE', #29623, 1000.000000000000000 ) ;
#22154=CARTESIAN_POINT ( 'NONE',  ( 23.87821517812499650, 242.9593750006145285, -4.985214923628404904 ) ) ;
#22155=( BOUNDED_CURVE ( )  B_SPLINE_CURVE ( 2, ( #35273, #9328, #591, #6861, #408, #18436, #11973, #15204, #15582 ),
 .UNSPECIFIED., .F., .F. ) 
 B_SPLINE_CURVE_WITH_KNOTS ( ( 3, 2, 2, 2, 3 ),
 ( 0.1195652173913043653, 0.1231884057971014551, 0.1304347826086956486, 0.1376811594202898559, 0.1413043478260869457 ),
 .UNSPECIFIED. ) 
 CURVE ( )  GEOMETRIC_REPRESENTATION_ITEM ( )  RATIONAL_B_SPLINE_CURVE ( ( 0.9330127018922194093, 0.9330127018922196314, 1.000000000000000000, 0.8660254037844387076, 1.000000000000000000, 0.8660254037844387076, 1.000000000000000000, 0.9330127018922196314, 0.9330127018922194093 ) ) 
 REPRESENTATION_ITEM ( '' )  );
#22157=EDGE_CURVE ( 'NONE', #21280, #149, #17371, .T. ) ;
#22162=CARTESIAN_POINT ( 'NONE',  ( -27.24356964375000345, 198.9593750006145285, 0.000000000000000000 ) ) ;
#22166=CARTESIAN_POINT ( 'NONE',  ( -4.500000000000000888, 210.0000000000000000, 0.000000000000000000 ) ) ;
#22174=CIRCLE ( 'NONE', #35459, 8.000000000000000000 ) ;
#22176=CARTESIAN_POINT ( 'NONE',  ( 23.99999999999999645, 248.5562500012290457, -5.196152422706631135 ) ) ;
#22180=CARTESIAN_POINT ( 'NONE',  ( 13.62178482187499640, 197.9093750006145456, -23.59362340125807123 ) ) ;
#22181=DIRECTION ( 'NONE',  ( -1.000000000000000000, 0.000000000000000000, -0.000000000000000000 ) ) ;
#22183=DIRECTION ( 'NONE',  ( 0.000000000000000000, 0.000000000000000000, -1.000000000000000000 ) ) ;
#22184=CARTESIAN_POINT ( 'NONE',  ( 18.12178482187500350, 242.2843750006145456, 4.985214923628407568 ) ) ;
#22191=CARTESIAN_POINT ( 'NONE',  ( 18.12178482187499640, 244.7218750006145171, -4.985214923628404904 ) ) ;
#22193=CARTESIAN_POINT ( 'NONE',  ( 3.306546357697853733E-15, 210.0000000000000284, 27.00000000000000000 ) ) ;
#22196=CARTESIAN_POINT ( 'NONE',  ( 22.60769515458672885, 244.2825961894323541, 5.999999999999997335 ) ) ;
#22199=ORIENTED_EDGE ( 'NONE', *, *, #2054, .T. ) ;
#22204=CARTESIAN_POINT ( 'NONE',  ( 26.75643035624999655, 243.1843750006145513, 3.323476615752267271 ) ) ;
#22205=CARTESIAN_POINT ( 'NONE',  ( -27.00000000000000355, 197.3750000012290400, -15.58845726811989429 ) ) ;
#22223=CARTESIAN_POINT ( 'NONE',  ( 27.24356964375000700, 197.7968750006145342, 15.72908226750537075 ) ) ;
#22225=EDGE_CURVE ( 'NONE', #31527, #7301, #8387, .T. ) ;
#22229=ORIENTED_EDGE ( 'NONE', *, *, #17031, .T. ) ;
#22230=VECTOR ( 'NONE', #9937, 1000.000000000000000 ) ;
#22231=CARTESIAN_POINT ( 'NONE',  ( 18.00000000000000355, 241.5812500012290513, 5.196152422706632912 ) ) ;
#22234=CARTESIAN_POINT ( 'NONE',  ( 13.62178482187499640, 198.3031250006145285, -23.59362340125807123 ) ) ;
#22245=CARTESIAN_POINT ( 'NONE',  ( -13.50000000000000533, 196.3249999999999886, -23.38268590217984411 ) ) ;
#22258=CARTESIAN_POINT ( 'NONE',  ( 18.00000000000000355, 244.2812500012290400, 5.196152422706632912 ) ) ;
#22259=ORIENTED_EDGE ( 'NONE', *, *, #18430, .F. ) ;
#22266=CARTESIAN_POINT ( 'NONE',  ( 26.75643035624999655, 248.6968750006145115, 3.323476615752267715 ) ) ;
#22268=CARTESIAN_POINT ( 'NONE',  ( 26.75643035624999655, 240.6343750006145115, -7.049594010296217766E-16 ) ) ;
#22272=CARTESIAN_POINT ( 'NONE',  ( 26.99999999999999645, 248.0312500012290400, -7.347880794884117764E-16 ) ) ;
#22280=ORIENTED_EDGE ( 'NONE', *, *, #17949, .F. ) ;
#22285=CARTESIAN_POINT ( 'NONE',  ( 15.24356964375000167, 248.8843750006145399, 3.323476615752272600 ) ) ;
#22288=CARTESIAN_POINT ( 'NONE',  ( 6.017554903305191161, 215.6184169112603968, 2.114697272285289475 ) ) ;
#22296=CARTESIAN_POINT ( 'NONE',  ( 13.62178482187501416, 195.9031250006145513, 23.59362340125806767 ) ) ;
#22310=CARTESIAN_POINT ( 'NONE',  ( 0.000000000000000000, 210.0000000000000284, 0.000000000000000000 ) ) ;
#22314=CARTESIAN_POINT ( 'NONE',  ( -13.49999999999998401, 196.9250000000000114, 23.38268590217985476 ) ) ;
#22315=CARTESIAN_POINT ( 'NONE',  ( 20.99999999999999645, 185.0294372515228645, -5.999999999999999112 ) ) ;
#22318=CARTESIAN_POINT ( 'NONE',  ( 18.00000000000000000, 241.8250000000000171, -5.196152422706630247 ) ) ;
#22319=ORIENTED_EDGE ( 'NONE', *, *, #27087, .T. ) ;
#22325=CARTESIAN_POINT ( 'NONE',  ( 18.00000000000000355, 242.4250000000000114, 5.196152422706632912 ) ) ;
#22331=CARTESIAN_POINT ( 'NONE',  ( 13.50000000000001421, 197.1125000012290513, 23.38268590217984055 ) ) ;
#22335=CARTESIAN_POINT ( 'NONE',  ( 18.12178482187500350, 242.2843750006145456, 4.985214923628407568 ) ) ;
#22337=CARTESIAN_POINT ( 'NONE',  ( -27.00000000000000355, 199.6625000012290343, 0.000000000000000000 ) ) ;
#22342=CARTESIAN_POINT ( 'NONE',  ( -27.24356964374999635, 197.6468750006145285, 15.72908226750539384 ) ) ;
#22359=CARTESIAN_POINT ( 'NONE',  ( 10.49999999999999467, 215.7563705986615901, 5.555555555555558911 ) ) ;
#22364=CARTESIAN_POINT ( 'NONE',  ( 27.24356964374999279, 197.4218750006145342, -15.72908226750539207 ) ) ;
#22368=CARTESIAN_POINT ( 'NONE',  ( 18.12178482187500350, 240.9343750006145513, 4.985214923628407568 ) ) ;
#22375=CARTESIAN_POINT ( 'NONE',  ( 23.87821517812499650, 245.0968750006145171, -4.985214923628404904 ) ) ;
#22379=CARTESIAN_POINT ( 'NONE',  ( 20.99999999999999289, 244.4874999999999829, -5.999999999999997335 ) ) ;
#22386=CARTESIAN_POINT ( 'NONE',  ( 18.12178482187500350, 244.8718750006145228, 4.985214923628407568 ) ) ;
#22387=ADVANCED_FACE ( 'NONE', ( #17506 ), #32650, .F. ) ;
#22391=EDGE_CURVE ( 'NONE', #4778, #20196, #50, .T. ) ;
#22397=CARTESIAN_POINT ( 'NONE',  ( 26.99999999999999645, 242.6687500012290570, -3.464101615137755275 ) ) ;
#22402=CARTESIAN_POINT ( 'NONE',  ( 20.99999999999999645, 248.7624999999999886, 5.999999999999998224 ) ) ;
#22405=EDGE_CURVE ( 'NONE', #10385, #16763, #29041, .T. ) ;
#22408=CARTESIAN_POINT ( 'NONE',  ( -13.62178482187500528, 197.5343750006145456, -23.59362340125807123 ) ) ;
#22409=CARTESIAN_POINT ( 'NONE',  ( 19.39230484541326049, 249.9075961894323541, -5.999999999999997335 ) ) ;
#22414=CARTESIAN_POINT ( 'NONE',  ( 21.00000000000000000, 242.2937500012290570, -6.928203230275506996 ) ) ;
#22433=CARTESIAN_POINT ( 'NONE',  ( -14.08244204927778576, 215.9517727336253756, -5.357269300704888160 ) ) ;
#22442=EDGE_LOOP ( 'NONE', ( #22084, #28993, #32882, #24652 ) ) ;
#22447=LINE ( 'NONE', #19246, #32327 ) ;
#22448=DIRECTION ( 'NONE',  ( -0.000000000000000000, 1.000000000000000000, -0.000000000000000000 ) ) ;
#22449=CARTESIAN_POINT ( 'NONE',  ( 19.39230484541326760, 247.8424038105676459, 5.999999999999999112 ) ) ;
#22450=CARTESIAN_POINT ( 'NONE',  ( 23.87821517812500005, 247.7593750006145399, 4.985214923628404016 ) ) ;
#22452=CARTESIAN_POINT ( 'NONE',  ( 18.12178482187500350, 242.2843750006145456, 4.985214923628407568 ) ) ;
#22456=CARTESIAN_POINT ( 'NONE',  ( 26.99999999999999645, 247.5812500012290513, -7.347880794884117764E-16 ) ) ;
#22462=ORIENTED_EDGE ( 'NONE', *, *, #15902, .T. ) ;
#22463=EDGE_LOOP ( 'NONE', ( #25819, #15371, #25985, #6271 ) ) ;
#22468=CYLINDRICAL_SURFACE ( 'NONE', #28695, 5.999999999999999112 ) ;
#22469=CARTESIAN_POINT ( 'NONE',  ( 21.00000000000000000, 248.0593750006145228, 6.646953231504538984 ) ) ;
#22473=CARTESIAN_POINT ( 'NONE',  ( 14.34881165084055965, 216.6511883491515675, -0.6450403596498489600 ) ) ;
#22476=ADVANCED_FACE ( 'NONE', ( #25008 ), #21301, .F. ) ;
#22486=CARTESIAN_POINT ( 'NONE',  ( -27.24356964374999990, 195.7156250006145513, -15.72908226750537786 ) ) ;
#22489=ORIENTED_EDGE ( 'NONE', *, *, #27094, .F. ) ;
#22500=CARTESIAN_POINT ( 'NONE',  ( 19.39230484541326760, 249.1924038105676686, 5.999999999999998224 ) ) ;
#22502=CARTESIAN_POINT ( 'NONE',  ( 13.50000000000001421, 198.8000000000000114, 23.38268590217984055 ) ) ;
#22506=CARTESIAN_POINT ( 'NONE',  ( 23.87821517812500005, 249.5593750006145228, 4.985214923628404016 ) ) ;
#22513=CARTESIAN_POINT ( 'NONE',  ( 15.00000000000000000, 243.6999999999999886, 0.000000000000000000 ) ) ;
#22517=VERTEX_POINT ( 'NONE', #10605 ) ;
#22519=CARTESIAN_POINT ( 'NONE',  ( 26.99999999999999645, 195.8750000012290400, -15.58845726811990495 ) ) ;
#22523=CARTESIAN_POINT ( 'NONE',  ( 26.75643035624999655, 242.8843750006145115, -7.049594010296217766E-16 ) ) ;
#22529=CARTESIAN_POINT ( 'NONE',  ( -27.24356964374999990, 198.0218750006145569, -15.72908226750537786 ) ) ;
#22534=CARTESIAN_POINT ( 'NONE',  ( 20.99999999999999645, 185.0294372515228645, 5.999999999999999112 ) ) ;
#22539=CARTESIAN_POINT ( 'NONE',  ( 20.99999999999998579, 247.2437500012290457, -5.999999999999997335 ) ) ;
#22547=CARTESIAN_POINT ( 'NONE',  ( -13.62178482187498396, 197.2343750006145626, 23.59362340125808188 ) ) ;
#22550=FACE_OUTER_BOUND ( 'NONE', #24959, .T. ) ;
#22551=CARTESIAN_POINT ( 'NONE',  ( 18.00000000000000000, 249.9250000000000114, -5.196152422706630247 ) ) ;
#22552=CARTESIAN_POINT ( 'NONE',  ( -27.24356964375000345, 199.8031250006145285, 0.000000000000000000 ) ) ;
#22557=VERTEX_POINT ( 'NONE', #35677 ) ;
#22558=CARTESIAN_POINT ( 'NONE',  ( 18.12178482187499640, 243.8218750006145399, -4.985214923628404904 ) ) ;
#22572=CARTESIAN_POINT ( 'NONE',  ( 20.99999999999999645, 244.6843750006145513, -6.646953231504538984 ) ) ;
#22580=CARTESIAN_POINT ( 'NONE',  ( 1.255007937094097924E-14, 199.4375000000000284, -27.00000000000000000 ) ) ;
#22585=AXIS2_PLACEMENT_3D ( 'NONE', #10405, #33525, #7567 ) ;
#22594=CARTESIAN_POINT ( 'NONE',  ( 20.99999999999997513, 246.7937500012290286, -5.999999999999999112 ) ) ;
#22595=CARTESIAN_POINT ( 'NONE',  ( -13.62178482187498396, 195.4343750006145228, 23.59362340125808188 ) ) ;
#22596=CARTESIAN_POINT ( 'NONE',  ( 18.00000000000000000, 249.9250000000000114, -5.196152422706630247 ) ) ;
#22602=CARTESIAN_POINT ( 'NONE',  ( 21.00000000000000000, 242.5187500012290513, 6.928203230275506996 ) ) ;
#22614=ADVANCED_FACE ( 'NONE', ( #32837 ), #6882, .T. ) ;
#22616=B_SPLINE_CURVE_WITH_KNOTS ( 'NONE', 3,
 ( #27370, #33810, #13158, #30220, #7662, #22070, #25085, #36640, #24713, #18861, #35894, #4245, #30409, #24533, #4804, #4432, #16013, #1590, #21880, #33621, #19239, #30781, #16384, #27928 ),
 .UNSPECIFIED., .F., .F.,
 ( 4, 2, 2, 2, 2, 2, 2, 2, 2, 2, 2, 4 ),
 ( 0.000000000000000000, 0.001571281823982130250, 0.002356922735973196025, 0.003142563647964261367, 0.004713845471946314855, 0.005499486383937341599, 0.006285127295928367476, 0.007856409119910477343, 0.009427690943892588077, 0.01021333185588364431, 0.01099897276787470055, 0.01257025459185682689 ),
 .UNSPECIFIED. ) ;
#22620=CARTESIAN_POINT ( 'NONE',  ( -27.00000000000000355, 197.8625000012290513, 0.000000000000000000 ) ) ;
#22621=CARTESIAN_POINT ( 'NONE',  ( -4.694659320240884604E-14, 197.5250000012290172, 27.00000000000000000 ) ) ;
#22632=DIRECTION ( 'NONE',  ( -0.000000000000000000, 1.000000000000000000, -0.000000000000000000 ) ) ;
#22638=CARTESIAN_POINT ( 'NONE',  ( 18.12178482187500350, 248.1343750006145399, 4.985214923628407568 ) ) ;
#22640=CARTESIAN_POINT ( 'NONE',  ( 20.99999999999999645, 242.0968750006145456, -6.646953231504538984 ) ) ;
#22643=DIRECTION ( 'NONE',  ( -0.000000000000000000, 1.000000000000000000, -0.000000000000000000 ) ) ;
#22644=CARTESIAN_POINT ( 'NONE',  ( 18.00000000000000355, 248.3312500012290513, 5.196152422706632912 ) ) ;
#22649=CARTESIAN_POINT ( 'NONE',  ( 20.99999999999995026, 240.9437500012290911, -5.999999999999998224 ) ) ;
#22660=CARTESIAN_POINT ( 'NONE',  ( 21.00000000000000000, 249.1843750006144944, -6.646953231504538984 ) ) ;
#22662=AXIS2_PLACEMENT_3D ( 'NONE', #13942, #5210, #36858 ) ;
#22665=CARTESIAN_POINT ( 'NONE',  ( 14.43174379454687362, 216.5682562054521725, 0.6968546016497486617 ) ) ;
#22672=CARTESIAN_POINT ( 'NONE',  ( 27.24356964375000700, 195.0406250006145399, 15.72908226750537075 ) ) ;
#22675=ORIENTED_EDGE ( 'NONE', *, *, #24434, .T. ) ;
#22677=CARTESIAN_POINT ( 'NONE',  ( 23.99999999999999645, 249.0062500012290627, -5.196152422706631135 ) ) ;
#22687=DIRECTION ( 'NONE',  ( -0.000000000000000000, 1.000000000000000000, -0.000000000000000000 ) ) ;
#22689=CARTESIAN_POINT ( 'NONE',  ( 18.00000000000000000, 243.2312500012290570, -5.196152422706630247 ) ) ;
#22691=CARTESIAN_POINT ( 'NONE',  ( 27.00000000000001066, 197.9375000000000284, 15.58845726811988897 ) ) ;
#22695=CARTESIAN_POINT ( 'NONE',  ( 26.75643035624999655, 249.6718750006145342, -3.323476615752271268 ) ) ;
#22696=ORIENTED_EDGE ( 'NONE', *, *, #6911, .T. ) ;
#22698=CARTESIAN_POINT ( 'NONE',  ( 10.49999999999999467, 210.0000000000000000, 0.000000000000000000 ) ) ;
#22699=ADVANCED_FACE ( 'NONE', ( #33545 ), #7959, .F. ) ;
#22703=CARTESIAN_POINT ( 'NONE',  ( 18.00000000000000000, 244.0749999999999886, -5.196152422706630247 ) ) ;
#22704=CARTESIAN_POINT ( 'NONE',  ( -13.49999999999998401, 198.7250000000000227, 23.38268590217985476 ) ) ;
#22705=EDGE_CURVE ( 'NONE', #35917, #20737, #31840, .T. ) ;
#22706=( BOUNDED_CURVE ( )  B_SPLINE_CURVE ( 2, ( #28325, #16964, #9126, #576, #17664, #13754, #20692, #9315, #29200 ),
 .UNSPECIFIED., .F., .F. ) 
 B_SPLINE_CURVE_WITH_KNOTS ( ( 3, 2, 2, 2, 3 ),
 ( 0.1847826086956521618, 0.1884057971014492794, 0.1956521739130434867, 0.2028985507246376940, 0.2065217391304347838 ),
 .UNSPECIFIED. ) 
 CURVE ( )  GEOMETRIC_REPRESENTATION_ITEM ( )  RATIONAL_B_SPLINE_CURVE ( ( 0.9330127018922194093, 0.9330127018922190762, 1.000000000000000000, 0.8660254037844387076, 1.000000000000000000, 0.8660254037844387076, 1.000000000000000000, 0.9330127018922194093, 0.9330127018922194093 ) ) 
 REPRESENTATION_ITEM ( '' )  );
#22710=CARTESIAN_POINT ( 'NONE',  ( 5.727106289114498080E-15, 194.8250000012290570, 31.17691453623979214 ) ) ;
#22714=CARTESIAN_POINT ( 'NONE',  ( 15.24356964375000167, 241.7968750006145342, 3.323476615752272600 ) ) ;
#22721=CARTESIAN_POINT ( 'NONE',  ( 13.62178482187499640, 197.4593750006145285, -23.59362340125807123 ) ) ;
#22732=CARTESIAN_POINT ( 'NONE',  ( 15.65448942698881574, 195.0065153083762652, -22.13879085154164628 ) ) ;
#22733=CARTESIAN_POINT ( 'NONE',  ( 20.99999999999999645, 185.0294372515228645, -5.999999999999999112 ) ) ;
#22737=CARTESIAN_POINT ( 'NONE',  ( -1.926257025242585782E-15, 196.1468750006145569, -31.45816453501076637 ) ) ;
#22740=CARTESIAN_POINT ( 'NONE',  ( -7.234628195640289583, 198.1075961894323143, -27.00000000000001421 ) ) ;
#22741=CARTESIAN_POINT ( 'NONE',  ( 15.24356964374999990, 241.3093750006145228, 0.000000000000000000 ) ) ;
#22742=CARTESIAN_POINT ( 'NONE',  ( -13.62178482187498396, 199.4281250006145569, 23.59362340125808188 ) ) ;
#22748=CARTESIAN_POINT ( 'NONE',  ( 18.12178482187500350, 241.2718750006145001, 4.985214923628407568 ) ) ;
#22757=CARTESIAN_POINT ( 'NONE',  ( 26.75643035624999655, 243.2218750006145171, -7.049594010296217766E-16 ) ) ;
#22764=FACE_OUTER_BOUND ( 'NONE', #32756, .T. ) ;
#22776=CARTESIAN_POINT ( 'NONE',  ( 20.99999999999995026, 241.3375000000000341, -5.999999999999998224 ) ) ;
#22778=CARTESIAN_POINT ( 'NONE',  ( -27.24356964375000345, 196.7093750006145569, 0.000000000000000000 ) ) ;
#22779=CARTESIAN_POINT ( 'NONE',  ( 6.753460448932012028, 195.0000000000000284, 26.40771703998824549 ) ) ;
#22780=CARTESIAN_POINT ( 'NONE',  ( -7.234628195640328663, 197.0549038117967484, 26.99999999999999289 ) ) ;
#22784=CARTESIAN_POINT ( 'NONE',  ( 26.99999999999999645, 240.8312500012290513, -7.347880794884117764E-16 ) ) ;
#22790=ORIENTED_EDGE ( 'NONE', *, *, #29328, .T. ) ;
#22796=AXIS2_PLACEMENT_3D ( 'NONE', #6005, #17587, #29119 ) ;
#22802=VERTEX_POINT ( 'NONE', #13798 ) ;
#22812=VERTEX_POINT ( 'NONE', #2216 ) ;
#22819=CARTESIAN_POINT ( 'NONE',  ( 23.99999999999999645, 246.3062500012290457, -5.196152422706631135 ) ) ;
#22820=CARTESIAN_POINT ( 'NONE',  ( 26.75643035624999655, 244.2718750006145001, -3.323476615752271712 ) ) ;
#22822=CARTESIAN_POINT ( 'NONE',  ( 26.75643035624999655, 241.5343750006145456, -7.049594010296217766E-16 ) ) ;
#22827=EDGE_CURVE ( 'NONE', #5728, #6033, #7547, .T. ) ;
#22828=CARTESIAN_POINT ( 'NONE',  ( 21.00000000000000000, 247.6937500012290343, -6.928203230275506996 ) ) ;
#22842=DIRECTION ( 'NONE',  ( -0.000000000000000000, 1.000000000000000000, -0.000000000000000000 ) ) ;
#22843=CARTESIAN_POINT ( 'NONE',  ( 18.12178482187499640, 248.7718750006145001, -4.985214923628404904 ) ) ;
#22846=CARTESIAN_POINT ( 'NONE',  ( 5.840947329779441866, 215.6846447513326268, 1.929602858956334099 ) ) ;
#22870=CARTESIAN_POINT ( 'NONE',  ( -13.50000000000000533, 197.2250000000000227, -23.38268590217984411 ) ) ;
#22873=CARTESIAN_POINT ( 'NONE',  ( 18.12178482187499640, 248.4343750006145228, -4.985214923628404904 ) ) ;
#22880=CARTESIAN_POINT ( 'NONE',  ( 26.99999999999999645, 244.3375000000000341, 3.464101615137751278 ) ) ;
#22884=VERTEX_POINT ( 'NONE', #21770 ) ;
#22886=CARTESIAN_POINT ( 'NONE',  ( -27.00000000000000355, 196.4750000012290343, -15.58845726811989429 ) ) ;
#22887=CARTESIAN_POINT ( 'NONE',  ( -7.234628195640263826, 196.4200961906613543, -27.00000000000003553 ) ) ;
#22892=CARTESIAN_POINT ( 'NONE',  ( 21.00000000000000000, 243.2218750006145456, 6.646953231504538984 ) ) ;
#22895=CARTESIAN_POINT ( 'NONE',  ( 18.00000000000000355, 242.9312500012290457, 5.196152422706632912 ) ) ;
#22899=( BOUNDED_CURVE ( )  B_SPLINE_CURVE ( 2, ( #24594, #1840, #33683, #19306, #13229, #10745, #22318, #10187, #15888 ),
 .UNSPECIFIED., .F., .F. ) 
 B_SPLINE_CURVE_WITH_KNOTS ( ( 3, 2, 2, 2, 3 ),
 ( 0.7717391304347825942, 0.7753623188405797118, 0.7826086956521739468, 0.7898550724637680709, 0.7934782608695651884 ),
 .UNSPECIFIED. ) 
 CURVE ( )  GEOMETRIC_REPRESENTATION_ITEM ( )  RATIONAL_B_SPLINE_CURVE ( ( 0.9330127018922194093, 0.9330127018922194093, 1.000000000000000000, 0.8660254037844387076, 1.000000000000000000, 0.8660254037844387076, 1.000000000000000000, 0.9330127018922194093, 0.9330127018922194093 ) ) 
 REPRESENTATION_ITEM ( '' )  );
#22901=CARTESIAN_POINT ( 'NONE',  ( -27.24356964374999635, 195.3968750006145569, 15.72908226750539384 ) ) ;
#22903=EDGE_CURVE ( 'NONE', #6033, #717, #37219, .T. ) ;
#22906=CARTESIAN_POINT ( 'NONE',  ( 18.00000000000000000, 240.4749999999999943, -5.196152422706630247 ) ) ;
#22907=CARTESIAN_POINT ( 'NONE',  ( 26.99999999999999645, 245.2750000000000057, -7.347880794884117764E-16 ) ) ;
#22923=CARTESIAN_POINT ( 'NONE',  ( 13.49999999999999645, 196.2500000000000000, -23.38268590217984766 ) ) ;
#22927=CARTESIAN_POINT ( 'NONE',  ( 18.12178482187500350, 241.3843750006145115, 4.985214923628407568 ) ) ;
#22928=CARTESIAN_POINT ( 'NONE',  ( -27.24356964375000345, 198.4531250006145342, 0.000000000000000000 ) ) ;
#22931=EDGE_LOOP ( 'NONE', ( #4259, #9494 ) ) ;
#22932=ORIENTED_EDGE ( 'NONE', *, *, #776, .T. ) ;
#22933=CARTESIAN_POINT ( 'NONE',  ( -1.926257025242585782E-15, 197.8906250006145342, -31.45816453501075927 ) ) ;
#22934=CARTESIAN_POINT ( 'NONE',  ( 18.12178482187500350, 241.7218750006145171, 4.985214923628407568 ) ) ;
#22939=CIRCLE ( 'NONE', #19916, 27.00000000000000000 ) ;
#22944=CARTESIAN_POINT ( 'NONE',  ( 23.87821517812500005, 244.4968750006145228, 4.985214923628404016 ) ) ;
#22945=CARTESIAN_POINT ( 'NONE',  ( 26.99999999999999645, 246.7187500012290684, -3.464101615137755275 ) ) ;
#22957=CARTESIAN_POINT ( 'NONE',  ( 26.99999999999999645, 245.7437500012290457, 3.464101615137751278 ) ) ;
#22964=CARTESIAN_POINT ( 'NONE',  ( 5.778771075727756162E-15, 195.9218750006145342, 31.45816453501075927 ) ) ;
#22965=LINE ( 'NONE', #11576, #29534 ) ;
#22966=CARTESIAN_POINT ( 'NONE',  ( 20.99999999999999645, 185.0294372515228645, 5.999999999999999112 ) ) ;
#22971=CARTESIAN_POINT ( 'NONE',  ( 21.00000000000000000, 248.7343750006145342, -6.646953231504538984 ) ) ;
#22982=CARTESIAN_POINT ( 'NONE',  ( -25.62253007092369117, 194.9999999999999716, 8.926458104496534318 ) ) ;
#22987=CARTESIAN_POINT ( 'NONE',  ( -28.72218192485006227, 203.0733802275103983, 4.011256465603768362 ) ) ;
#23000=CARTESIAN_POINT ( 'NONE',  ( 7.234628195640309123, 197.6174038105676516, -27.00000000000000711 ) ) ;
#23002=CARTESIAN_POINT ( 'NONE',  ( 18.12178482187499640, 245.7343750006145342, -4.985214923628404904 ) ) ;
#23004=CARTESIAN_POINT ( 'NONE',  ( 15.24356964375000167, 240.8968750006145001, 3.323476615752272600 ) ) ;
#23005=VERTEX_POINT ( 'NONE', #28185 ) ;
#23008=CARTESIAN_POINT ( 'NONE',  ( 24.00000000000000000, 247.5062500012290627, 5.196152422706629359 ) ) ;
#23017=VERTEX_POINT ( 'NONE', #4876 ) ;
#23024=CARTESIAN_POINT ( 'NONE',  ( 18.12178482187499640, 245.6218750006145228, -4.985214923628404904 ) ) ;
#23027=CARTESIAN_POINT ( 'NONE',  ( 21.00000000000003553, 209.9999999999999716, -5.999999999999996447 ) ) ;
#23037=CARTESIAN_POINT ( 'NONE',  ( 5.778771075727756162E-15, 194.9656250006145228, 31.45816453501075927 ) ) ;
#23044=EDGE_CURVE ( 'NONE', #253, #1148, #24335, .T. ) ;
#23053=CARTESIAN_POINT ( 'NONE',  ( -13.50000000000000533, 199.0250000000000057, -23.38268590217984411 ) ) ;
#23056=CARTESIAN_POINT ( 'NONE',  ( 15.24356964374999990, 248.4718750006144603, -3.323476615752268604 ) ) ;
#23057=ORIENTED_EDGE ( 'NONE', *, *, #34267, .T. ) ;
#23059=CARTESIAN_POINT ( 'NONE',  ( 26.99999999999999645, 243.4749999999999943, -7.347880794884117764E-16 ) ) ;
#23063=CARTESIAN_POINT ( 'NONE',  ( 15.00000000000000000, 241.8625000000000114, -3.464101615137752166 ) ) ;
#23066=VERTEX_POINT ( 'NONE', #37266 ) ;
#23068=CARTESIAN_POINT ( 'NONE',  ( -13.49999999999998401, 196.5875000012290457, 23.38268590217985476 ) ) ;
#23073=CARTESIAN_POINT ( 'NONE',  ( 26.75643035624999655, 241.5718750006145115, -3.323476615752271712 ) ) ;
#23083=CARTESIAN_POINT ( 'NONE',  ( 27.24356964374999635, 195.1718750006145342, -15.72908226750539029 ) ) ;
#23088=CARTESIAN_POINT ( 'NONE',  ( 20.99999999999999289, 240.4374999999999716, -5.999999999999997335 ) ) ;
#23089=LINE ( 'NONE', #34633, #37435 ) ;
#23099=CARTESIAN_POINT ( 'NONE',  ( 24.00000000000000000, 249.7000000000000171, 5.196152422706629359 ) ) ;
#23100=CARTESIAN_POINT ( 'NONE',  ( -27.00000000000000355, 195.1250000012290400, -15.58845726811989429 ) ) ;
#23104=CARTESIAN_POINT ( 'NONE',  ( 27.24356964375000345, 195.5843750006145285, -3.336375036156643733E-15 ) ) ;
#23108=CARTESIAN_POINT ( 'NONE',  ( 19.00081571707362116, 239.8729221881839351, -5.492723647597327563 ) ) ;
#23109=CARTESIAN_POINT ( 'NONE',  ( 27.24356964375000345, 198.2281250006145399, -3.336375036156643733E-15 ) ) ;
#23114=ORIENTED_EDGE ( 'NONE', *, *, #37125, .T. ) ;
#23115=CARTESIAN_POINT ( 'NONE',  ( -27.24356964375000345, 197.1031250006145399, 0.000000000000000000 ) ) ;
#23116=CARTESIAN_POINT ( 'NONE',  ( 26.75643035624999655, 242.2843750006145171, 3.323476615752267715 ) ) ;
#23120=( BOUNDED_CURVE ( )  B_SPLINE_CURVE ( 2, ( #9523, #6866, #12165, #4014, #35277, #26758, #27329, #32444, #1358 ),
 .UNSPECIFIED., .F., .F. ) 
 B_SPLINE_CURVE_WITH_KNOTS ( ( 3, 2, 2, 2, 3 ),
 ( 0.2934782608695652439, 0.2971014492753623060, 0.3043478260869565410, 0.3115942028985507206, 0.3152173913043477826 ),
 .UNSPECIFIED. ) 
 CURVE ( )  GEOMETRIC_REPRESENTATION_ITEM ( )  RATIONAL_B_SPLINE_CURVE ( ( 0.9330127018922194093, 0.9330127018922198534, 1.000000000000000000, 0.8660254037844387076, 1.000000000000000000, 0.8660254037844387076, 1.000000000000000000, 0.9330127018922198534, 0.9330127018922191873 ) ) 
 REPRESENTATION_ITEM ( '' )  );
#23125=CARTESIAN_POINT ( 'NONE',  ( 26.75643035624999655, 242.2843750006145456, 3.323476615752267271 ) ) ;
#23135=CARTESIAN_POINT ( 'NONE',  ( -13.49999999999998401, 198.8375000012290457, 23.38268590217985476 ) ) ;
#23142=CARTESIAN_POINT ( 'NONE',  ( 21.00000000000000000, 243.1093750006145058, 6.646953231504538984 ) ) ;
#23146=CARTESIAN_POINT ( 'NONE',  ( 26.99999999999999645, 244.0187500012290513, -3.464101615137755275 ) ) ;
#23147=CARTESIAN_POINT ( 'NONE',  ( 26.99999999999999645, 241.2249999999999943, -7.347880794884117764E-16 ) ) ;
#23150=CARTESIAN_POINT ( 'NONE',  ( 27.24356964375000700, 195.5468750006145342, 15.72908226750537075 ) ) ;
#23151=CARTESIAN_POINT ( 'NONE',  ( 20.99999999999997513, 246.2874999999999943, -5.999999999999999112 ) ) ;
#23155=ORIENTED_EDGE ( 'NONE', *, *, #22405, .F. ) ;
#23157=CARTESIAN_POINT ( 'NONE',  ( 23.87821517812500005, 249.4468750006145115, 4.985214923628404016 ) ) ;
#23168=CARTESIAN_POINT ( 'NONE',  ( 26.75643035624999655, 248.1343750006145399, 3.323476615752267271 ) ) ;
#23169=CARTESIAN_POINT ( 'NONE',  ( -12.09976244894570563, 194.9999999999999432, 24.41260623486415682 ) ) ;
#23181=ORIENTED_EDGE ( 'NONE', *, *, #21864, .F. ) ;
#23187=CARTESIAN_POINT ( 'NONE',  ( 13.50000000000001421, 196.2125000012290172, 23.38268590217984055 ) ) ;
#23188=DIRECTION ( 'NONE',  ( -0.000000000000000000, 1.000000000000000000, -0.000000000000000000 ) ) ;
#23190=CARTESIAN_POINT ( 'NONE',  ( 21.00000000000000000, 245.9218750006145058, 6.646953231504538984 ) ) ;
#23196=CARTESIAN_POINT ( 'NONE',  ( 15.00000000000000000, 245.9687500012290684, -3.464101615137752166 ) ) ;
#23197=VERTEX_POINT ( 'NONE', #28547 ) ;
#23200=CARTESIAN_POINT ( 'NONE',  ( 7.234628195640322446, 197.9950961906613429, 26.99999999999999645 ) ) ;
#23204=ORIENTED_EDGE ( 'NONE', *, *, #24532, .F. ) ;
#23205=ORIENTED_EDGE ( 'NONE', *, *, #11687, .T. ) ;
#23206=ORIENTED_EDGE ( 'NONE', *, *, #14077, .F. ) ;
#23209=CARTESIAN_POINT ( 'NONE',  ( 21.00000000000000000, 246.7093750006145285, 6.646953231504538984 ) ) ;
#23213=CARTESIAN_POINT ( 'NONE',  ( 19.44430458907289605, 214.1485210958233836, -5.808099892140725196 ) ) ;
#23221=CARTESIAN_POINT ( 'NONE',  ( -20.86978604919638869, 194.8026013911397740, -17.51182792271053046 ) ) ;
#23228=CARTESIAN_POINT ( 'NONE',  ( 19.98630977700905831, 239.7005235349005829, -5.748934002787875919 ) ) ;
#23233=LINE ( 'NONE', #9009, #8584 ) ;
#23237=CARTESIAN_POINT ( 'NONE',  ( 5.778771075727756162E-15, 199.5218750006145854, 31.45816453501075927 ) ) ;
#23240=CARTESIAN_POINT ( 'NONE',  ( 20.99999999999999645, 248.8468750006145456, -6.646953231504538984 ) ) ;
#23249=CARTESIAN_POINT ( 'NONE',  ( 15.00000000000000000, 242.3125000000000000, -3.464101615137752166 ) ) ;
#23256=CARTESIAN_POINT ( 'NONE',  ( -27.00000000000000355, 195.1625000012290343, 0.000000000000000000 ) ) ;
#23261=CARTESIAN_POINT ( 'NONE',  ( 26.75643035624999655, 240.2218750006145171, -3.323476615752271712 ) ) ;
#23263=CARTESIAN_POINT ( 'NONE',  ( 20.99999999999995026, 242.7437500012290741, -5.999999999999998224 ) ) ;
#23269=CARTESIAN_POINT ( 'NONE',  ( -1.926257025242585782E-15, 197.0468750006145626, -31.45816453501075927 ) ) ;
#23277=CARTESIAN_POINT ( 'NONE',  ( 20.99999999999997513, 247.1875000000000284, -5.999999999999999112 ) ) ;
#23284=CARTESIAN_POINT ( 'NONE',  ( 21.00000000000000000, 245.6125000000000114, 5.999999999999998224 ) ) ;
#23291=CARTESIAN_POINT ( 'NONE',  ( 27.24356964375000700, 195.9968750006145513, 15.72908226750537075 ) ) ;
#23295=CARTESIAN_POINT ( 'NONE',  ( 15.00000000000000000, 247.2624999999999886, -3.464101615137752166 ) ) ;
#23296=CARTESIAN_POINT ( 'NONE',  ( 27.24356964375000345, 197.7781250006145228, -3.336375036156643733E-15 ) ) ;
#23301=CARTESIAN_POINT ( 'NONE',  ( -13.62178482187500528, 197.0281250006145228, -23.59362340125807123 ) ) ;
#23302=CARTESIAN_POINT ( 'NONE',  ( 26.75643035624999655, 243.2593750006145115, -3.323476615752271712 ) ) ;
#23303=EDGE_CURVE ( 'NONE', #33968, #24114, #11032, .T. ) ;
#23306=CARTESIAN_POINT ( 'NONE',  ( 26.75643035624999655, 246.9343750006145228, -7.049594010296217766E-16 ) ) ;
#23310=CARTESIAN_POINT ( 'NONE',  ( 20.99999999999999645, 242.2093750006144717, 6.646953231504538984 ) ) ;
#23320=CARTESIAN_POINT ( 'NONE',  ( 19.39230484541326760, 241.5986538117967370, 5.999999999999999112 ) ) ;
#23323=CARTESIAN_POINT ( 'NONE',  ( 23.87821517812499650, 241.9468750006145115, -4.985214923628404904 ) ) ;
#23329=( BOUNDED_CURVE ( )  B_SPLINE_CURVE ( 2, ( #8391, #16183, #16555, #2133, #27733, #30956, #22245, #10477, #10666 ),
 .UNSPECIFIED., .F., .F. ) 
 B_SPLINE_CURVE_WITH_KNOTS ( ( 3, 2, 2, 2, 3 ),
 ( 0.6458333333333333703, 0.6527777777777777901, 0.6666666666666666297, 0.6805555555555555802, 0.6875000000000000000 ),
 .UNSPECIFIED. ) 
 CURVE ( )  GEOMETRIC_REPRESENTATION_ITEM ( )  RATIONAL_B_SPLINE_CURVE ( ( 0.9330127018922192983, 0.9330127018922198534, 1.000000000000000000, 0.8660254037844387076, 1.000000000000000000, 0.8660254037844387076, 1.000000000000000000, 0.9330127018922194093, 0.9330127018922194093 ) ) 
 REPRESENTATION_ITEM ( '' )  );
#23331=CARTESIAN_POINT ( 'NONE',  ( 13.62178482187501416, 195.5093750006145399, 23.59362340125806767 ) ) ;
#23337=ORIENTED_EDGE ( 'NONE', *, *, #34029, .T. ) ;
#23338=CARTESIAN_POINT ( 'NONE',  ( 15.24356964374999990, 249.2968750006145058, 0.000000000000000000 ) ) ;
#23343=ORIENTED_EDGE ( 'NONE', *, *, #31169, .F. ) ;
#23345=CARTESIAN_POINT ( 'NONE',  ( 19.39230484541324628, 245.9138461906613315, -5.999999999999989342 ) ) ;
#23350=CARTESIAN_POINT ( 'NONE',  ( 18.12178482187499640, 248.7718750006145001, -4.985214923628404904 ) ) ;
#23356=CARTESIAN_POINT ( 'NONE',  ( -28.88880888891164744, 202.4104480656949079, 2.583632243664814254 ) ) ;
#23370=DIRECTION ( 'NONE',  ( -0.000000000000000000, 1.000000000000000000, -0.000000000000000000 ) ) ;
#23371=CARTESIAN_POINT ( 'NONE',  ( 7.234628195640295800, 197.4325961894323882, 27.00000000000001066 ) ) ;
#23373=EDGE_CURVE ( 'NONE', #1338, #21070, #29858, .T. ) ;
#23374=CARTESIAN_POINT ( 'NONE',  ( 15.24356964374999990, 244.4593750006145569, 0.000000000000000000 ) ) ;
#23377=ORIENTED_EDGE ( 'NONE', *, *, #7286, .F. ) ;
#23379=CARTESIAN_POINT ( 'NONE',  ( 26.99999999999999645, 246.7187500012290400, -3.464101615137755275 ) ) ;
#23392=CARTESIAN_POINT ( 'NONE',  ( 21.00000000000000000, 247.6093750006145342, 6.646953231504538984 ) ) ;
#23396=CARTESIAN_POINT ( 'NONE',  ( 15.84454946586586566, 211.9332939502924660, -5.693556627489360089 ) ) ;
#23406=ORIENTED_EDGE ( 'NONE', *, *, #15154, .F. ) ;
#23413=AXIS2_PLACEMENT_3D ( 'NONE', #13427, #7372, #36348 ) ;
#23417=CARTESIAN_POINT ( 'NONE',  ( 20.99999999999999645, 185.0294372515228645, -5.999999999999999112 ) ) ;
#23419=CARTESIAN_POINT ( 'NONE',  ( 13.50000000000001421, 196.1000000000000227, 23.38268590217984055 ) ) ;
#23420=CARTESIAN_POINT ( 'NONE',  ( 19.95811783012821650, 240.0005236131589754, -5.908847734042844912 ) ) ;
#23422=CARTESIAN_POINT ( 'NONE',  ( 23.87821517812499650, 245.6593750006145171, -4.985214923628404904 ) ) ;
#23423=ORIENTED_EDGE ( 'NONE', *, *, #12715, .F. ) ;
#23425=CARTESIAN_POINT ( 'NONE',  ( 26.99999999999999645, 243.4375000000000284, 3.464101615137751278 ) ) ;
#23426=FACE_OUTER_BOUND ( 'NONE', #16593, .T. ) ;
#23429=CARTESIAN_POINT ( 'NONE',  ( 18.00000000000000355, 240.1750000000000114, 5.196152422706632912 ) ) ;
#23440=CARTESIAN_POINT ( 'NONE',  ( 26.75643035624999655, 241.0843750006145285, -7.049594010296217766E-16 ) ) ;
#23449=CARTESIAN_POINT ( 'NONE',  ( 18.39679865110830548, 195.0000000000000284, -19.80091321147607886 ) ) ;
#23450=CARTESIAN_POINT ( 'NONE',  ( 13.62178482187499640, 196.1093750006145342, -23.59362340125807123 ) ) ;
#23464=CYLINDRICAL_SURFACE ( 'NONE', #8659, 27.00000000000000000 ) ;
#23466=CARTESIAN_POINT ( 'NONE',  ( 27.00000000000000355, 199.4375000012290400, -3.306546357697854128E-15 ) ) ;
#23471=CARTESIAN_POINT ( 'NONE',  ( 7.234628195640269155, 196.0825961894323939, 27.00000000000003197 ) ) ;
#23475=CARTESIAN_POINT ( 'NONE',  ( 18.00000000000000355, 247.8249999999999886, 5.196152422706632912 ) ) ;
#23476=CARTESIAN_POINT ( 'NONE',  ( 27.24356964375000345, 198.6781250006145569, -3.336375036156643733E-15 ) ) ;
#23480=ORIENTED_EDGE ( 'NONE', *, *, #581, .T. ) ;
#23482=CARTESIAN_POINT ( 'NONE',  ( 13.62178482187499640, 196.9531250006145342, -23.59362340125807123 ) ) ;
#23483=CARTESIAN_POINT ( 'NONE',  ( 15.24356964374999990, 242.9968750006145228, 0.000000000000000000 ) ) ;
#23487=CARTESIAN_POINT ( 'NONE',  ( 15.24356964374999990, 246.6718750006145342, -3.323476615752268604 ) ) ;
#23493=CARTESIAN_POINT ( 'NONE',  ( 23.87821517812500005, 241.7968750006145342, 4.985214923628404016 ) ) ;
#23504=EDGE_CURVE ( 'NONE', #7705, #483, #36931, .T. ) ;
#23508=CARTESIAN_POINT ( 'NONE',  ( 7.234628195640322446, 198.8950961906613770, 26.99999999999999645 ) ) ;
#23511=CARTESIAN_POINT ( 'NONE',  ( 4.999999999999997335, 216.0000000000000000, 7.347880794884120722E-16 ) ) ;
#23512=CARTESIAN_POINT ( 'NONE',  ( 23.87821517812500005, 242.2468750006145228, 4.985214923628404016 ) ) ;
#23517=CARTESIAN_POINT ( 'NONE',  ( 24.00000000000000000, 241.6000000000000227, 5.196152422706629359 ) ) ;
#23519=LINE ( 'NONE', #32792, #11223 ) ;
#23520=CARTESIAN_POINT ( 'NONE',  ( -1.057942093924267191, 194.9999999999999432, 27.27867916801710635 ) ) ;
#23525=ORIENTED_EDGE ( 'NONE', *, *, #26065, .F. ) ;
#23526=CARTESIAN_POINT ( 'NONE',  ( 15.00000000000000000, 240.1562500012290684, 0.000000000000000000 ) ) ;
#23530=DIRECTION ( 'NONE',  ( 0.000000000000000000, 0.000000000000000000, 1.000000000000000000 ) ) ;
#23533=ORIENTED_EDGE ( 'NONE', *, *, #16238, .F. ) ;
#23563=CARTESIAN_POINT ( 'NONE',  ( 23.87821517812499650, 245.6593750006145171, -4.985214923628404904 ) ) ;
#23565=CARTESIAN_POINT ( 'NONE',  ( 18.12178482187499640, 240.3343750006145285, -4.985214923628404904 ) ) ;
#23568=CARTESIAN_POINT ( 'NONE',  ( 26.99999999999999645, 246.2312500012290570, -7.347880794884117764E-16 ) ) ;
#23576=( BOUNDED_CURVE ( )  B_SPLINE_CURVE ( 2, ( #29488, #17943, #12434, #32706, #20602, #11866, #26834, #6371, #23625 ),
 .UNSPECIFIED., .F., .F. ) 
 B_SPLINE_CURVE_WITH_KNOTS ( ( 3, 2, 2, 2, 3 ),
 ( 0.3152173913043477826, 0.3188405797101449002, 0.3260869565217391353, 0.3333333333333333148, 0.3369565217391304324 ),
 .UNSPECIFIED. ) 
 CURVE ( )  GEOMETRIC_REPRESENTATION_ITEM ( )  RATIONAL_B_SPLINE_CURVE ( ( 0.9330127018922191873, 0.9330127018922187432, 1.000000000000000000, 0.8660254037844387076, 1.000000000000000000, 0.8660254037844387076, 1.000000000000000000, 0.9330127018922194093, 0.9330127018922194093 ) ) 
 REPRESENTATION_ITEM ( '' )  );
#23580=CARTESIAN_POINT ( 'NONE',  ( 18.12178482187500350, 247.5718750006145115, 4.985214923628407568 ) ) ;
#23594=ORIENTED_EDGE ( 'NONE', *, *, #36699, .T. ) ;
#23602=FACE_OUTER_BOUND ( 'NONE', #32617, .T. ) ;
#23604=CARTESIAN_POINT ( 'NONE',  ( 20.99999999999999289, 248.9874999999999829, -5.999999999999997335 ) ) ;
#23607=CARTESIAN_POINT ( 'NONE',  ( 15.24356964375000167, 247.1968750006145115, 3.323476615752272600 ) ) ;
#23609=VERTEX_POINT ( 'NONE', #16112 ) ;
#23611=( BOUNDED_CURVE ( )  B_SPLINE_CURVE ( 2, ( #35859, #7814, #13308, #10092, #7627, #21662, #19202, #15978, #16345 ),
 .UNSPECIFIED., .F., .F. ) 
 B_SPLINE_CURVE_WITH_KNOTS ( ( 3, 2, 2, 2, 3 ),
 ( 0.4673913043478261087, 0.4710144927536231707, 0.4782608695652174058, 0.4855072463768115854, 0.4891304347826087029 ),
 .UNSPECIFIED. ) 
 CURVE ( )  GEOMETRIC_REPRESENTATION_ITEM ( )  RATIONAL_B_SPLINE_CURVE ( ( 0.9330127018922194093, 0.9330127018922198534, 1.000000000000000000, 0.8660254037844387076, 1.000000000000000000, 0.8660254037844387076, 1.000000000000000000, 0.9330127018922194093, 0.9330127018922194093 ) ) 
 REPRESENTATION_ITEM ( '' )  );
#23614=DIRECTION ( 'NONE',  ( -4.130293990420971855E-17, 1.000000000000000000, 0.000000000000000000 ) ) ;
#23617=CARTESIAN_POINT ( 'NONE',  ( 15.00000000000000000, 240.5125000000000171, -3.464101615137752166 ) ) ;
#23618=EDGE_CURVE ( 'NONE', #13079, #21280, #16485, .T. ) ;
#23622=VERTEX_POINT ( 'NONE', #4720 ) ;
#23625=CARTESIAN_POINT ( 'NONE',  ( 21.00000000000000000, 246.5124999999999602, 5.999999999999998224 ) ) ;
#23626=CARTESIAN_POINT ( 'NONE',  ( 15.00000000000000178, 248.2375000000000398, 3.464101615137757051 ) ) ;
#23633=CARTESIAN_POINT ( 'NONE',  ( 18.12178482187499640, 240.7843750006145171, -4.985214923628404904 ) ) ;
#23642=CARTESIAN_POINT ( 'NONE',  ( 27.11680205743124361, 195.0000000000000284, 0.9911108661349460336 ) ) ;
#23643=CARTESIAN_POINT ( 'NONE',  ( 13.62178482187499640, 197.0093750006145399, -23.59362340125807123 ) ) ;
#23648=DIRECTION ( 'NONE',  ( -1.734723475976807094E-15, 0.000000000000000000, 1.000000000000000000 ) ) ;
#23655=CARTESIAN_POINT ( 'NONE',  ( 23.99999999999999645, 244.9000000000000057, -5.196152422706631135 ) ) ;
#23657=CARTESIAN_POINT ( 'NONE',  ( 26.99999999999999645, 199.4750000012290343, -15.58845726811990495 ) ) ;
#23659=VERTEX_POINT ( 'NONE', #30322 ) ;
#23666=CARTESIAN_POINT ( 'NONE',  ( 15.00000000000000000, 249.0624999999999716, -3.464101615137752166 ) ) ;
#23667=CARTESIAN_POINT ( 'NONE',  ( 13.62178482187501416, 196.8031250006145285, 23.59362340125806767 ) ) ;
#23671=ORIENTED_EDGE ( 'NONE', *, *, #30568, .T. ) ;
#23672=CARTESIAN_POINT ( 'NONE',  ( 27.24356964374999635, 196.4656250006145228, -15.72908226750539029 ) ) ;
#23673=CARTESIAN_POINT ( 'NONE',  ( 15.24356964374999990, 239.8093750006145228, -3.323476615752268604 ) ) ;
#23676=CARTESIAN_POINT ( 'NONE',  ( 18.12178482187499640, 247.0843750006145285, -4.985214923628404904 ) ) ;
#23681=EDGE_CURVE ( 'NONE', #23017, #21628, #3281, .T. ) ;
#23682=CARTESIAN_POINT ( 'NONE',  ( 23.87821517812500005, 242.2468750006145228, 4.985214923628404016 ) ) ;
#23695=CARTESIAN_POINT ( 'NONE',  ( 27.00000000000001421, 198.3875000000000171, 15.58845726811988897 ) ) ;
#23697=CARTESIAN_POINT ( 'NONE',  ( 27.00000000000001421, 198.9500000012290002, 15.58845726811988897 ) ) ;
#23698=ADVANCED_FACE ( 'NONE', ( #14007 ), #918, .F. ) ;
#23701=CARTESIAN_POINT ( 'NONE',  ( 26.75643035624999655, 242.8093750006144944, -3.323476615752271712 ) ) ;
#23703=EDGE_CURVE ( 'NONE', #10385, #23800, #7187, .T. ) ;
#23707=CARTESIAN_POINT ( 'NONE',  ( 20.99999999999999645, 185.0294372515228645, 0.000000000000000000 ) ) ;
#23714=CARTESIAN_POINT ( 'NONE',  ( 23.87821517812499650, 246.8968750006145285, -4.985214923628404904 ) ) ;
#23721=FACE_OUTER_BOUND ( 'NONE', #29246, .T. ) ;
#23722=VERTEX_POINT ( 'NONE', #25374 ) ;
#23724=AXIS2_PLACEMENT_3D ( 'NONE', #22310, #16440, #8092 ) ;
#23727=EDGE_CURVE ( 'NONE', #33209, #17126, #32061, .T. ) ;
#23729=CARTESIAN_POINT ( 'NONE',  ( 15.24356964374999990, 248.8468750006145171, 0.000000000000000000 ) ) ;
#23734=CARTESIAN_POINT ( 'NONE',  ( 26.99999999999999645, 248.0687500012290627, -3.464101615137755275 ) ) ;
#23737=AXIS2_PLACEMENT_3D ( 'NONE', #13074, #4163, #6632 ) ;
#23742=ORIENTED_EDGE ( 'NONE', *, *, #28696, .T. ) ;
#23752=CARTESIAN_POINT ( 'NONE',  ( 18.12178482187499640, 242.1343750006145115, -4.985214923628404904 ) ) ;
#23754=CARTESIAN_POINT ( 'NONE',  ( 15.24356964374999990, 239.9593750006145285, 0.000000000000000000 ) ) ;
#23756=CARTESIAN_POINT ( 'NONE',  ( 21.00000000000000000, 246.1187500012290172, 6.928203230275506996 ) ) ;
#23759=CARTESIAN_POINT ( 'NONE',  ( 20.99999999999997513, 246.7375000000000114, -5.999999999999999112 ) ) ;
#23767=CARTESIAN_POINT ( 'NONE',  ( 26.75643035624999655, 247.2718750006145001, -7.049594010296217766E-16 ) ) ;
#23770=AXIS2_PLACEMENT_3D ( 'NONE', #35800, #27655, #18385 ) ;
#23772=CARTESIAN_POINT ( 'NONE',  ( 12.98158921324743176, 213.0069040450241005, -5.206989594062311433 ) ) ;
#23774=B_SPLINE_CURVE_WITH_KNOTS ( 'NONE', 3,
 ( #33590, #7629, #4774, #27896, #25793, #22779, #19944, #11951, #14805, #26164, #20682, #31852, #23520, #5697, #32228, #29188, #37342, #35066 ),
 .UNSPECIFIED., .F., .F.,
 ( 4, 2, 2, 2, 2, 2, 2, 2, 4 ),
 ( 0.000000000000000000, 0.002646020752430532173, 0.005292041504861064345, 0.007938062257291596951, 0.009261072633506861954, 0.01058408300972212696, 0.01587612451458319390, 0.01852214526701372391, 0.02116816601944425738 ),
 .UNSPECIFIED. ) ;
#23781=CARTESIAN_POINT ( 'NONE',  ( 20.99999999999999645, 185.0294372515228645, 0.000000000000000000 ) ) ;
#23797=CARTESIAN_POINT ( 'NONE',  ( 18.00000000000000000, 247.2812500012290400, -5.196152422706630247 ) ) ;
#23799=CARTESIAN_POINT ( 'NONE',  ( 18.12178482187499640, 247.0843750006145285, -4.985214923628404904 ) ) ;
#23800=VERTEX_POINT ( 'NONE', #19524 ) ;
#23806=CARTESIAN_POINT ( 'NONE',  ( 15.00000000000000000, 240.0999999999999943, 0.000000000000000000 ) ) ;
#23807=CARTESIAN_POINT ( 'NONE',  ( -9.244144843276098200, 218.8666023059713268, 3.366928170503552309 ) ) ;
#23809=EDGE_LOOP ( 'NONE', ( #18823, #28035, #23904, #32042 ) ) ;
#23814=CARTESIAN_POINT ( 'NONE',  ( 20.99999999999995026, 243.1375000000000455, -5.999999999999998224 ) ) ;
#23818=CARTESIAN_POINT ( 'NONE',  ( 26.99999999999999645, 249.2874999999999943, 3.464101615137751278 ) ) ;
#23819=CARTESIAN_POINT ( 'NONE',  ( 26.75643035624999655, 240.6343750006145115, -7.049594010296217766E-16 ) ) ;
#23829=CARTESIAN_POINT ( 'NONE',  ( -27.24356964374999990, 198.8656250006145569, -15.72908226750537786 ) ) ;
#23835=CARTESIAN_POINT ( 'NONE',  ( 22.60769515458672885, 245.2388461906613486, 5.999999999999997335 ) ) ;
#23836=CARTESIAN_POINT ( 'NONE',  ( 19.39230484541324628, 247.2075961894323086, -5.999999999999989342 ) ) ;
#23846=VECTOR ( 'NONE', #25703, 1000.000000000000000 ) ;
#23850=CARTESIAN_POINT ( 'NONE',  ( 1.120210788295102201E-13, 195.0500000012290798, -27.00000000000000711 ) ) ;
#23851=ORIENTED_EDGE ( 'NONE', *, *, #4027, .T. ) ;
#23854=CARTESIAN_POINT ( 'NONE',  ( -13.49999999999998401, 198.3875000012290286, 23.38268590217985476 ) ) ;
#23858=CARTESIAN_POINT ( 'NONE',  ( 24.00000000000000000, 247.9000000000000057, 5.196152422706629359 ) ) ;
#23859=CARTESIAN_POINT ( 'NONE',  ( 13.62178482187499640, 196.5031250006145456, -23.59362340125807123 ) ) ;
#23863=CARTESIAN_POINT ( 'NONE',  ( 27.24356964375000345, 195.0781250006145342, -3.336375036156643733E-15 ) ) ;
#23864=CARTESIAN_POINT ( 'NONE',  ( 26.75643035624999655, 240.4843750006145058, 3.323476615752267715 ) ) ;
#23867=CARTESIAN_POINT ( 'NONE',  ( 23.87821517812500005, 247.3093750006145228, 4.985214923628404016 ) ) ;
#23876=CARTESIAN_POINT ( 'NONE',  ( 15.24356964374999990, 242.9593750006145001, -3.323476615752268604 ) ) ;
#23890=CARTESIAN_POINT ( 'NONE',  ( 19.39230484541326405, 248.3486538117967370, 5.999999999999995559 ) ) ;
#23893=CARTESIAN_POINT ( 'NONE',  ( 15.24356964375000167, 243.0343750006144887, 3.323476615752272600 ) ) ;
#23904=ORIENTED_EDGE ( 'NONE', *, *, #30346, .T. ) ;
#23906=CARTESIAN_POINT ( 'NONE',  ( 26.75643035624999655, 246.7843750006145171, 3.323476615752267715 ) ) ;
#23919=CARTESIAN_POINT ( 'NONE',  ( 15.24356964374999990, 249.7093750006145285, -3.323476615752268604 ) ) ;
#23921=CARTESIAN_POINT ( 'NONE',  ( 3.551475717527324030E-15, 210.0000000000000284, 28.99999999999999645 ) ) ;
#23925=ORIENTED_EDGE ( 'NONE', *, *, #8524, .T. ) ;
#23926=CARTESIAN_POINT ( 'NONE',  ( 20.99999999999999645, 185.0294372515228645, -5.999999999999999112 ) ) ;
#23930=CARTESIAN_POINT ( 'NONE',  ( 20.99999999999995026, 241.3375000000000341, -5.999999999999998224 ) ) ;
#23934=CARTESIAN_POINT ( 'NONE',  ( 7.234628195640295800, 197.5450961906613827, 27.00000000000001066 ) ) ;
#23939=CARTESIAN_POINT ( 'NONE',  ( 7.234628195640269155, 195.7450961906613713, 27.00000000000003197 ) ) ;
#23947=CARTESIAN_POINT ( 'NONE',  ( 21.00000000000000000, 243.6437500012290513, -6.928203230275506996 ) ) ;
#23950=PLANE ( 'NONE',  #5779 ) ;
#23955=VERTEX_POINT ( 'NONE', #31253 ) ;
#23958=CARTESIAN_POINT ( 'NONE',  ( 26.75643035624999655, 244.0843750006145285, 3.323476615752267715 ) ) ;
#23986=CARTESIAN_POINT ( 'NONE',  ( -7.234628195640263826, 195.4075961894323825, -27.00000000000003553 ) ) ;
#23988=CARTESIAN_POINT ( 'NONE',  ( 26.75643035624999655, 249.6718750006145342, -3.323476615752271712 ) ) ;
#23990=CARTESIAN_POINT ( 'NONE',  ( 15.24356964374999990, 246.6718750006145342, -3.323476615752268604 ) ) ;
#24001=CYLINDRICAL_SURFACE ( 'NONE', #1251, 5.999999999999999112 ) ;
#24008=( BOUNDED_CURVE ( )  B_SPLINE_CURVE ( 2, ( #24907, #22449, #31162, #7670, #33996, #4995, #27937, #28123, #13734 ),
 .UNSPECIFIED., .F., .F. ) 
 B_SPLINE_CURVE_WITH_KNOTS ( ( 3, 2, 2, 2, 3 ),
 ( 0.2065217391304347838, 0.2101449275362318736, 0.2173913043478260809, 0.2246376811594202882, 0.2282608695652173780 ),
 .UNSPECIFIED. ) 
 CURVE ( )  GEOMETRIC_REPRESENTATION_ITEM ( )  RATIONAL_B_SPLINE_CURVE ( ( 0.9330127018922194093, 0.9330127018922194093, 1.000000000000000000, 0.8660254037844387076, 1.000000000000000000, 0.8660254037844387076, 1.000000000000000000, 0.9330127018922196314, 0.9330127018922194093 ) ) 
 REPRESENTATION_ITEM ( '' )  );
#24009=CARTESIAN_POINT ( 'NONE',  ( -13.50000000000000533, 197.2250000000000227, -23.38268590217984411 ) ) ;
#24010=VECTOR ( 'NONE', #35960, 1000.000000000000000 ) ;
#24011=CARTESIAN_POINT ( 'NONE',  ( 20.99999999999999289, 243.6437500012290229, -5.999999999999997335 ) ) ;
#24018=CARTESIAN_POINT ( 'NONE',  ( 21.00000000000000000, 241.1125000000000114, 5.999999999999998224 ) ) ;
#24019=CARTESIAN_POINT ( 'NONE',  ( 27.24356964375000345, 199.5781250006145342, -3.336375036156643733E-15 ) ) ;
#24035=DIRECTION ( 'NONE',  ( 0.000000000000000000, 0.000000000000000000, -1.000000000000000000 ) ) ;
#24040=CARTESIAN_POINT ( 'NONE',  ( 5.438367727407757144E-14, 198.2000000012290002, -27.00000000000000000 ) ) ;
#24044=CARTESIAN_POINT ( 'NONE',  ( 18.00000000000000000, 245.8750000000000000, -5.196152422706630247 ) ) ;
#24045=CARTESIAN_POINT ( 'NONE',  ( -1.926257025242585782E-15, 195.6406250006145342, -31.45816453501076637 ) ) ;
#24050=CARTESIAN_POINT ( 'NONE',  ( 13.62178482187501416, 195.9031250006145513, 23.59362340125806767 ) ) ;
#24051=CARTESIAN_POINT ( 'NONE',  ( 18.12178482187499640, 240.6718750006145058, -4.985214923628404904 ) ) ;
#24054=CARTESIAN_POINT ( 'NONE',  ( 23.87821517812499650, 247.0093750006145399, -4.985214923628404904 ) ) ;
#24057=EDGE_CURVE ( 'NONE', #24921, #25531, #4514, .T. ) ;
#24061=FACE_OUTER_BOUND ( 'NONE', #30488, .T. ) ;
#24063=( BOUNDED_CURVE ( )  B_SPLINE_CURVE ( 2, ( #34587, #20015, #11290, #19655, #17355, #34408, #16616, #10913, #5400 ),
 .UNSPECIFIED., .F., .F. ) 
 B_SPLINE_CURVE_WITH_KNOTS ( ( 3, 2, 2, 2, 3 ),
 ( 0.7065217391304348116, 0.7101449275362319291, 0.7173913043478260532, 0.7246376811594202882, 0.7282608695652174058 ),
 .UNSPECIFIED. ) 
 CURVE ( )  GEOMETRIC_REPRESENTATION_ITEM ( )  RATIONAL_B_SPLINE_CURVE ( ( 0.9330127018922194093, 0.9330127018922194093, 1.000000000000000000, 0.8660254037844387076, 1.000000000000000000, 0.8660254037844387076, 1.000000000000000000, 0.9330127018922194093, 0.9330127018922194093 ) ) 
 REPRESENTATION_ITEM ( '' )  );
#24078=CARTESIAN_POINT ( 'NONE',  ( 15.24356964375000167, 248.9968750006145513, 3.323476615752272600 ) ) ;
#24082=CARTESIAN_POINT ( 'NONE',  ( 21.00000000000000000, 242.4625000000000057, 5.999999999999998224 ) ) ;
#24085=FACE_OUTER_BOUND ( 'NONE', #6996, .T. ) ;
#24091=CARTESIAN_POINT ( 'NONE',  ( 23.87821517812500005, 247.6468750006145285, 4.985214923628404016 ) ) ;
#24105=ADVANCED_FACE ( 'NONE', ( #15122 ), #12276, .F. ) ;
#24108=CARTESIAN_POINT ( 'NONE',  ( 20.99999999999999645, 247.6093750006145342, 6.646953231504538984 ) ) ;
#24114=VERTEX_POINT ( 'NONE', #35580 ) ;
#24119=CARTESIAN_POINT ( 'NONE',  ( 19.39230484541323918, 241.3575961894323427, -5.999999999999987566 ) ) ;
#24122=EDGE_LOOP ( 'NONE', ( #9017, #16999, #8244, #28370 ) ) ;
#24129=CARTESIAN_POINT ( 'NONE',  ( -27.24356964374999990, 199.3718750006145513, -15.72908226750537786 ) ) ;
#24132=( BOUNDED_CURVE ( )  B_SPLINE_CURVE ( 2, ( #2443, #8695, #14571, #25942, #3185, #29144, #26305, #22740, #34839 ),
 .UNSPECIFIED., .F., .F. ) 
 B_SPLINE_CURVE_WITH_KNOTS ( ( 3, 2, 2, 2, 3 ),
 ( 0.3125000000000000000, 0.3194444444444444198, 0.3333333333333333148, 0.3472222222222222099, 0.3541666666666666852 ),
 .UNSPECIFIED. ) 
 CURVE ( )  GEOMETRIC_REPRESENTATION_ITEM ( )  RATIONAL_B_SPLINE_CURVE ( ( 0.9330127018922194093, 0.9330127018922194093, 1.000000000000000000, 0.8660254037844387076, 1.000000000000000000, 0.8660254037844387076, 1.000000000000000000, 0.9330127018922190762, 0.9330127018922194093 ) ) 
 REPRESENTATION_ITEM ( '' )  );
#24137=CARTESIAN_POINT ( 'NONE',  ( 18.00000000000000355, 243.3812500012290343, 5.196152422706632912 ) ) ;
#24140=CARTESIAN_POINT ( 'NONE',  ( 15.00000000000000000, 242.7999999999999829, 0.000000000000000000 ) ) ;
#24143=ORIENTED_EDGE ( 'NONE', *, *, #5092, .T. ) ;
#24145=CARTESIAN_POINT ( 'NONE',  ( 18.12178482187500350, 244.4218750006145058, 4.985214923628407568 ) ) ;
#24162=ORIENTED_EDGE ( 'NONE', *, *, #18177, .F. ) ;
#24171=CARTESIAN_POINT ( 'NONE',  ( 19.39230484541326760, 247.4486538117967314, 5.999999999999999112 ) ) ;
#24173=CARTESIAN_POINT ( 'NONE',  ( 20.99999999999999645, 246.3718750006144944, 6.646953231504538984 ) ) ;
#24176=FACE_OUTER_BOUND ( 'NONE', #10570, .T. ) ;
#24185=CARTESIAN_POINT ( 'NONE',  ( 1.069080835302379631E-14, 196.6250000012290400, 27.00000000000000000 ) ) ;
#24194=CARTESIAN_POINT ( 'NONE',  ( 17.52409618574002792, 213.4759038142795191, 5.188047882455193438 ) ) ;
#24203=CARTESIAN_POINT ( 'NONE',  ( 27.24356964374999635, 197.8156250006145171, -15.72908226750539029 ) ) ;
#24226=AXIS2_PLACEMENT_3D ( 'NONE', #25054, #30752, #10461 ) ;
#24231=CARTESIAN_POINT ( 'NONE',  ( 26.99999999999999645, 247.0749999999999886, -7.347880794884117764E-16 ) ) ;
#24232=CARTESIAN_POINT ( 'NONE',  ( -27.24356964374999279, 195.7906250006145399, 15.72908226750539384 ) ) ;
#24237=CARTESIAN_POINT ( 'NONE',  ( 27.24356964375000700, 195.9406250006145456, 15.72908226750537075 ) ) ;
#24242=CARTESIAN_POINT ( 'NONE',  ( 21.00000000000000000, 245.0218750006145285, 6.646953231504538984 ) ) ;
#24250=CARTESIAN_POINT ( 'NONE',  ( 18.12178482187499640, 240.6718750006145058, -4.985214923628404904 ) ) ;
#24260=CARTESIAN_POINT ( 'NONE',  ( 20.99999999999998579, 248.5374999999999659, -5.999999999999997335 ) ) ;
#24261=FACE_OUTER_BOUND ( 'NONE', #14390, .T. ) ;
#24262=CARTESIAN_POINT ( 'NONE',  ( 27.00000000000000355, 198.4250000000000114, -3.306546357697854128E-15 ) ) ;
#24267=CARTESIAN_POINT ( 'NONE',  ( 18.12178482187499640, 240.6718750006145058, -4.985214923628404904 ) ) ;
#24271=ADVANCED_FACE ( 'NONE', ( #4122 ), #10042, .T. ) ;
#24272=CARTESIAN_POINT ( 'NONE',  ( -27.24356964375000345, 199.4093750006145456, 0.000000000000000000 ) ) ;
#24274=CARTESIAN_POINT ( 'NONE',  ( 20.99999999999999645, 185.0294372515228645, 0.000000000000000000 ) ) ;
#24275=CARTESIAN_POINT ( 'NONE',  ( 20.99999999999999645, 185.0294372515228645, 5.999999999999999112 ) ) ;
#24279=ORIENTED_EDGE ( 'NONE', *, *, #13410, .F. ) ;
#24280=EDGE_LOOP ( 'NONE', ( #10846, #16911, #26881, #9235, #8628, #2479 ) ) ;
#24281=CARTESIAN_POINT ( 'NONE',  ( 18.12178482187500350, 248.0218750006145001, 4.985214923628407568 ) ) ;
#24286=CARTESIAN_POINT ( 'NONE',  ( 20.99999999999999645, 250.0000000000000000, 0.000000000000000000 ) ) ;
#24287=ORIENTED_EDGE ( 'NONE', *, *, #30910, .F. ) ;
#24290=VERTEX_POINT ( 'NONE', #8739 ) ;
#24294=VECTOR ( 'NONE', #21724, 1000.000000000000000 ) ;
#24296=CARTESIAN_POINT ( 'NONE',  ( 18.12178482187500350, 246.2218750006145171, 4.985214923628407568 ) ) ;
#24301=VERTEX_POINT ( 'NONE', #11575 ) ;
#24302=CARTESIAN_POINT ( 'NONE',  ( -27.99076334771182673, 207.4091998227514182, 7.586839709977279078 ) ) ;
#24307=CARTESIAN_POINT ( 'NONE',  ( 15.00000000000000000, 249.1562500012290400, 0.000000000000000000 ) ) ;
#24310=VERTEX_POINT ( 'NONE', #20497 ) ;
#24317=CARTESIAN_POINT ( 'NONE',  ( -27.00000000000000355, 196.3625000000000114, -15.58845726811989429 ) ) ;
#24324=CARTESIAN_POINT ( 'NONE',  ( 21.00000000000000000, 243.8687500012290172, 6.928203230275506996 ) ) ;
#24327=DIRECTION ( 'NONE',  ( 0.000000000000000000, -0.000000000000000000, -1.000000000000000000 ) ) ;
#24333=CARTESIAN_POINT ( 'NONE',  ( 26.75643035624999655, 244.5718750006145115, -7.049594010296217766E-16 ) ) ;
#24335=( BOUNDED_CURVE ( )  B_SPLINE_CURVE ( 2, ( #37446, #16826, #22704, #11313, #26260, #20039, #8107, #11127, #14344 ),
 .UNSPECIFIED., .F., .F. ) 
 B_SPLINE_CURVE_WITH_KNOTS ( ( 3, 2, 2, 2, 3 ),
 ( 0.2291666666666666574, 0.2361111111111111049, 0.2500000000000000000, 0.2638888888888888951, 0.2708333333333333703 ),
 .UNSPECIFIED. ) 
 CURVE ( )  GEOMETRIC_REPRESENTATION_ITEM ( )  RATIONAL_B_SPLINE_CURVE ( ( 0.9330127018922194093, 0.9330127018922194093, 1.000000000000000000, 0.8660254037844387076, 1.000000000000000000, 0.8660254037844387076, 1.000000000000000000, 0.9330127018922190762, 0.9330127018922194093 ) ) 
 REPRESENTATION_ITEM ( '' )  );
#24344=CARTESIAN_POINT ( 'NONE',  ( 20.99999999999999645, 246.5124999999999602, 5.999999999999998224 ) ) ;
#24352=LINE ( 'NONE', #7472, #1018 ) ;
#24360=CARTESIAN_POINT ( 'NONE',  ( 23.87821517812499650, 249.2593750006145399, -4.985214923628404904 ) ) ;
#24362=CARTESIAN_POINT ( 'NONE',  ( 23.87821517812499650, 243.8593750006145342, -4.985214923628404904 ) ) ;
#24374=CARTESIAN_POINT ( 'NONE',  ( -27.87471972953270338, 210.0000000000000284, 8.000000000000000000 ) ) ;
#24381=CARTESIAN_POINT ( 'NONE',  ( -7.234628195640263826, 197.2075961894323370, -27.00000000000003553 ) ) ;
#24382=CARTESIAN_POINT ( 'NONE',  ( 19.55576478543887831, 211.4442352145762527, 5.894939585073154298 ) ) ;
#24390=CARTESIAN_POINT ( 'NONE',  ( -27.24356964374999635, 198.0406250006145399, 15.72908226750539384 ) ) ;
#24396=DIRECTION ( 'NONE',  ( -0.000000000000000000, -1.000000000000000000, -0.000000000000000000 ) ) ;
#24405=CARTESIAN_POINT ( 'NONE',  ( 15.00000000000000000, 249.6062500012290570, 0.000000000000000000 ) ) ;
#24407=CARTESIAN_POINT ( 'NONE',  ( 27.00000000000001066, 199.7375000000000114, 15.58845726811988897 ) ) ;
#24408=CARTESIAN_POINT ( 'NONE',  ( 24.00000000000000000, 247.5062500012290627, 5.196152422706629359 ) ) ;
#24411=CARTESIAN_POINT ( 'NONE',  ( 20.99999999999999645, 242.0124999999999886, 5.999999999999998224 ) ) ;
#24418=CARTESIAN_POINT ( 'NONE',  ( 24.00000000000000000, 245.1999999999999886, 5.196152422706629359 ) ) ;
#24420=CARTESIAN_POINT ( 'NONE',  ( -27.24356964374999279, 196.2406250006145285, 15.72908226750539384 ) ) ;
#24425=CARTESIAN_POINT ( 'NONE',  ( 27.00000000000000355, 197.6375000012290286, -3.306546357697854128E-15 ) ) ;
#24426=CARTESIAN_POINT ( 'NONE',  ( 21.00000000000000000, 240.4093750006145171, 6.646953231504538984 ) ) ;
#24429=CARTESIAN_POINT ( 'NONE',  ( 18.12178482187500350, 245.4343750006145228, 4.985214923628407568 ) ) ;
#24434=EDGE_CURVE ( 'NONE', #19674, #22517, #21065, .T. ) ;
#24436=CARTESIAN_POINT ( 'NONE',  ( 23.87821517812499650, 240.5968750006145171, -4.985214923628404904 ) ) ;
#24446=CARTESIAN_POINT ( 'NONE',  ( 19.39230484541326760, 244.2424038105676516, 5.999999999999999112 ) ) ;
#24450=CARTESIAN_POINT ( 'NONE',  ( 23.87821517812499650, 240.5968750006145171, -4.985214923628404904 ) ) ;
#24451=ORIENTED_EDGE ( 'NONE', *, *, #2440, .T. ) ;
#24455=CARTESIAN_POINT ( 'NONE',  ( 26.99999999999999645, 242.5374999999999943, 3.464101615137751278 ) ) ;
#24456=CARTESIAN_POINT ( 'NONE',  ( 19.97221621173429540, 239.9536485273282835, -5.828891293067281154 ) ) ;
#24459=CARTESIAN_POINT ( 'NONE',  ( 21.00000000000000000, 241.8718750006145228, 6.646953231504538984 ) ) ;
#24467=CARTESIAN_POINT ( 'NONE',  ( 26.75643035624999655, 247.2718750006145001, -7.049594010296217766E-16 ) ) ;
#24473=ORIENTED_EDGE ( 'NONE', *, *, #22391, .T. ) ;
#24480=CARTESIAN_POINT ( 'NONE',  ( 23.87821517812499650, 247.7968750006145058, -4.985214923628404904 ) ) ;
#24492=DIRECTION ( 'NONE',  ( 0.000000000000000000, 0.000000000000000000, 1.000000000000000000 ) ) ;
#24496=ORIENTED_EDGE ( 'NONE', *, *, #22827, .T. ) ;
#24497=CARTESIAN_POINT ( 'NONE',  ( 7.234628195640337545, 197.7299038117967029, -26.99999999999999289 ) ) ;
#24502=CARTESIAN_POINT ( 'NONE',  ( 5.778771075727756162E-15, 199.0718750006145399, 31.45816453501075927 ) ) ;
#24504=CARTESIAN_POINT ( 'NONE',  ( 2.999999999999997335, 252.0000000000000000, -2.500000000000000000 ) ) ;
#24507=CARTESIAN_POINT ( 'NONE',  ( 15.00000000000000178, 243.7937500012290570, 3.464101615137757051 ) ) ;
#24515=CARTESIAN_POINT ( 'NONE',  ( 23.87821517812500005, 244.0468750006145058, 4.985214923628404016 ) ) ;
#24532=EDGE_CURVE ( 'NONE', #10609, #25022, #23519, .T. ) ;
#24533=CARTESIAN_POINT ( 'NONE',  ( -28.51642293503100944, 203.9737468885152794, -5.287141534248642749 ) ) ;
#24534=VERTEX_POINT ( 'NONE', #20681 ) ;
#24541=VECTOR ( 'NONE', #35629, 1000.000000000000000 ) ;
#24544=CARTESIAN_POINT ( 'NONE',  ( 15.24356964374999990, 244.4593750006145569, 0.000000000000000000 ) ) ;
#24546=CARTESIAN_POINT ( 'NONE',  ( 21.00000000000000000, 245.2187500012290116, 5.999999999999998224 ) ) ;
#24559=CARTESIAN_POINT ( 'NONE',  ( 14.99999999999999289, 204.0000000000000000, 0.000000000000000000 ) ) ;
#24564=CARTESIAN_POINT ( 'NONE',  ( 20.99999999999999645, 210.0000000000000000, 5.999999999999996447 ) ) ;
#24574=CARTESIAN_POINT ( 'NONE',  ( -27.24356964375000345, 198.9031250006145228, 0.000000000000000000 ) ) ;
#24590=CARTESIAN_POINT ( 'NONE',  ( 27.00000000000000355, 199.3249999999999886, -3.306546357697854128E-15 ) ) ;
#24591=DIRECTION ( 'NONE',  ( -0.000000000000000000, 1.000000000000000000, -0.000000000000000000 ) ) ;
#24594=CARTESIAN_POINT ( 'NONE',  ( 21.00000000000000000, 242.0124999999999886, 5.999999999999998224 ) ) ;
#24595=ORIENTED_EDGE ( 'NONE', *, *, #10646, .T. ) ;
#24600=CARTESIAN_POINT ( 'NONE',  ( 15.00000000000000000, 246.3625000000000114, -3.464101615137752166 ) ) ;
#24605=ORIENTED_EDGE ( 'NONE', *, *, #23303, .T. ) ;
#24607=CARTESIAN_POINT ( 'NONE',  ( 13.50000000000001421, 198.4625000012290172, 23.38268590217984055 ) ) ;
#24611=CARTESIAN_POINT ( 'NONE',  ( 21.00000000000000000, 245.6968750006145399, -6.646953231504538984 ) ) ;
#24613=( BOUNDED_CURVE ( )  B_SPLINE_CURVE ( 2, ( #22075, #18684, #10873, #19245, #7293, #33627, #4437, #16574, #7477 ),
 .UNSPECIFIED., .F., .F. ) 
 B_SPLINE_CURVE_WITH_KNOTS ( ( 3, 2, 2, 2, 3 ),
 ( 0.2282608695652173780, 0.2318840579710144956, 0.2391304347826087029, 0.2463768115942029102, 0.2500000000000000000 ),
 .UNSPECIFIED. ) 
 CURVE ( )  GEOMETRIC_REPRESENTATION_ITEM ( )  RATIONAL_B_SPLINE_CURVE ( ( 0.9330127018922194093, 0.9330127018922190762, 1.000000000000000000, 0.8660254037844387076, 1.000000000000000000, 0.8660254037844387076, 1.000000000000000000, 0.9330127018922196314, 0.9330127018922194093 ) ) 
 REPRESENTATION_ITEM ( '' )  );
#24615=PLANE ( 'NONE',  #23413 ) ;
#24619=CARTESIAN_POINT ( 'NONE',  ( 20.00041244883536606, 239.7473985345926053, -5.668978318349186196 ) ) ;
#24632=CARTESIAN_POINT ( 'NONE',  ( 15.24356964374999990, 240.2593750006145115, -3.323476615752268604 ) ) ;
#24636=CARTESIAN_POINT ( 'NONE',  ( -13.62178482187498396, 198.1343750006145399, 23.59362340125808188 ) ) ;
#24638=CARTESIAN_POINT ( 'NONE',  ( 15.00000000000000000, 239.7062500012290513, 0.000000000000000000 ) ) ;
#24639=CARTESIAN_POINT ( 'NONE',  ( 15.24356964374999990, 243.5218750006145569, -3.323476615752268604 ) ) ;
#24643=VERTEX_POINT ( 'NONE', #3229 ) ;
#24645=CARTESIAN_POINT ( 'NONE',  ( 21.00000000000000000, 244.6843750006144944, -6.646953231504538984 ) ) ;
#24652=ORIENTED_EDGE ( 'NONE', *, *, #1028, .F. ) ;
#24659=CARTESIAN_POINT ( 'NONE',  ( 15.24356964374999990, 247.9093750006145171, -3.323476615752268604 ) ) ;
#24660=CARTESIAN_POINT ( 'NONE',  ( 1.255007937094097924E-14, 199.1000000012290627, -27.00000000000000000 ) ) ;
#24664=EDGE_CURVE ( 'NONE', #28768, #17657, #6643, .T. ) ;
#24680=CARTESIAN_POINT ( 'NONE',  ( 5.778771075727756162E-15, 196.8218750006145399, 31.45816453501075927 ) ) ;
#24685=CARTESIAN_POINT ( 'NONE',  ( 18.00000000000000000, 243.2312500012290570, -5.196152422706630247 ) ) ;
#24692=ORIENTED_EDGE ( 'NONE', *, *, #14594, .F. ) ;
#24696=ADVANCED_FACE ( 'NONE', ( #35441 ), #21254, .F. ) ;
#24699=ADVANCED_FACE ( 'NONE', ( #15554 ), #7032, .F. ) ;
#24706=CARTESIAN_POINT ( 'NONE',  ( -6.213268057914762998, 222.0587653132713228, -2.500000000000000000 ) ) ;
#24713=CARTESIAN_POINT ( 'NONE',  ( -28.15924032180904035, 205.9842294738515420, -6.938746391785683976 ) ) ;
#24715=AXIS2_PLACEMENT_3D ( 'NONE', #4632, #30426, #26492 ) ;
#24722=CARTESIAN_POINT ( 'NONE',  ( 23.87821517812500005, 246.8593750006145342, 4.985214923628404016 ) ) ;
#24724=CARTESIAN_POINT ( 'NONE',  ( 15.24356964374999990, 243.5593750006145228, 0.000000000000000000 ) ) ;
#24728=ADVANCED_FACE ( 'NONE', ( #11950 ), #36006, .F. ) ;
#24734=ORIENTED_EDGE ( 'NONE', *, *, #14549, .F. ) ;
#24737=VECTOR ( 'NONE', #34454, 1000.000000000000000 ) ;
#24741=DIRECTION ( 'NONE',  ( -0.000000000000000000, -1.000000000000000000, -0.000000000000000000 ) ) ;
#24742=CARTESIAN_POINT ( 'NONE',  ( 0.000000000000000000, 195.0000000000000000, -28.99999999999999645 ) ) ;
#24746=CARTESIAN_POINT ( 'NONE',  ( 20.99999999999999289, 243.6437500012290229, -5.999999999999997335 ) ) ;
#24747=CARTESIAN_POINT ( 'NONE',  ( 18.18132103106019315, 212.8186789689243881, 5.491377079899629976 ) ) ;
#24755=CARTESIAN_POINT ( 'NONE',  ( 27.24356964374999635, 196.4656250006145228, -15.72908226750539029 ) ) ;
#24758=ORIENTED_EDGE ( 'NONE', *, *, #32027, .T. ) ;
#24770=CARTESIAN_POINT ( 'NONE',  ( 18.00000000000000000, 246.3249999999999886, -5.196152422706630247 ) ) ;
#24779=EDGE_LOOP ( 'NONE', ( #25936, #12900, #17097, #12238, #30337, #25097 ) ) ;
#24783=CARTESIAN_POINT ( 'NONE',  ( 15.00000000000000000, 245.0499999999999829, 0.000000000000000000 ) ) ;
#24788=ORIENTED_EDGE ( 'NONE', *, *, #35521, .F. ) ;
#24790=CARTESIAN_POINT ( 'NONE',  ( 13.50000000000001421, 198.0125000012290286, 23.38268590217984055 ) ) ;
#24794=CARTESIAN_POINT ( 'NONE',  ( 23.87821517812499650, 244.3093750006145228, -4.985214923628404904 ) ) ;
#24801=CARTESIAN_POINT ( 'NONE',  ( 5.778771075727756162E-15, 198.6218750006145513, 31.45816453501075927 ) ) ;
#24805=DIRECTION ( 'NONE',  ( 0.000000000000000000, 0.000000000000000000, -1.000000000000000000 ) ) ;
#24816=CARTESIAN_POINT ( 'NONE',  ( 23.87821517812499650, 249.2593750006145399, -4.985214923628404904 ) ) ;
#24820=CARTESIAN_POINT ( 'NONE',  ( -13.62178482187500528, 196.6343750006145399, -23.59362340125807123 ) ) ;
#24823=CARTESIAN_POINT ( 'NONE',  ( 15.24356964374999990, 242.6593750006145171, 0.000000000000000000 ) ) ;
#24830=CARTESIAN_POINT ( 'NONE',  ( 23.87821517812500005, 244.9468750006145115, 4.985214923628404016 ) ) ;
#24836=EDGE_CURVE ( 'NONE', #2146, #28321, #2752, .T. ) ;
#24838=ORIENTED_EDGE ( 'NONE', *, *, #23044, .T. ) ;
#24845=CARTESIAN_POINT ( 'NONE',  ( 15.24356964374999990, 247.9468750006145115, 0.000000000000000000 ) ) ;
#24847=CARTESIAN_POINT ( 'NONE',  ( 24.00000000000000000, 240.2500000000000000, 5.196152422706629359 ) ) ;
#24850=EDGE_CURVE ( 'NONE', #2674, #13240, #4197, .T. ) ;
#24854=AXIS2_PLACEMENT_3D ( 'NONE', #7632, #2488, #36609 ) ;
#24855=CARTESIAN_POINT ( 'NONE',  ( 18.00000000000000000, 244.5250000000000057, -5.196152422706630247 ) ) ;
#24856=EDGE_CURVE ( 'NONE', #5512, #6657, #9354, .T. ) ;
#24864=DIRECTION ( 'NONE',  ( -0.000000000000000000, 1.000000000000000000, -0.000000000000000000 ) ) ;
#24868=CARTESIAN_POINT ( 'NONE',  ( 5.778771075727756162E-15, 198.6218750006145513, 31.45816453501075927 ) ) ;
#24870=CARTESIAN_POINT ( 'NONE',  ( 22.60769515458672885, 242.2174038105676459, -5.999999999999998224 ) ) ;
#24874=CARTESIAN_POINT ( 'NONE',  ( 26.99999999999999645, 240.3812500012290343, -7.347880794884117764E-16 ) ) ;
#24880=ADVANCED_FACE ( 'NONE', ( #809, #12380 ), #23950, .T. ) ;
#24901=EDGE_LOOP ( 'NONE', ( #31619, #32651 ) ) ;
#24903=CARTESIAN_POINT ( 'NONE',  ( -27.00000000000000355, 196.0250000012290457, -15.58845726811989429 ) ) ;
#24907=CARTESIAN_POINT ( 'NONE',  ( 21.00000000000000000, 247.8624999999999545, 5.999999999999998224 ) ) ;
#24908=CARTESIAN_POINT ( 'NONE',  ( 21.00000000000000000, 248.6218750006145228, 6.646953231504538984 ) ) ;
#24910=CARTESIAN_POINT ( 'NONE',  ( 20.99999999999999645, 243.2218750006145456, 6.646953231504538984 ) ) ;
#24921=VERTEX_POINT ( 'NONE', #18653 ) ;
#24925=CARTESIAN_POINT ( 'NONE',  ( 20.99999999999997868, 210.0000000000000000, -5.999999999999999112 ) ) ;
#24931=CARTESIAN_POINT ( 'NONE',  ( 14.89154389910932252, 216.1084561008947844, 0.4848545222723734671 ) ) ;
#24938=CARTESIAN_POINT ( 'NONE',  ( 27.24356964375000345, 195.5281250006145228, -3.336375036156643733E-15 ) ) ;
#24950=FACE_OUTER_BOUND ( 'NONE', #14457, .T. ) ;
#24958=CARTESIAN_POINT ( 'NONE',  ( 7.234628195640309123, 198.6299038117966802, -27.00000000000000711 ) ) ;
#24959=EDGE_LOOP ( 'NONE', ( #36042, #26035, #4826, #22489 ) ) ;
#24963=CARTESIAN_POINT ( 'NONE',  ( 15.00000000000000000, 243.6625000000000227, -3.464101615137752166 ) ) ;
#24964=DIRECTION ( 'NONE',  ( -1.000000000000000000, -4.130293990420971855E-17, 0.000000000000000000 ) ) ;
#24969=CARTESIAN_POINT ( 'NONE',  ( 13.50000000000001421, 199.3625000012290513, 23.38268590217984055 ) ) ;
#24970=CARTESIAN_POINT ( 'NONE',  ( 19.39230484541326760, 248.7986538117967541, 5.999999999999998224 ) ) ;
#24973=CARTESIAN_POINT ( 'NONE',  ( 23.87821517812500005, 246.4093750006145171, 4.985214923628404016 ) ) ;
#24980=CARTESIAN_POINT ( 'NONE',  ( -1.926257025242585782E-15, 197.4968750006145513, -31.45816453501075927 ) ) ;
#24986=EDGE_CURVE ( 'NONE', #10609, #9065, #8084, .T. ) ;
#24990=AXIS2_PLACEMENT_3D ( 'NONE', #394, #23530, #8249 ) ;
#25003=CARTESIAN_POINT ( 'NONE',  ( 27.24356964375000700, 198.6968750006145115, 15.72908226750537075 ) ) ;
#25007=CARTESIAN_POINT ( 'NONE',  ( 26.75643035624999655, 242.8843750006145115, -7.049594010296217766E-16 ) ) ;
#25008=FACE_OUTER_BOUND ( 'NONE', #3754, .T. ) ;
#25012=ORIENTED_EDGE ( 'NONE', *, *, #23303, .F. ) ;
#25014=AXIS2_PLACEMENT_3D ( 'NONE', #18857, #30405, #13154 ) ;
#25015=CARTESIAN_POINT ( 'NONE',  ( 15.24356964374999990, 243.4093750006145171, -3.323476615752268604 ) ) ;
#25022=VERTEX_POINT ( 'NONE', #1562 ) ;
#25027=CARTESIAN_POINT ( 'NONE',  ( 26.75643035624999655, 243.6343750006144830, 3.323476615752267271 ) ) ;
#25032=ORIENTED_EDGE ( 'NONE', *, *, #11222, .F. ) ;
#25036=CARTESIAN_POINT ( 'NONE',  ( 1.069080835302379631E-14, 199.6625000000000227, 27.00000000000000000 ) ) ;
#25046=( BOUNDED_CURVE ( )  B_SPLINE_CURVE ( 2, ( #15302, #32729, #1074, #26855, #14740, #321, #693, #32915, #12073 ),
 .UNSPECIFIED., .F., .F. ) 
 B_SPLINE_CURVE_WITH_KNOTS ( ( 3, 2, 2, 2, 3 ),
 ( 0.4673913043478261087, 0.4710144927536231707, 0.4782608695652174058, 0.4855072463768115854, 0.4891304347826087029 ),
 .UNSPECIFIED. ) 
 CURVE ( )  GEOMETRIC_REPRESENTATION_ITEM ( )  RATIONAL_B_SPLINE_CURVE ( ( 0.9330127018922194093, 0.9330127018922198534, 1.000000000000000000, 0.8660254037844387076, 1.000000000000000000, 0.8660254037844387076, 1.000000000000000000, 0.9330127018922194093, 0.9330127018922194093 ) ) 
 REPRESENTATION_ITEM ( '' )  );
#25051=CARTESIAN_POINT ( 'NONE',  ( 13.62178482187501416, 198.2093750006145285, 23.59362340125806767 ) ) ;
#25053=AXIS2_PLACEMENT_3D ( 'NONE', #16073, #35957, #32742 ) ;
#25054=CARTESIAN_POINT ( 'NONE',  ( 0.000000000000000000, 202.0000000000000000, 0.000000000000000000 ) ) ;
#25058=CARTESIAN_POINT ( 'NONE',  ( 26.99999999999999645, 241.7687500012290229, -3.464101615137755275 ) ) ;
#25061=CARTESIAN_POINT ( 'NONE',  ( -27.24356964374999635, 198.0406250006145399, 15.72908226750539384 ) ) ;
#25064=EDGE_LOOP ( 'NONE', ( #28503, #19786, #19987, #23181 ) ) ;
#25085=CARTESIAN_POINT ( 'NONE',  ( -28.01712176579047764, 207.1685799127409382, -7.486769987355970102 ) ) ;
#25090=DIRECTION ( 'NONE',  ( 0.000000000000000000, 0.000000000000000000, -1.000000000000000000 ) ) ;
#25091=CARTESIAN_POINT ( 'NONE',  ( 27.00000000000001421, 195.3500000012290343, 15.58845726811988897 ) ) ;
#25094=CARTESIAN_POINT ( 'NONE',  ( 21.00000000000000000, 248.1718750006145342, 6.646953231504538984 ) ) ;
#25096=CARTESIAN_POINT ( 'NONE',  ( 18.12178482187499640, 245.2843750006145456, -4.985214923628404904 ) ) ;
#25097=ORIENTED_EDGE ( 'NONE', *, *, #2962, .F. ) ;
#25099=CARTESIAN_POINT ( 'NONE',  ( 21.00000000000000000, 248.1437500012290513, -6.928203230275506996 ) ) ;
#25105=ADVANCED_FACE ( 'NONE', ( #33411 ), #5404, .T. ) ;
#25108=ORIENTED_EDGE ( 'NONE', *, *, #13141, .T. ) ;
#25114=CARTESIAN_POINT ( 'NONE',  ( 26.75643035624999655, 248.5843750006145001, 3.323476615752267715 ) ) ;
#25119=CARTESIAN_POINT ( 'NONE',  ( 5.409584567222309737, 215.8464057872915305, 1.363118671454217390 ) ) ;
#25126=ADVANCED_FACE ( 'NONE', ( #26641 ), #29106, .F. ) ;
#25128=CARTESIAN_POINT ( 'NONE',  ( 27.24356964375000700, 196.3906250006145058, 15.72908226750537075 ) ) ;
#25145=CARTESIAN_POINT ( 'NONE',  ( -13.50000000000000533, 198.6875000012290400, -23.38268590217984411 ) ) ;
#25147=CARTESIAN_POINT ( 'NONE',  ( 5.727106289114498080E-15, 197.4124999999999943, 31.17691453623979214 ) ) ;
#25158=CARTESIAN_POINT ( 'NONE',  ( 26.99999999999999645, 243.9250000000000114, -7.347880794884117764E-16 ) ) ;
#25163=ORIENTED_EDGE ( 'NONE', *, *, #22903, .F. ) ;
#25164=CARTESIAN_POINT ( 'NONE',  ( 27.00000000000001066, 197.1500000012290172, 15.58845726811988897 ) ) ;
#25166=EDGE_CURVE ( 'NONE', #13240, #30190, #23576, .T. ) ;
#25171=CARTESIAN_POINT ( 'NONE',  ( 26.75643035624999655, 242.4343750006145513, -7.049594010296217766E-16 ) ) ;
#25178=CARTESIAN_POINT ( 'NONE',  ( 27.24356964375000345, 198.2843750006145456, -3.336375036156643733E-15 ) ) ;
#25193=CARTESIAN_POINT ( 'NONE',  ( 26.99999999999999645, 240.3437500012290116, 3.464101615137751278 ) ) ;
#25197=CARTESIAN_POINT ( 'NONE',  ( 27.24356964375000700, 197.7968750006145342, 15.72908226750537075 ) ) ;
#25200=CARTESIAN_POINT ( 'NONE',  ( 2.999999999999997335, 244.5000000000000000, -2.500000000000000000 ) ) ;
#25201=CARTESIAN_POINT ( 'NONE',  ( 15.00000000000000178, 249.5875000000000341, 3.464101615137757051 ) ) ;
#25207=CARTESIAN_POINT ( 'NONE',  ( 26.75643035624999655, 244.0843750006145285, 3.323476615752267715 ) ) ;
#25221=CARTESIAN_POINT ( 'NONE',  ( 26.75643035624999655, 245.5093750006145115, -3.323476615752271268 ) ) ;
#25228=CARTESIAN_POINT ( 'NONE',  ( 18.00000000000000355, 244.6750000000000114, 5.196152422706632912 ) ) ;
#25230=CIRCLE ( 'NONE', #8888, 28.99999999999999645 ) ;
#25234=ORIENTED_EDGE ( 'NONE', *, *, #1109, .T. ) ;
#25239=CARTESIAN_POINT ( 'NONE',  ( -27.24356964374999990, 198.9218750006145626, -15.72908226750537786 ) ) ;
#25247=CARTESIAN_POINT ( 'NONE',  ( 26.99999999999999645, 240.8687500012290457, -3.464101615137755275 ) ) ;
#25250=CARTESIAN_POINT ( 'NONE',  ( 13.62178482187501416, 198.6031250006145399, 23.59362340125806767 ) ) ;
#25258=DIRECTION ( 'NONE',  ( 0.000000000000000000, 1.000000000000000000, 0.000000000000000000 ) ) ;
#25261=CYLINDRICAL_SURFACE ( 'NONE', #12543, 5.999999999999999112 ) ;
#25269=PRODUCT_DEFINITION_SHAPE ( 'NONE', 'NONE',  #33139 ) ;
#25274=CARTESIAN_POINT ( 'NONE',  ( 13.50000000000001421, 198.9125000012290343, 23.38268590217984055 ) ) ;
#25275=EDGE_LOOP ( 'NONE', ( #20512, #5851, #27445, #10038 ) ) ;
#25280=( LENGTH_UNIT ( ) NAMED_UNIT ( * ) SI_UNIT ( .MILLI., .METRE. ) );
#25283=CARTESIAN_POINT ( 'NONE',  ( 21.00000000000000000, 247.2718750006145569, 6.646953231504538984 ) ) ;
#25285=CARTESIAN_POINT ( 'NONE',  ( 23.87821517812500005, 242.3593750006145342, 4.985214923628404016 ) ) ;
#25288=CARTESIAN_POINT ( 'NONE',  ( 15.00000000000000000, 247.7687500012291082, -3.464101615137752166 ) ) ;
#25299=DIRECTION ( 'NONE',  ( 0.000000000000000000, 0.000000000000000000, 1.000000000000000000 ) ) ;
#25301=CARTESIAN_POINT ( 'NONE',  ( 26.75643035624999655, 249.5218750006145001, -7.049594010296217766E-16 ) ) ;
#25304=CARTESIAN_POINT ( 'NONE',  ( 14.99999999999999822, 225.9999999999999716, 0.1963495407219037481 ) ) ;
#25306=FACE_OUTER_BOUND ( 'NONE', #14848, .T. ) ;
#25312=CARTESIAN_POINT ( 'NONE',  ( 27.24356964374999635, 195.5656250006145171, -15.72908226750539029 ) ) ;
#25316=ORIENTED_EDGE ( 'NONE', *, *, #17995, .T. ) ;
#25332=CARTESIAN_POINT ( 'NONE',  ( 13.50000000000001421, 197.4500000000000171, 23.38268590217984055 ) ) ;
#25334=LINE ( 'NONE', #22315, #23846 ) ;
#25337=CARTESIAN_POINT ( 'NONE',  ( 15.24356964374999990, 249.8218750006145399, -3.323476615752268604 ) ) ;
#25338=VERTEX_POINT ( 'NONE', #18321 ) ;
#25344=CARTESIAN_POINT ( 'NONE',  ( 26.99999999999999645, 244.4124999999999943, -3.464101615137755275 ) ) ;
#25346=EDGE_CURVE ( 'NONE', #7130, #30424, #11940, .T. ) ;
#25347=( BOUNDED_CURVE ( )  B_SPLINE_CURVE ( 2, ( #8047, #28313, #19623, #5192, #10506 ),
 .UNSPECIFIED., .F., .F. ) 
 B_SPLINE_CURVE_WITH_KNOTS ( ( 3, 2, 3 ),
 ( 0.000000000000000000, 0.01388888888888888985, 0.02083333333333333565 ),
 .UNSPECIFIED. ) 
 CURVE ( )  GEOMETRIC_REPRESENTATION_ITEM ( )  RATIONAL_B_SPLINE_CURVE ( ( 1.000000000000000000, 0.8660254037844387076, 1.000000000000000000, 0.9330127018922192983, 0.9330127018922194093 ) ) 
 REPRESENTATION_ITEM ( '' )  );
#25350=ORIENTED_EDGE ( 'NONE', *, *, #29030, .F. ) ;
#25351=CARTESIAN_POINT ( 'NONE',  ( 27.00000000000000355, 195.3875000012290286, -3.306546357697854128E-15 ) ) ;
#25355=CARTESIAN_POINT ( 'NONE',  ( 15.24356964375000167, 243.5968750006144887, 3.323476615752272600 ) ) ;
#25357=CARTESIAN_POINT ( 'NONE',  ( 20.00041209925370467, 239.8223985277589918, -5.668978256696592055 ) ) ;
#25361=CARTESIAN_POINT ( 'NONE',  ( 27.24356964374999635, 198.3218750006145399, -15.72908226750539029 ) ) ;
#25364=DIRECTION ( 'NONE',  ( -0.000000000000000000, -1.000000000000000000, -0.000000000000000000 ) ) ;
#25374=CARTESIAN_POINT ( 'NONE',  ( 1.069080835302379631E-14, 199.6625000000000227, 27.00000000000000000 ) ) ;
#25375=LINE ( 'NONE', #16860, #9538 ) ;
#25376=VERTEX_POINT ( 'NONE', #7133 ) ;
#25379=CARTESIAN_POINT ( 'NONE',  ( 5.778771075727756162E-15, 196.8218750006145683, 31.45816453501076637 ) ) ;
#25384=CARTESIAN_POINT ( 'NONE',  ( 15.24356964374999990, 240.3718750006145228, -3.323476615752268604 ) ) ;
#25385=DIRECTION ( 'NONE',  ( 0.000000000000000000, -1.000000000000000000, 0.000000000000000000 ) ) ;
#25390=CARTESIAN_POINT ( 'NONE',  ( 15.24356964375000167, 245.7343750006145058, 3.323476615752272600 ) ) ;
#25403=CARTESIAN_POINT ( 'NONE',  ( 26.75643035624999655, 244.6093750006145342, -3.323476615752271268 ) ) ;
#25404=CARTESIAN_POINT ( 'NONE',  ( 22.60769515458672885, 240.4174038105676630, -5.999999999999998224 ) ) ;
#25410=CARTESIAN_POINT ( 'NONE',  ( -7.234628195640307347, 199.4575961894323370, -27.00000000000000711 ) ) ;
#25420=DIRECTION ( 'NONE',  ( 0.000000000000000000, 0.000000000000000000, 1.000000000000000000 ) ) ;
#25424=CARTESIAN_POINT ( 'NONE',  ( 20.99999999999999289, 242.2937500012290570, -5.999999999999997335 ) ) ;
#25425=CARTESIAN_POINT ( 'NONE',  ( -13.62178482187500528, 195.7343750006145626, -23.59362340125807123 ) ) ;
#25431=CARTESIAN_POINT ( 'NONE',  ( 15.00000000000000178, 240.6437500012290513, 3.464101615137757051 ) ) ;
#25432=AXIS2_PLACEMENT_3D ( 'NONE', #5330, #14245, #11207 ) ;
#25437=ORIENTED_EDGE ( 'NONE', *, *, #1321, .T. ) ;
#25444=EDGE_CURVE ( 'NONE', #23659, #8033, #21150, .T. ) ;
#25455=ADVANCED_FACE ( 'NONE', ( #1425 ), #1987, .F. ) ;
#25458=CARTESIAN_POINT ( 'NONE',  ( 20.99999999999998579, 247.9187500012290002, 5.999999999999998224 ) ) ;
#25465=DIRECTION ( 'NONE',  ( -0.000000000000000000, -1.000000000000000000, -0.000000000000000000 ) ) ;
#25468=CARTESIAN_POINT ( 'NONE',  ( 18.12178482187499640, 246.6343750006145115, -4.985214923628404904 ) ) ;
#25470=CARTESIAN_POINT ( 'NONE',  ( 15.24356964374999990, 242.6593750006145171, 0.000000000000000000 ) ) ;
#25473=CARTESIAN_POINT ( 'NONE',  ( 15.00000000000000000, 249.5687500012290343, -3.464101615137752166 ) ) ;
#25479=EDGE_LOOP ( 'NONE', ( #35824, #5500, #4433, #27562 ) ) ;
#25480=VERTEX_POINT ( 'NONE', #21909 ) ;
#25484=CARTESIAN_POINT ( 'NONE',  ( 15.00000000000000000, 241.9562500012290513, 0.000000000000000000 ) ) ;
#25485=DIRECTION ( 'NONE',  ( -1.000000000000000000, -4.130293990420971855E-17, 0.000000000000000000 ) ) ;
#25486=CARTESIAN_POINT ( 'NONE',  ( 15.24356964374999990, 249.7093750006145285, -3.323476615752268604 ) ) ;
#25489=CARTESIAN_POINT ( 'NONE',  ( 6.418300056333629655, 215.4681374788749793, -2.477503916095892489 ) ) ;
#25498=VECTOR ( 'NONE', #9099, 1000.000000000000227 ) ;
#25499=CARTESIAN_POINT ( 'NONE',  ( -1.926257025242585782E-15, 195.1906250006145456, -31.45816453501075927 ) ) ;
#25515=CARTESIAN_POINT ( 'NONE',  ( 27.00000000000001066, 197.0374999999999943, 15.58845726811988897 ) ) ;
#25519=CARTESIAN_POINT ( 'NONE',  ( 15.24356964374999990, 249.4093750006145171, 0.000000000000000000 ) ) ;
#25520=ORIENTED_EDGE ( 'NONE', *, *, #8449, .F. ) ;
#25527=CARTESIAN_POINT ( 'NONE',  ( 21.00000000000000000, 243.1374999999999886, -6.928203230275506996 ) ) ;
#25530=VERTEX_POINT ( 'NONE', #7499 ) ;
#25531=VERTEX_POINT ( 'NONE', #19075 ) ;
#25533=CARTESIAN_POINT ( 'NONE',  ( -27.00000000000000355, 195.1250000012290400, -15.58845726811989429 ) ) ;
#25537=CARTESIAN_POINT ( 'NONE',  ( 21.00000000000000000, 241.8718750006145228, 6.646953231504538984 ) ) ;
#25545=CARTESIAN_POINT ( 'NONE',  ( -27.24356964374999635, 198.5468750006145626, 15.72908226750539384 ) ) ;
#25549=CARTESIAN_POINT ( 'NONE',  ( 1.069080835302379631E-14, 198.7624999999999886, 27.00000000000000000 ) ) ;
#25554=CARTESIAN_POINT ( 'NONE',  ( 13.49999999999999645, 197.2625000012290286, -23.38268590217984766 ) ) ;
#25559=CARTESIAN_POINT ( 'NONE',  ( 22.60769515458673240, 248.7825961894322973, 6.000000000000000000 ) ) ;
#25560=LINE ( 'NONE', #22733, #30730 ) ;
#25564=DIRECTION ( 'NONE',  ( 0.000000000000000000, 0.000000000000000000, 1.000000000000000000 ) ) ;
#25568=CARTESIAN_POINT ( 'NONE',  ( 21.00000000000000000, 240.2968750006145342, -6.646953231504538984 ) ) ;
#25569=CARTESIAN_POINT ( 'NONE',  ( 27.24356964374999279, 198.7156250006145513, -15.72908226750539207 ) ) ;
#25574=CARTESIAN_POINT ( 'NONE',  ( 15.24356964374999990, 241.1968750006145115, 0.000000000000000000 ) ) ;
#25578=CARTESIAN_POINT ( 'NONE',  ( 23.99999999999999645, 244.4499999999999886, -5.196152422706631135 ) ) ;
#25579=EDGE_CURVE ( 'NONE', #2118, #36527, #6633, .T. ) ;
#25586=CARTESIAN_POINT ( 'NONE',  ( 15.24356964375000167, 243.9343750006145228, 3.323476615752272600 ) ) ;
#25597=CARTESIAN_POINT ( 'NONE',  ( 26.99999999999999645, 244.3937500012290513, 3.464101615137751278 ) ) ;
#25602=ORIENTED_EDGE ( 'NONE', *, *, #7834, .F. ) ;
#25608=CARTESIAN_POINT ( 'NONE',  ( -1.926257025242585782E-15, 195.6968750006145683, -31.45816453501075927 ) ) ;
#25614=CARTESIAN_POINT ( 'NONE',  ( 15.00000000000000000, 241.0562500012290457, 0.000000000000000000 ) ) ;
#25639=VECTOR ( 'NONE', #16956, 1000.000000000000000 ) ;
#25642=ORIENTED_EDGE ( 'NONE', *, *, #36458, .F. ) ;
#25644=CARTESIAN_POINT ( 'NONE',  ( -7.234628195640354420, 196.1549038117966859, 26.99999999999996803 ) ) ;
#25647=FACE_OUTER_BOUND ( 'NONE', #37084, .T. ) ;
#25648=CARTESIAN_POINT ( 'NONE',  ( 26.99999999999999645, 246.2687500012290513, -3.464101615137755275 ) ) ;
#25650=CARTESIAN_POINT ( 'NONE',  ( 18.12178482187499640, 244.3843750006145115, -4.985214923628404904 ) ) ;
#25652=CARTESIAN_POINT ( 'NONE',  ( 20.99999999999999645, 241.4218750006145626, 6.646953231504538984 ) ) ;
#25656=CARTESIAN_POINT ( 'NONE',  ( 26.99999999999999645, 248.0687500012290343, -3.464101615137755275 ) ) ;
#25664=ORIENTED_EDGE ( 'NONE', *, *, #27143, .F. ) ;
#25665=ORIENTED_EDGE ( 'NONE', *, *, #13511, .T. ) ;
#25670=PRODUCT_DEFINITION_FORMATION_WITH_SPECIFIED_SOURCE ( 'ANY', '', #28915, .NOT_KNOWN. ) ;
#25672=CARTESIAN_POINT ( 'NONE',  ( 21.00000000000000000, 249.4093750006145171, 6.646953231504538984 ) ) ;
#25678=CARTESIAN_POINT ( 'NONE',  ( 5.409584567223228113, 215.8464057872915589, -1.363118671453956265 ) ) ;
#25685=EDGE_CURVE ( 'NONE', #28635, #9537, #31181, .T. ) ;
#25702=CARTESIAN_POINT ( 'NONE',  ( -26.99999999999998934, 198.2374999999999829, 15.58845726811991561 ) ) ;
#25703=DIRECTION ( 'NONE',  ( -0.000000000000000000, 1.000000000000000000, -0.000000000000000000 ) ) ;
#25712=CARTESIAN_POINT ( 'NONE',  ( 21.00000000000000000, 244.7125000000000057, 6.928203230275506996 ) ) ;
#25716=ORIENTED_EDGE ( 'NONE', *, *, #4108, .T. ) ;
#25718=CARTESIAN_POINT ( 'NONE',  ( 5.727106289114498080E-15, 196.1750000012290513, 31.17691453623979214 ) ) ;
#25723=CARTESIAN_POINT ( 'NONE',  ( 26.75643035624999655, 243.3343750006145285, -7.049594010296217766E-16 ) ) ;
#25725=CYLINDRICAL_SURFACE ( 'NONE', #26429, 2.649999999999991029 ) ;
#25731=CARTESIAN_POINT ( 'NONE',  ( 23.27690126865536158, 194.9999999999999716, -13.80801991767920534 ) ) ;
#25732=CARTESIAN_POINT ( 'NONE',  ( 13.62178482187501416, 195.9593750006145569, 23.59362340125806767 ) ) ;
#25736=CARTESIAN_POINT ( 'NONE',  ( 15.00000000000000000, 240.5124999999999602, -3.464101615137752610 ) ) ;
#25737=LINE ( 'NONE', #22534, #24737 ) ;
#25743=CARTESIAN_POINT ( 'NONE',  ( 15.00000000000000000, 249.5124999999999602, -3.464101615137752610 ) ) ;
#25745=CARTESIAN_POINT ( 'NONE',  ( 22.60769515458672885, 240.4736538117967086, -5.999999999999998224 ) ) ;
#25749=CARTESIAN_POINT ( 'NONE',  ( 20.99999999999999645, 185.0294372515228645, -5.999999999999999112 ) ) ;
#25752=DIRECTION ( 'NONE',  ( 0.000000000000000000, 1.000000000000000000, 0.000000000000000000 ) ) ;
#25753=CARTESIAN_POINT ( 'NONE',  ( 18.00000000000000355, 249.6250000000000000, 5.196152422706632912 ) ) ;
#25754=CARTESIAN_POINT ( 'NONE',  ( 13.62178482187499640, 197.8531250006145399, -23.59362340125807123 ) ) ;
#25760=CARTESIAN_POINT ( 'NONE',  ( 21.00000000000000000, 242.4343750006145228, -6.646953231504538984 ) ) ;
#25769=CARTESIAN_POINT ( 'NONE',  ( 23.87821517812500005, 243.5968750006145171, 4.985214923628404016 ) ) ;
#25774=AXIS2_PLACEMENT_3D ( 'NONE', #2295, #13687, #16340 ) ;
#25784=ADVANCED_FACE ( 'NONE', ( #5203 ), #13753, .F. ) ;
#25791=CYLINDRICAL_SURFACE ( 'NONE', #20803, 5.999999999999999112 ) ;
#25792=CARTESIAN_POINT ( 'NONE',  ( -27.24356964374999990, 195.7718750006145569, -15.72908226750537786 ) ) ;
#25793=CARTESIAN_POINT ( 'NONE',  ( 8.433054386417008885, 195.0000000000000284, 25.92026892250748205 ) ) ;
#25799=CARTESIAN_POINT ( 'NONE',  ( 15.24356964374999990, 248.8468750006145171, 0.000000000000000000 ) ) ;
#25805=VECTOR ( 'NONE', #2613, 1000.000000000000000 ) ;
#25812=DIRECTION ( 'NONE',  ( -0.000000000000000000, 1.000000000000000000, -0.000000000000000000 ) ) ;
#25815=CARTESIAN_POINT ( 'NONE',  ( -22.11840882573491740, 195.0000000000000284, 15.80876310588338463 ) ) ;
#25819=ORIENTED_EDGE ( 'NONE', *, *, #3801, .F. ) ;
#25821=CARTESIAN_POINT ( 'NONE',  ( 11.62741699796951345, 213.5147186257614180, -6.000000000000000000 ) ) ;
#25834=DIRECTION ( 'NONE',  ( 0.000000000000000000, 0.000000000000000000, -1.000000000000000000 ) ) ;
#25835=CARTESIAN_POINT ( 'NONE',  ( 26.75643035624999655, 246.4468750006144830, 3.323476615752267715 ) ) ;
#25837=CARTESIAN_POINT ( 'NONE',  ( 26.75643035624999655, 241.9843750006145342, -7.049594010296217766E-16 ) ) ;
#25840=CARTESIAN_POINT ( 'NONE',  ( 1.069080835302379631E-14, 198.3124999999999716, 27.00000000000000000 ) ) ;
#25842=CARTESIAN_POINT ( 'NONE',  ( 26.99999999999999645, 245.3687500012290457, -3.464101615137755275 ) ) ;
#25853=ORIENTED_EDGE ( 'NONE', *, *, #11660, .F. ) ;
#25856=CARTESIAN_POINT ( 'NONE',  ( 26.75643035624999655, 245.9593750006145001, -3.323476615752271712 ) ) ;
#25886=CARTESIAN_POINT ( 'NONE',  ( -27.00000000000000355, 197.7125000000000057, -15.58845726811989429 ) ) ;
#25890=VERTEX_POINT ( 'NONE', #8983 ) ;
#25897=CARTESIAN_POINT ( 'NONE',  ( 24.00000000000000000, 240.6999999999999886, 5.196152422706629359 ) ) ;
#25904=CARTESIAN_POINT ( 'NONE',  ( -1.909035429704832693E-15, 196.8500000012290343, -31.17691453623979214 ) ) ;
#25906=VECTOR ( 'NONE', #18105, 1000.000000000000000 ) ;
#25909=CARTESIAN_POINT ( 'NONE',  ( 23.87821517812499650, 241.1593750006145171, -4.985214923628404904 ) ) ;
#25910=VECTOR ( 'NONE', #567, 1000.000000000000000 ) ;
#25912=CARTESIAN_POINT ( 'NONE',  ( 19.39230484541326760, 242.9486538117967029, 5.999999999999999112 ) ) ;
#25917=CARTESIAN_POINT ( 'NONE',  ( 26.58413874528002907, 195.0000000000000000, -5.631313390073841241 ) ) ;
#25918=CARTESIAN_POINT ( 'NONE',  ( 5.778771075727756162E-15, 196.3718750006145513, 31.45816453501075927 ) ) ;
#25924=CARTESIAN_POINT ( 'NONE',  ( 15.00000000000000000, 247.2624999999999886, -3.464101615137752610 ) ) ;
#25936=ORIENTED_EDGE ( 'NONE', *, *, #10728, .F. ) ;
#25939=CARTESIAN_POINT ( 'NONE',  ( 13.62178482187501416, 195.0593750006145513, 23.59362340125806767 ) ) ;
#25942=CARTESIAN_POINT ( 'NONE',  ( -26.99999999999999645, 198.2375000000000114, 15.58845726811991561 ) ) ;
#25943=CARTESIAN_POINT ( 'NONE',  ( 15.24356964374999990, 240.8593750006145342, 0.000000000000000000 ) ) ;
#25944=CARTESIAN_POINT ( 'NONE',  ( 13.62178482187501416, 199.5031250006145456, 23.59362340125806767 ) ) ;
#25949=CARTESIAN_POINT ( 'NONE',  ( 13.62178482187499640, 199.2031250006145342, -23.59362340125807123 ) ) ;
#25950=CARTESIAN_POINT ( 'NONE',  ( 21.00000000000000000, 243.1093750006145058, 6.646953231504538984 ) ) ;
#25958=CARTESIAN_POINT ( 'NONE',  ( 23.87821517812499650, 241.0468750006145058, -4.985214923628404904 ) ) ;
#25965=CARTESIAN_POINT ( 'NONE',  ( 20.99999999999999645, 240.2125000000000057, 5.999999999999998224 ) ) ;
#25969=CARTESIAN_POINT ( 'NONE',  ( 15.00000000000000178, 241.5437500012290570, 3.464101615137757051 ) ) ;
#25976=( BOUNDED_CURVE ( )  B_SPLINE_CURVE ( 2, ( #21665, #16535, #33777, #21852, #18832, #10648, #1745, #33404, #36607 ),
 .UNSPECIFIED., .F., .F. ) 
 B_SPLINE_CURVE_WITH_KNOTS ( ( 3, 2, 2, 2, 3 ),
 ( 0.5760869565217391353, 0.5797101449275362528, 0.5869565217391304879, 0.5942028985507246119, 0.5978260869565217295 ),
 .UNSPECIFIED. ) 
 CURVE ( )  GEOMETRIC_REPRESENTATION_ITEM ( )  RATIONAL_B_SPLINE_CURVE ( ( 0.9330127018922194093, 0.9330127018922194093, 1.000000000000000000, 0.8660254037844387076, 1.000000000000000000, 0.8660254037844387076, 1.000000000000000000, 0.9330127018922194093, 0.9330127018922194093 ) ) 
 REPRESENTATION_ITEM ( '' )  );
#25978=CARTESIAN_POINT ( 'NONE',  ( -1.926257025242585782E-15, 196.5968750006145456, -31.45816453501075927 ) ) ;
#25985=ORIENTED_EDGE ( 'NONE', *, *, #37470, .T. ) ;
#25986=CARTESIAN_POINT ( 'NONE',  ( 26.99999999999999645, 240.3437500012290400, 3.464101615137751278 ) ) ;
#25996=( BOUNDED_CURVE ( )  B_SPLINE_CURVE ( 2, ( #18243, #29787, #26563, #35845, #3818, #9141, #15011, #29214, #17677 ),
 .UNSPECIFIED., .F., .F. ) 
 B_SPLINE_CURVE_WITH_KNOTS ( ( 3, 2, 2, 2, 3 ),
 ( 0.7500000000000000000, 0.7536231884057971175, 0.7608695652173913526, 0.7681159420289854767, 0.7717391304347825942 ),
 .UNSPECIFIED. ) 
 CURVE ( )  GEOMETRIC_REPRESENTATION_ITEM ( )  RATIONAL_B_SPLINE_CURVE ( ( 0.9330127018922194093, 0.9330127018922194093, 1.000000000000000000, 0.8660254037844387076, 1.000000000000000000, 0.8660254037844387076, 1.000000000000000000, 0.9330127018922194093, 0.9330127018922194093 ) ) 
 REPRESENTATION_ITEM ( '' )  );
#25998=CARTESIAN_POINT ( 'NONE',  ( 26.75643035624999655, 248.2093750006145285, -3.323476615752271268 ) ) ;
#26000=CARTESIAN_POINT ( 'NONE',  ( -18.43413144353408484, 194.9999999999999432, 19.99507324645828277 ) ) ;
#26018=CARTESIAN_POINT ( 'NONE',  ( 13.49999999999999645, 197.5999999999999943, -23.38268590217984766 ) ) ;
#26020=CARTESIAN_POINT ( 'NONE',  ( 23.87821517812500005, 245.5093750006145399, 4.985214923628404016 ) ) ;
#26023=EDGE_LOOP ( 'NONE', ( #37376, #25437, #34177, #32469 ) ) ;
#26025=DIRECTION ( 'NONE',  ( 0.000000000000000000, 1.000000000000000000, 0.000000000000000000 ) ) ;
#26026=CARTESIAN_POINT ( 'NONE',  ( 24.00000000000000000, 246.1562500012290400, 5.196152422706629359 ) ) ;
#26035=ORIENTED_EDGE ( 'NONE', *, *, #36935, .T. ) ;
#26042=CARTESIAN_POINT ( 'NONE',  ( 21.00000000000000000, 247.8343750006144717, -6.646953231504538984 ) ) ;
#26046=CARTESIAN_POINT ( 'NONE',  ( 16.34449471653107011, 214.6555052834990818, -4.429144169343526727 ) ) ;
#26060=CARTESIAN_POINT ( 'NONE',  ( 19.39230484541323918, 243.1575961894323541, -5.999999999999987566 ) ) ;
#26065=EDGE_CURVE ( 'NONE', #6301, #12071, #35183, .T. ) ;
#26067=LINE ( 'NONE', #20397, #13440 ) ;
#26071=CARTESIAN_POINT ( 'NONE',  ( 27.24356964375000700, 199.5968750006145456, 15.72908226750537075 ) ) ;
#26074=CARTESIAN_POINT ( 'NONE',  ( 23.87821517812499650, 247.9093750006145171, -4.985214923628404904 ) ) ;
#26081=CARTESIAN_POINT ( 'NONE',  ( 15.00000000000000178, 241.4874999999999829, 3.464101615137757051 ) ) ;
#26084=ORIENTED_EDGE ( 'NONE', *, *, #8485, .T. ) ;
#26087=CARTESIAN_POINT ( 'NONE',  ( -1.909035429704832693E-15, 195.0500000012290229, -31.17691453623979214 ) ) ;
#26092=CARTESIAN_POINT ( 'NONE',  ( 15.24356964374999990, 240.4093750006145456, 0.000000000000000000 ) ) ;
#26095=DIRECTION ( 'NONE',  ( -0.000000000000000000, 1.000000000000000000, -0.000000000000000000 ) ) ;
#26101=CARTESIAN_POINT ( 'NONE',  ( -27.24356964375000345, 194.9093750006145456, 0.000000000000000000 ) ) ;
#26103=EDGE_LOOP ( 'NONE', ( #20714, #34914, #20336, #14449, #11606, #17488 ) ) ;
#26112=CARTESIAN_POINT ( 'NONE',  ( 20.99999999999999645, 249.6625000000000512, 5.999999999999998224 ) ) ;
#26113=FACE_OUTER_BOUND ( 'NONE', #30049, .T. ) ;
#26120=CARTESIAN_POINT ( 'NONE',  ( 27.24356964375000700, 195.0968750006145456, 15.72908226750537075 ) ) ;
#26124=CARTESIAN_POINT ( 'NONE',  ( 26.99999999999999645, 248.8750000000000000, -7.347880794884117764E-16 ) ) ;
#26125=CARTESIAN_POINT ( 'NONE',  ( -27.24356964374999279, 198.9406250006145171, 15.72908226750539384 ) ) ;
#26128=ORIENTED_EDGE ( 'NONE', *, *, #8236, .F. ) ;
#26130=B_SPLINE_CURVE_WITH_KNOTS ( 'NONE', 3,
 ( #15112, #29318, #884, #29696, #29125, #6393, #18340, #17775 ),
 .UNSPECIFIED., .F., .F.,
 ( 4, 2, 2, 4 ),
 ( 0.000000000000000000, 0.002520245793383945297, 0.003780368690075958278, 0.005040491586767971259 ),
 .UNSPECIFIED. ) ;
#26131=CARTESIAN_POINT ( 'NONE',  ( 27.24356964375000700, 199.0906250006145228, 15.72908226750537075 ) ) ;
#26132=CARTESIAN_POINT ( 'NONE',  ( 21.00000000000000000, 241.7593750006145115, 6.646953231504538984 ) ) ;
#26135=CARTESIAN_POINT ( 'NONE',  ( 21.00000000000000000, 247.0468750006145058, -6.646953231504538984 ) ) ;
#26141=CARTESIAN_POINT ( 'NONE',  ( 20.99999999999999645, 242.6593750006145171, 6.646953231504538984 ) ) ;
#26149=CARTESIAN_POINT ( 'NONE',  ( -27.00000000000000355, 198.7250000012290343, -15.58845726811989429 ) ) ;
#26156=CARTESIAN_POINT ( 'NONE',  ( 15.24356964374999990, 242.0593750006145513, -3.323476615752268604 ) ) ;
#26161=CARTESIAN_POINT ( 'NONE',  ( 20.99999999999999645, 247.8624999999999545, 5.999999999999998224 ) ) ;
#26162=CARTESIAN_POINT ( 'NONE',  ( 2.999999999999997335, 244.5000000000000000, 5.000000000000000000 ) ) ;
#26163=CARTESIAN_POINT ( 'NONE',  ( 27.24356964375000700, 195.9968750006145513, 15.72908226750537075 ) ) ;
#26164=CARTESIAN_POINT ( 'NONE',  ( 3.306246199927494800, 194.9999999999999716, 27.04578575729343726 ) ) ;
#26165=CARTESIAN_POINT ( 'NONE',  ( -27.00000000000000355, 196.9250000012290229, -15.58845726811989429 ) ) ;
#26170=CARTESIAN_POINT ( 'NONE',  ( 26.99999999999999645, 239.9687500012290684, -3.464101615137755275 ) ) ;
#26180=CARTESIAN_POINT ( 'NONE',  ( 23.87821517812499650, 248.6968750006145115, -4.985214923628404904 ) ) ;
#26181=CARTESIAN_POINT ( 'NONE',  ( -26.74238012849437141, 194.9999999999999432, -4.224268460287527560 ) ) ;
#26191=( BOUNDED_CURVE ( )  B_SPLINE_CURVE ( 2, ( #35140, #17917, #34411, #8450, #2935, #14504, #20392, #26060, #20018 ),
 .UNSPECIFIED., .F., .F. ) 
 B_SPLINE_CURVE_WITH_KNOTS ( ( 3, 2, 2, 2, 3 ),
 ( 0.6413043478260869179, 0.6449275362318840354, 0.6521739130434782705, 0.6594202898550725056, 0.6630434782608695121 ),
 .UNSPECIFIED. ) 
 CURVE ( )  GEOMETRIC_REPRESENTATION_ITEM ( )  RATIONAL_B_SPLINE_CURVE ( ( 0.9330127018922194093, 0.9330127018922194093, 1.000000000000000000, 0.8660254037844387076, 1.000000000000000000, 0.8660254037844387076, 1.000000000000000000, 0.9330127018922202975, 0.9330127018922192983 ) ) 
 REPRESENTATION_ITEM ( '' )  );
#26194=ORIENTED_EDGE ( 'NONE', *, *, #8768, .T. ) ;
#26199=AXIS2_PLACEMENT_3D ( 'NONE', #27234, #1821, #16429 ) ;
#26200=CARTESIAN_POINT ( 'NONE',  ( 27.00000000000000355, 196.2875000012290343, -3.306546357697854128E-15 ) ) ;
#26201=CARTESIAN_POINT ( 'NONE',  ( -4.694659320240884604E-14, 197.4124999999999943, 27.00000000000000000 ) ) ;
#26203=CARTESIAN_POINT ( 'NONE',  ( 26.75643035624999655, 244.6843750006145228, -7.049594010296217766E-16 ) ) ;
#26209=CARTESIAN_POINT ( 'NONE',  ( 26.99999999999999645, 247.5437500012290570, 3.464101615137751278 ) ) ;
#26221=CARTESIAN_POINT ( 'NONE',  ( 15.24356964374999990, 247.0468750006145058, 0.000000000000000000 ) ) ;
#26224=CARTESIAN_POINT ( 'NONE',  ( 16.85147890419441197, 211.5556954109263756, -5.808099892140870857 ) ) ;
#26231=DIRECTION ( 'NONE',  ( 0.000000000000000000, 0.000000000000000000, -1.000000000000000000 ) ) ;
#26247=CARTESIAN_POINT ( 'NONE',  ( 7.234628195640363302, 195.8174038105676402, -26.99999999999996803 ) ) ;
#26249=CARTESIAN_POINT ( 'NONE',  ( -13.62178482187500528, 199.7843750006145456, -23.59362340125807123 ) ) ;
#26252=CARTESIAN_POINT ( 'NONE',  ( 18.12178482187500350, 246.7843750006145456, 4.985214923628407568 ) ) ;
#26253=ORIENTED_EDGE ( 'NONE', *, *, #6109, .F. ) ;
#26255=( BOUNDED_CURVE ( )  B_SPLINE_CURVE ( 2, ( #1405, #36087, #10131, #33254, #16203, #8409, #11244, #31891, #2342 ),
 .UNSPECIFIED., .F., .F. ) 
 B_SPLINE_CURVE_WITH_KNOTS ( ( 3, 2, 2, 2, 3 ),
 ( 0.1458333333333333426, 0.1527777777777777901, 0.1666666666666666574, 0.1805555555555555525, 0.1875000000000000000 ),
 .UNSPECIFIED. ) 
 CURVE ( )  GEOMETRIC_REPRESENTATION_ITEM ( )  RATIONAL_B_SPLINE_CURVE ( ( 0.9330127018922194093, 0.9330127018922194093, 1.000000000000000000, 0.8660254037844387076, 1.000000000000000000, 0.8660254037844387076, 1.000000000000000000, 0.9330127018922194093, 0.9330127018922194093 ) ) 
 REPRESENTATION_ITEM ( '' )  );
#26259=CARTESIAN_POINT ( 'NONE',  ( 23.99999999999999645, 241.7500000000000000, -5.196152422706631135 ) ) ;
#26260=CARTESIAN_POINT ( 'NONE',  ( -27.00000000000000355, 198.6500000000000341, 0.000000000000000000 ) ) ;
#26273=CARTESIAN_POINT ( 'NONE',  ( 15.24356964375000167, 239.9968750006145513, 3.323476615752272600 ) ) ;
#26282=CARTESIAN_POINT ( 'NONE',  ( 21.40987794368840014, 195.0000000000000000, -16.52969473239648224 ) ) ;
#26283=CARTESIAN_POINT ( 'NONE',  ( 5.778771075727756162E-15, 195.9218750006145342, 31.45816453501075927 ) ) ;
#26297=CARTESIAN_POINT ( 'NONE',  ( 1.069080835302379631E-14, 195.2750000012290457, 27.00000000000000000 ) ) ;
#26301=CARTESIAN_POINT ( 'NONE',  ( 13.50000000000001421, 196.1000000000000227, 23.38268590217984055 ) ) ;
#26305=CARTESIAN_POINT ( 'NONE',  ( -13.50000000000000533, 198.1250000000000284, -23.38268590217984411 ) ) ;
#26306=CARTESIAN_POINT ( 'NONE',  ( 15.00000000000000000, 248.1625000000000227, -3.464101615137752166 ) ) ;
#26307=CARTESIAN_POINT ( 'NONE',  ( -27.24356964375000345, 198.8656250006145285, -15.72908226750537786 ) ) ;
#26308=EDGE_CURVE ( 'NONE', #23800, #20737, #36256, .T. ) ;
#26313=CARTESIAN_POINT ( 'NONE',  ( -13.62178482187498396, 196.7281250006145399, 23.59362340125808188 ) ) ;
#26314=CARTESIAN_POINT ( 'NONE',  ( 15.24356964374999990, 241.6093750006145058, -3.323476615752268604 ) ) ;
#26318=CARTESIAN_POINT ( 'NONE',  ( 23.87821517812499650, 247.9093750006145171, -4.985214923628404904 ) ) ;
#26324=CARTESIAN_POINT ( 'NONE',  ( 26.75643035624999655, 242.7718750006145001, -7.049594010296217766E-16 ) ) ;
#26337=CARTESIAN_POINT ( 'NONE',  ( 1.255007937094097924E-14, 199.1000000012290627, -27.00000000000000000 ) ) ;
#26340=CARTESIAN_POINT ( 'NONE',  ( 26.75643035624999655, 243.1843750006144944, 3.323476615752267715 ) ) ;
#26345=ADVANCED_FACE ( 'NONE', ( #34814 ), #31976, .T. ) ;
#26346=CARTESIAN_POINT ( 'NONE',  ( 26.99999999999999645, 241.6750000000000114, -7.347880794884117764E-16 ) ) ;
#26348=DIRECTION ( 'NONE',  ( 0.000000000000000000, 0.000000000000000000, 1.000000000000000000 ) ) ;
#26354=CARTESIAN_POINT ( 'NONE',  ( 15.24356964374999990, 248.3593750006145342, -3.323476615752268604 ) ) ;
#26359=ORIENTED_EDGE ( 'NONE', *, *, #23703, .T. ) ;
#26367=CARTESIAN_POINT ( 'NONE',  ( 26.75643035624999655, 248.5843750006145001, 3.323476615752267271 ) ) ;
#26373=VERTEX_POINT ( 'NONE', #32157 ) ;
#26374=CARTESIAN_POINT ( 'NONE',  ( -28.58815133238078232, 203.6511048533163546, 4.874370134510862762 ) ) ;
#26383=EDGE_CURVE ( 'NONE', #35593, #28768, #7094, .T. ) ;
#26391=CARTESIAN_POINT ( 'NONE',  ( 15.00000000000000000, 240.1562500012290684, 0.000000000000000000 ) ) ;
#26393=CARTESIAN_POINT ( 'NONE',  ( 23.87821517812500005, 245.9593750006145569, 4.985214923628404016 ) ) ;
#26395=CARTESIAN_POINT ( 'NONE',  ( 20.99999999999999645, 240.0718750006145399, 6.646953231504538984 ) ) ;
#26399=CARTESIAN_POINT ( 'NONE',  ( 26.99999999999999645, 247.0937500012290400, 3.464101615137751278 ) ) ;
#26407=ORIENTED_EDGE ( 'NONE', *, *, #29602, .T. ) ;
#26409=CARTESIAN_POINT ( 'NONE',  ( 26.75643035624999655, 245.4718750006145171, -7.049594010296217766E-16 ) ) ;
#26416=( BOUNDED_CURVE ( )  B_SPLINE_CURVE ( 2, ( #29185, #3227, #14800, #32225, #26346, #382, #23517, #35063, #9113 ),
 .UNSPECIFIED., .F., .F. ) 
 B_SPLINE_CURVE_WITH_KNOTS ( ( 3, 2, 2, 2, 3 ),
 ( 0.7934782608695651884, 0.7971014492753623060, 0.8043478260869565410, 0.8115942028985507761, 0.8152173913043478937 ),
 .UNSPECIFIED. ) 
 CURVE ( )  GEOMETRIC_REPRESENTATION_ITEM ( )  RATIONAL_B_SPLINE_CURVE ( ( 0.9330127018922194093, 0.9330127018922194093, 1.000000000000000000, 0.8660254037844387076, 1.000000000000000000, 0.8660254037844387076, 1.000000000000000000, 0.9330127018922182991, 0.9330127018922192983 ) ) 
 REPRESENTATION_ITEM ( '' )  );
#26422=VERTEX_POINT ( 'NONE', #3913 ) ;
#26429=AXIS2_PLACEMENT_3D ( 'NONE', #20611, #37278, #3344 ) ;
#26434=CARTESIAN_POINT ( 'NONE',  ( 5.649999999999987921, 244.5000000000000000, 2.500000000000000000 ) ) ;
#26437=CARTESIAN_POINT ( 'NONE',  ( -1.926257025242585782E-15, 199.2968750006145342, -31.45816453501075927 ) ) ;
#26440=CARTESIAN_POINT ( 'NONE',  ( 23.87821517812499650, 247.4593750006145285, -4.985214923628404904 ) ) ;
#26441=EDGE_LOOP ( 'NONE', ( #28073, #3304, #36013, #9959, #15633, #5583, #17148, #22022, #30992, #18231, #36401, #28636, #21444, #10800, #1140, #35294, #2960, #19896, #13095, #15234, #24692, #4085, #27343, #25602, #20356, #21647, #4735, #4137, #18863, #34741, #6557, #473, #8009, #14795, #15359, #9077, #11026, #18535, #30624, #8111, #33989, #25664, #19486, #25520, #16959, #5686, #33811, #37127 ) ) ;
#26443=CARTESIAN_POINT ( 'NONE',  ( 21.00000000000000000, 243.3624999999999829, 5.999999999999998224 ) ) ;
#26447=CARTESIAN_POINT ( 'NONE',  ( 18.00000000000000355, 241.5249999999999773, 5.196152422706632912 ) ) ;
#26451=ORIENTED_EDGE ( 'NONE', *, *, #23618, .F. ) ;
#26459=CARTESIAN_POINT ( 'NONE',  ( 18.12178482187500350, 241.3843750006145115, 4.985214923628407568 ) ) ;
#26469=CARTESIAN_POINT ( 'NONE',  ( 27.24356964375000345, 196.4843750006145626, -3.336375036156643733E-15 ) ) ;
#26474=DIRECTION ( 'NONE',  ( -0.000000000000000000, -0.000000000000000000, 1.000000000000000000 ) ) ;
#26482=CARTESIAN_POINT ( 'NONE',  ( -1.045839947578415010E-13, 195.7250000012290343, 27.00000000000000355 ) ) ;
#26489=CARTESIAN_POINT ( 'NONE',  ( -7.234628195640354420, 195.7049038117966404, 26.99999999999996803 ) ) ;
#26492=DIRECTION ( 'NONE',  ( 0.000000000000000000, 0.000000000000000000, 1.000000000000000000 ) ) ;
#26493=CARTESIAN_POINT ( 'NONE',  ( 26.99999999999999645, 247.5625000000000000, -3.464101615137755275 ) ) ;
#26494=CARTESIAN_POINT ( 'NONE',  ( 27.24356964374999279, 195.1156250006145285, -15.72908226750539207 ) ) ;
#26500=ORIENTED_EDGE ( 'NONE', *, *, #31169, .T. ) ;
#26501=CARTESIAN_POINT ( 'NONE',  ( -27.24356964374999990, 195.7156250006145513, -15.72908226750537786 ) ) ;
#26505=CARTESIAN_POINT ( 'NONE',  ( 23.87821517812499650, 248.3593750006145342, -4.985214923628404904 ) ) ;
#26512=CARTESIAN_POINT ( 'NONE',  ( 20.99999999999999645, 241.0843750006145285, -6.646953231504538984 ) ) ;
#26522=CARTESIAN_POINT ( 'NONE',  ( 20.99999999999999645, 185.0294372515228645, 5.999999999999999112 ) ) ;
#26529=CARTESIAN_POINT ( 'NONE',  ( 15.24356964375000167, 241.2343750006145058, 3.323476615752272600 ) ) ;
#26534=CARTESIAN_POINT ( 'NONE',  ( -1.926257025242585782E-15, 199.2968750006145342, -31.45816453501076637 ) ) ;
#26535=CARTESIAN_POINT ( 'NONE',  ( -20.80563922340697403, 195.0000000000000284, -17.20829382900668492 ) ) ;
#26543=CARTESIAN_POINT ( 'NONE',  ( 26.75643035624999655, 249.5218750006145001, -7.049594010296217766E-16 ) ) ;
#26547=EDGE_CURVE ( 'NONE', #25530, #2674, #19725, .T. ) ;
#26549=PLANE ( 'NONE',  #15401 ) ;
#26555=CARTESIAN_POINT ( 'NONE',  ( 20.99999999999999645, 248.7343750006145058, -6.646953231504538984 ) ) ;
#26563=CARTESIAN_POINT ( 'NONE',  ( 23.99999999999999645, 241.8062500012290457, -5.196152422706631135 ) ) ;
#26567=CARTESIAN_POINT ( 'NONE',  ( 21.00000000000000000, 249.0437500012290570, -5.999999999999998224 ) ) ;
#26573=CARTESIAN_POINT ( 'NONE',  ( 20.99999999999999289, 242.2374999999999545, -5.999999999999997335 ) ) ;
#26580=CARTESIAN_POINT ( 'NONE',  ( 21.00000000000000000, 242.5468750006145342, -6.646953231504538984 ) ) ;
#26582=CARTESIAN_POINT ( 'NONE',  ( 18.12178482187500350, 240.4843750006145342, 4.985214923628407568 ) ) ;
#26585=CARTESIAN_POINT ( 'NONE',  ( 15.00000000000000000, 246.0062500012290627, 0.000000000000000000 ) ) ;
#26588=CARTESIAN_POINT ( 'NONE',  ( 15.00000000000000000, 246.8500000000000227, 0.000000000000000000 ) ) ;
#26596=CARTESIAN_POINT ( 'NONE',  ( 26.75643035624999655, 247.2343750006145058, 3.323476615752267715 ) ) ;
#26600=CARTESIAN_POINT ( 'NONE',  ( 21.00000000000001776, 209.9999999999999432, -5.999999999999996447 ) ) ;
#26602=SURFACE_STYLE_FILL_AREA ( #4045 ) ;
#26619=CARTESIAN_POINT ( 'NONE',  ( 24.00000000000000000, 247.0562500012290457, 5.196152422706629359 ) ) ;
#26623=CARTESIAN_POINT ( 'NONE',  ( 22.60769515458672885, 241.3736538117966859, -5.999999999999998224 ) ) ;
#26626=CARTESIAN_POINT ( 'NONE',  ( 18.12178482187499640, 245.7343750006145342, -4.985214923628404904 ) ) ;
#26630=DIRECTION ( 'NONE',  ( 0.000000000000000000, -1.000000000000000000, 0.000000000000000000 ) ) ;
#26634=CARTESIAN_POINT ( 'NONE',  ( 24.00000000000000000, 240.2500000000000000, 5.196152422706629359 ) ) ;
#26641=FACE_OUTER_BOUND ( 'NONE', #30982, .T. ) ;
#26648=CARTESIAN_POINT ( 'NONE',  ( 26.75643035624999655, 240.5968750006145456, 3.323476615752267715 ) ) ;
#26658=CARTESIAN_POINT ( 'NONE',  ( -13.62178482187500528, 198.8281250006145342, -23.59362340125807123 ) ) ;
#26661=ORIENTED_EDGE ( 'NONE', *, *, #5997, .T. ) ;
#26663=CARTESIAN_POINT ( 'NONE',  ( 24.00000000000000000, 245.2562500012290627, 5.196152422706629359 ) ) ;
#26664=CARTESIAN_POINT ( 'NONE',  ( -3.253724281355068545E-15, 198.6500000012290172, -27.00000000000000355 ) ) ;
#26674=CYLINDRICAL_SURFACE ( 'NONE', #21049, 5.999999999999999112 ) ;
#26675=FACE_OUTER_BOUND ( 'NONE', #5281, .T. ) ;
#26683=CARTESIAN_POINT ( 'NONE',  ( 21.00000000000000000, 248.0875000000000057, -6.928203230275506996 ) ) ;
#26684=CARTESIAN_POINT ( 'NONE',  ( -13.62178482187498396, 195.8281250006145342, 23.59362340125808188 ) ) ;
#26689=CARTESIAN_POINT ( 'NONE',  ( 13.62178482187499640, 195.6031250006145115, -23.59362340125807123 ) ) ;
#26690=CARTESIAN_POINT ( 'NONE',  ( 15.24356964374999990, 240.2593750006145115, -3.323476615752268604 ) ) ;
#26693=CARTESIAN_POINT ( 'NONE',  ( 15.24356964374999990, 248.0218750006145285, -3.323476615752268604 ) ) ;
#26699=CARTESIAN_POINT ( 'NONE',  ( 18.12178482187499640, 242.9218750006145058, -4.985214923628404904 ) ) ;
#26710=CARTESIAN_POINT ( 'NONE',  ( 23.99999999999999645, 248.5000000000000000, -5.196152422706631135 ) ) ;
#26717=CARTESIAN_POINT ( 'NONE',  ( 23.87821517812500005, 241.7968750006145342, 4.985214923628404016 ) ) ;
#26728=ORIENTED_EDGE ( 'NONE', *, *, #13511, .F. ) ;
#26730=CARTESIAN_POINT ( 'NONE',  ( 15.24356964374999990, 247.0468750006145058, 0.000000000000000000 ) ) ;
#26737=ORIENTED_EDGE ( 'NONE', *, *, #7630, .T. ) ;
#26744=CARTESIAN_POINT ( 'NONE',  ( 23.87821517812499650, 248.2468750006145228, -4.985214923628404904 ) ) ;
#26747=CARTESIAN_POINT ( 'NONE',  ( 27.00000000000000355, 196.6250000000000284, -3.306546357697854128E-15 ) ) ;
#26758=CARTESIAN_POINT ( 'NONE',  ( 15.00000000000000000, 246.4187500012290286, -3.464101615137752610 ) ) ;
#26762=DIRECTION ( 'NONE',  ( -4.130293990420971855E-17, 1.000000000000000000, 0.000000000000000000 ) ) ;
#26767=CARTESIAN_POINT ( 'NONE',  ( -14.50000000000000000, 215.7563705986615901, -5.555555555555558023 ) ) ;
#26773=CARTESIAN_POINT ( 'NONE',  ( 15.24356964375000167, 240.4468750006145399, 3.323476615752272600 ) ) ;
#26774=ORIENTED_EDGE ( 'NONE', *, *, #37465, .T. ) ;
#26775=CARTESIAN_POINT ( 'NONE',  ( 18.00000000000000000, 242.7812500012290400, -5.196152422706630247 ) ) ;
#26779=CARTESIAN_POINT ( 'NONE',  ( 15.00000000000000178, 246.8874999999999886, 3.464101615137757051 ) ) ;
#26787=CARTESIAN_POINT ( 'NONE',  ( 15.24356964375000167, 245.2843750006144887, 3.323476615752272600 ) ) ;
#26803=CARTESIAN_POINT ( 'NONE',  ( 26.99999999999999645, 240.7374999999999545, 3.464101615137751278 ) ) ;
#26806=DIRECTION ( 'NONE',  ( -0.000000000000000000, 1.000000000000000000, -0.000000000000000000 ) ) ;
#26810=CARTESIAN_POINT ( 'NONE',  ( 22.60769515458674306, 247.0388461906614168, 5.999999999999992895 ) ) ;
#26812=DIRECTION ( 'NONE',  ( -0.000000000000000000, -1.000000000000000000, -0.000000000000000000 ) ) ;
#26814=CARTESIAN_POINT ( 'NONE',  ( 23.99999999999999645, 241.3562500012290286, -5.196152422706631135 ) ) ;
#26816=DIRECTION ( 'NONE',  ( 0.000000000000000000, 0.000000000000000000, 1.000000000000000000 ) ) ;
#26818=CARTESIAN_POINT ( 'NONE',  ( 23.87821517812500005, 247.3093750006145228, 4.985214923628404016 ) ) ;
#26823=DIRECTION ( 'NONE',  ( -0.000000000000000000, 1.000000000000000000, -0.000000000000000000 ) ) ;
#26831=ORIENTED_EDGE ( 'NONE', *, *, #9631, .T. ) ;
#26832=LINE ( 'NONE', #36107, #24294 ) ;
#26834=CARTESIAN_POINT ( 'NONE',  ( 24.00000000000000000, 246.5499999999999829, 5.196152422706629359 ) ) ;
#26835=CARTESIAN_POINT ( 'NONE',  ( 27.00000000000000355, 195.2750000000000057, -3.306546357697854128E-15 ) ) ;
#26842=CARTESIAN_POINT ( 'NONE',  ( 18.00000000000000000, 245.4250000000000114, -5.196152422706630247 ) ) ;
#26850=CARTESIAN_POINT ( 'NONE',  ( -13.62178482187498396, 198.9781250006145399, 23.59362340125808188 ) ) ;
#26855=CARTESIAN_POINT ( 'NONE',  ( 15.00000000000000178, 244.6937500012290627, 3.464101615137757051 ) ) ;
#26856=CARTESIAN_POINT ( 'NONE',  ( 20.99999999999998579, 247.2437500012290457, -5.999999999999997335 ) ) ;
#26866=DIRECTION ( 'NONE',  ( -0.000000000000000000, -1.000000000000000000, -0.000000000000000000 ) ) ;
#26868=VERTEX_POINT ( 'NONE', #17117 ) ;
#26869=CARTESIAN_POINT ( 'NONE',  ( 24.00000000000000000, 244.8062500012290457, 5.196152422706629359 ) ) ;
#26871=CYLINDRICAL_SURFACE ( 'NONE', #21207, 5.999999999999999112 ) ;
#26875=CARTESIAN_POINT ( 'NONE',  ( 15.00000000000000000, 249.5499999999999829, 0.000000000000000000 ) ) ;
#26876=CARTESIAN_POINT ( 'NONE',  ( -27.24356964375000345, 195.7156250006145513, -15.72908226750537786 ) ) ;
#26880=EDGE_LOOP ( 'NONE', ( #27718, #2819, #7683 ) ) ;
#26881=ORIENTED_EDGE ( 'NONE', *, *, #7534, .F. ) ;
#26882=CARTESIAN_POINT ( 'NONE',  ( -27.24356964375000345, 196.2031250006145342, 0.000000000000000000 ) ) ;
#26883=DIRECTION ( 'NONE',  ( -0.000000000000000000, 1.000000000000000000, -0.000000000000000000 ) ) ;
#26886=CARTESIAN_POINT ( 'NONE',  ( 21.00000000000000000, 248.3968750006145285, -6.646953231504538984 ) ) ;
#26888=AXIS2_PLACEMENT_3D ( 'NONE', #28864, #26025, #5372 ) ;
#26895=CARTESIAN_POINT ( 'NONE',  ( 15.24356964374999990, 240.7468750006144944, 0.000000000000000000 ) ) ;
#26909=FACE_OUTER_BOUND ( 'NONE', #31085, .T. ) ;
#26912=CARTESIAN_POINT ( 'NONE',  ( 23.87821517812499650, 243.2968750006145058, -4.985214923628404904 ) ) ;
#26923=CARTESIAN_POINT ( 'NONE',  ( 26.75643035624999655, 246.8218750006145115, -7.049594010296217766E-16 ) ) ;
#26931=ORIENTED_EDGE ( 'NONE', *, *, #4147, .T. ) ;
#26936=CARTESIAN_POINT ( 'NONE',  ( 18.12178482187499640, 245.6218750006145228, -4.985214923628404904 ) ) ;
#26937=CARTESIAN_POINT ( 'NONE',  ( 7.234628195640269155, 196.5325961894323257, 27.00000000000003197 ) ) ;
#26942=EDGE_LOOP ( 'NONE', ( #7401, #1000, #14991 ) ) ;
#26951=CARTESIAN_POINT ( 'NONE',  ( 13.50000000000001421, 197.5625000012290400, 23.38268590217984055 ) ) ;
#26958=CARTESIAN_POINT ( 'NONE',  ( 0.000000000000000000, 0.000000000000000000, -2.500000000000000000 ) ) ;
#26960=DIRECTION ( 'NONE',  ( -0.000000000000000000, -1.000000000000000000, -0.000000000000000000 ) ) ;
#26965=CARTESIAN_POINT ( 'NONE',  ( 23.99999999999999645, 244.5062500012290627, -5.196152422706631135 ) ) ;
#26971=EDGE_CURVE ( 'NONE', #8056, #4638, #16930, .T. ) ;
#26975=ORIENTED_EDGE ( 'NONE', *, *, #36583, .F. ) ;
#26977=CARTESIAN_POINT ( 'NONE',  ( 18.12178482187499640, 245.1718750006145058, -4.985214923628404904 ) ) ;
#26979=( BOUNDED_CURVE ( )  B_SPLINE_CURVE ( 2, ( #6375, #17577, #20987, #11870, #9036, #23818, #31966, #31775, #677 ),
 .UNSPECIFIED., .F., .F. ) 
 B_SPLINE_CURVE_WITH_KNOTS ( ( 3, 2, 2, 2, 3 ),
 ( 0.05434782608695652023, 0.05797101449275362389, 0.06521739130434782428, 0.07246376811594203160, 0.07608695652173913526 ),
 .UNSPECIFIED. ) 
 CURVE ( )  GEOMETRIC_REPRESENTATION_ITEM ( )  RATIONAL_B_SPLINE_CURVE ( ( 0.9330127018922191873, 0.9330127018922191873, 1.000000000000000000, 0.8660254037844387076, 1.000000000000000000, 0.8660254037844387076, 1.000000000000000000, 0.9330127018922191873, 0.9330127018922192983 ) ) 
 REPRESENTATION_ITEM ( '' )  );
#26994=VECTOR ( 'NONE', #26762, 1000.000000000000000 ) ;
#26997=DIRECTION ( 'NONE',  ( -0.000000000000000000, 1.000000000000000000, -0.000000000000000000 ) ) ;
#27003=DIRECTION ( 'NONE',  ( 0.000000000000000000, 0.000000000000000000, -1.000000000000000000 ) ) ;
#27007=CARTESIAN_POINT ( 'NONE',  ( 21.00000000000000000, 249.5218750006145285, 6.646953231504538984 ) ) ;
#27009=CARTESIAN_POINT ( 'NONE',  ( 20.99999999999999645, 245.4718750006145456, 6.646953231504538984 ) ) ;
#27013=VECTOR ( 'NONE', #34908, 1000.000000000000000 ) ;
#27014=EDGE_CURVE ( 'NONE', #28321, #27758, #31539, .T. ) ;
#27023=CARTESIAN_POINT ( 'NONE',  ( -7.234628195640354420, 196.0424038105676630, 26.99999999999996803 ) ) ;
#27026=CARTESIAN_POINT ( 'NONE',  ( 19.39230484541326405, 248.2924038105676630, 5.999999999999995559 ) ) ;
#27040=CARTESIAN_POINT ( 'NONE',  ( 26.99999999999999645, 247.0749999999999886, -7.347880794884117764E-16 ) ) ;
#27041=CARTESIAN_POINT ( 'NONE',  ( -1.926257025242585782E-15, 197.8906250006145342, -31.45816453501075927 ) ) ;
#27060=CARTESIAN_POINT ( 'NONE',  ( 23.99999999999999645, 247.6562500012290400, -5.196152422706631135 ) ) ;
#27070=CARTESIAN_POINT ( 'NONE',  ( 18.00000000000000000, 246.3249999999999886, -5.196152422706630247 ) ) ;
#27071=CARTESIAN_POINT ( 'NONE',  ( -27.24356964374999279, 196.6906250006145456, 15.72908226750539384 ) ) ;
#27076=CARTESIAN_POINT ( 'NONE',  ( -27.24356964375000345, 195.7531250006145456, 0.000000000000000000 ) ) ;
#27077=CARTESIAN_POINT ( 'NONE',  ( 18.12178482187500350, 240.3718750006145228, 4.985214923628407568 ) ) ;
#27081=CARTESIAN_POINT ( 'NONE',  ( 15.24356964374999990, 245.3593750006145342, 0.000000000000000000 ) ) ;
#27085=EDGE_CURVE ( 'NONE', #24290, #17896, #37133, .T. ) ;
#27087=EDGE_CURVE ( 'NONE', #36527, #25890, #25996, .T. ) ;
#27094=EDGE_CURVE ( 'NONE', #2407, #31898, #36402, .T. ) ;
#27102=CARTESIAN_POINT ( 'NONE',  ( 18.00000000000000355, 248.3312500012290513, 5.196152422706632912 ) ) ;
#27105=CARTESIAN_POINT ( 'NONE',  ( 21.00000000000000000, 249.0718750006145399, 6.646953231504538984 ) ) ;
#27106=ORIENTED_EDGE ( 'NONE', *, *, #4027, .F. ) ;
#27109=CARTESIAN_POINT ( 'NONE',  ( -27.24356964374999279, 199.4468750006145399, 15.72908226750539384 ) ) ;
#27110=CARTESIAN_POINT ( 'NONE',  ( 19.95811783012822005, 240.0005236131589754, -5.908847734042844912 ) ) ;
#27111=DIRECTION ( 'NONE',  ( -0.000000000000000000, 1.000000000000000000, -0.000000000000000000 ) ) ;
#27116=EDGE_LOOP ( 'NONE', ( #25853, #15841, #15212, #63 ) ) ;
#27117=ORIENTED_EDGE ( 'NONE', *, *, #17824, .F. ) ;
#27118=CARTESIAN_POINT ( 'NONE',  ( 26.75643035624999655, 245.9218750006145342, -7.049594010296217766E-16 ) ) ;
#27130=CARTESIAN_POINT ( 'NONE',  ( 15.24356964374999990, 246.1093750006145342, -3.323476615752268604 ) ) ;
#27131=CARTESIAN_POINT ( 'NONE',  ( 20.99999999999999289, 240.4374999999999716, -5.999999999999997335 ) ) ;
#27135=ORIENTED_EDGE ( 'NONE', *, *, #1487, .T. ) ;
#27143=EDGE_CURVE ( 'NONE', #21628, #9483, #22155, .T. ) ;
#27146=ORIENTED_EDGE ( 'NONE', *, *, #9642, .T. ) ;
#27152=CARTESIAN_POINT ( 'NONE',  ( 7.234628195640309123, 195.9299038117966916, -27.00000000000000711 ) ) ;
#27153=CARTESIAN_POINT ( 'NONE',  ( -13.62178482187498396, 199.4843750006145626, 23.59362340125808188 ) ) ;
#27159=CARTESIAN_POINT ( 'NONE',  ( 26.99999999999999645, 244.4312500012290457, -7.347880794884117764E-16 ) ) ;
#27162=CARTESIAN_POINT ( 'NONE',  ( -27.24356964374999990, 199.7656250006145342, -15.72908226750537786 ) ) ;
#27167=CARTESIAN_POINT ( 'NONE',  ( 18.12178482187500350, 244.8718750006145228, 4.985214923628407568 ) ) ;
#27180=CARTESIAN_POINT ( 'NONE',  ( 1.069080835302379631E-14, 199.6625000000000227, 27.00000000000000000 ) ) ;
#27184=CARTESIAN_POINT ( 'NONE',  ( 20.99999999999999645, 185.0294372515228645, 5.999999999999999112 ) ) ;
#27189=LINE ( 'NONE', #6922, #116 ) ;
#27193=CARTESIAN_POINT ( 'NONE',  ( 18.12178482187499640, 249.3343750006145285, -4.985214923628404904 ) ) ;
#27195=CARTESIAN_POINT ( 'NONE',  ( 18.12178482187499640, 244.3843750006145115, -4.985214923628404904 ) ) ;
#27205=ORIENTED_EDGE ( 'NONE', *, *, #23044, .F. ) ;
#27207=ORIENTED_EDGE ( 'NONE', *, *, #34894, .T. ) ;
#27218=CARTESIAN_POINT ( 'NONE',  ( 7.405590309535792670, 215.0979036339245170, 3.170162721592201471 ) ) ;
#27227=CARTESIAN_POINT ( 'NONE',  ( 22.60769515458672174, 246.9825961894323427, 6.000000000000004441 ) ) ;
#27228=CARTESIAN_POINT ( 'NONE',  ( 27.24356964375000345, 199.1281250006145171, -3.336375036156643733E-15 ) ) ;
#27234=CARTESIAN_POINT ( 'NONE',  ( 2.999999999999997335, 244.5000000000000000, -2.499999999999999556 ) ) ;
#27244=CARTESIAN_POINT ( 'NONE',  ( -3.253724281355068545E-15, 198.9874999999999829, -27.00000000000000355 ) ) ;
#27249=ORIENTED_EDGE ( 'NONE', *, *, #2981, .F. ) ;
#27256=CARTESIAN_POINT ( 'NONE',  ( 26.99999999999999645, 245.7249999999999943, -7.347880794884117764E-16 ) ) ;
#27257=CARTESIAN_POINT ( 'NONE',  ( 13.62178482187501416, 197.2531250006145456, 23.59362340125806767 ) ) ;
#27260=ORIENTED_EDGE ( 'NONE', *, *, #18977, .T. ) ;
#27261=ORIENTED_EDGE ( 'NONE', *, *, #15030, .T. ) ;
#27262=CARTESIAN_POINT ( 'NONE',  ( 5.727106289114498080E-15, 199.3250000012290570, 31.17691453623979214 ) ) ;
#27263=CARTESIAN_POINT ( 'NONE',  ( 15.24356964374999990, 240.7093750006145285, -3.323476615752268604 ) ) ;
#27266=CARTESIAN_POINT ( 'NONE',  ( 26.75643035624999655, 244.2343750006145342, -7.049594010296217766E-16 ) ) ;
#27268=( BOUNDED_CURVE ( )  B_SPLINE_CURVE ( 2, ( #13401, #7715, #13219, #33675, #36138, #18919, #24770, #30656, #5046 ),
 .UNSPECIFIED., .F., .F. ) 
 B_SPLINE_CURVE_WITH_KNOTS ( ( 3, 2, 2, 2, 3 ),
 ( 0.3369565217391304324, 0.3405797101449275499, 0.3478260869565217295, 0.3550724637681159646, 0.3586956521739130266 ),
 .UNSPECIFIED. ) 
 CURVE ( )  GEOMETRIC_REPRESENTATION_ITEM ( )  RATIONAL_B_SPLINE_CURVE ( ( 0.9330127018922194093, 0.9330127018922194093, 1.000000000000000000, 0.8660254037844387076, 1.000000000000000000, 0.8660254037844387076, 1.000000000000000000, 0.9330127018922198534, 0.9330127018922191873 ) ) 
 REPRESENTATION_ITEM ( '' )  );
#27272=CARTESIAN_POINT ( 'NONE',  ( 27.00000000000000355, 197.9750000000000227, -3.306546357697854128E-15 ) ) ;
#27286=CARTESIAN_POINT ( 'NONE',  ( 26.75643035624999655, 249.6343750006145399, -7.049594010296217766E-16 ) ) ;
#27295=CARTESIAN_POINT ( 'NONE',  ( 21.00000000000000000, 243.8968750006145001, -6.646953231504538984 ) ) ;
#27299=ORIENTED_EDGE ( 'NONE', *, *, #34611, .F. ) ;
#27300=VERTEX_POINT ( 'NONE', #784 ) ;
#27301=CARTESIAN_POINT ( 'NONE',  ( 18.12178482187499640, 246.9718750006145171, -4.985214923628404904 ) ) ;
#27303=EDGE_CURVE ( 'NONE', #15380, #1047, #12353, .T. ) ;
#27310=ORIENTED_EDGE ( 'NONE', *, *, #24057, .T. ) ;
#27315=AXIS2_PLACEMENT_3D ( 'NONE', #33274, #30437, #4456 ) ;
#27318=CARTESIAN_POINT ( 'NONE',  ( 23.87821517812500005, 247.6468750006145285, 4.985214923628404016 ) ) ;
#27321=CARTESIAN_POINT ( 'NONE',  ( 15.00000000000000000, 245.9124999999999943, -3.464101615137752610 ) ) ;
#27329=CARTESIAN_POINT ( 'NONE',  ( 18.00000000000000000, 246.3812500012290343, -5.196152422706630247 ) ) ;
#27338=DIRECTION ( 'NONE',  ( -0.000000000000000000, 1.000000000000000000, -0.000000000000000000 ) ) ;
#27339=CARTESIAN_POINT ( 'NONE',  ( 27.24356964374999635, 199.6718750006145058, -15.72908226750539029 ) ) ;
#27343=ORIENTED_EDGE ( 'NONE', *, *, #30568, .F. ) ;
#27345=CARTESIAN_POINT ( 'NONE',  ( 15.00000000000000000, 244.2062500012290513, 0.000000000000000000 ) ) ;
#27351=ORIENTED_EDGE ( 'NONE', *, *, #34661, .F. ) ;
#27353=CARTESIAN_POINT ( 'NONE',  ( 21.00000000000000000, 243.5593750006145228, 6.646953231504538984 ) ) ;
#27370=CARTESIAN_POINT ( 'NONE',  ( -27.87471972953270338, 210.0000000000000284, -8.000000000000000000 ) ) ;
#27379=CARTESIAN_POINT ( 'NONE',  ( 15.24356964375000167, 248.9968750006145513, 3.323476615752272600 ) ) ;
#27381=CARTESIAN_POINT ( 'NONE',  ( 26.75643035624999655, 245.1343750006145115, -7.049594010296217766E-16 ) ) ;
#27387=DIRECTION ( 'NONE',  ( 0.000000000000000000, 0.000000000000000000, -1.000000000000000000 ) ) ;
#27403=CARTESIAN_POINT ( 'NONE',  ( -5.732297079746171420, 222.9518338469886203, 2.500000000000000000 ) ) ;
#27410=CARTESIAN_POINT ( 'NONE',  ( 5.778771075727756162E-15, 199.0156250006145342, 31.45816453501075927 ) ) ;
#27422=( BOUNDED_CURVE ( )  B_SPLINE_CURVE ( 2, ( #16895, #2475, #17265, #9100, #28805, #25597, #3030, #8542, #14232 ),
 .UNSPECIFIED., .F., .T. ) 
 B_SPLINE_CURVE_WITH_KNOTS ( ( 3, 2, 2, 2, 3 ),
 ( 0.4891304347826087029, 0.4927536231884058204, 0.5000000000000000000, 0.5072463768115942351, 0.5108695652173913526 ),
 .UNSPECIFIED. ) 
 CURVE ( )  GEOMETRIC_REPRESENTATION_ITEM ( )  RATIONAL_B_SPLINE_CURVE ( ( 0.9330127018922194093, 0.9330127018922194093, 1.000000000000000000, 0.8660254037844387076, 1.000000000000000000, 0.8660254037844387076, 1.000000000000000000, 0.9330127018922182991, 0.9330127018922192983 ) ) 
 REPRESENTATION_ITEM ( '' )  );
#27424=CARTESIAN_POINT ( 'NONE',  ( 19.39230484541326760, 240.6986538117967314, 5.999999999999999112 ) ) ;
#27428=CARTESIAN_POINT ( 'NONE',  ( -13.50000000000000533, 199.4750000000000227, -23.38268590217984411 ) ) ;
#27429=DIRECTION ( 'NONE',  ( 0.000000000000000000, 0.000000000000000000, 1.000000000000000000 ) ) ;
#27439=CARTESIAN_POINT ( 'NONE',  ( 18.00000000000000355, 246.0250000000000057, 5.196152422706632912 ) ) ;
#27444=VERTEX_POINT ( 'NONE', #18998 ) ;
#27445=ORIENTED_EDGE ( 'NONE', *, *, #28150, .T. ) ;
#27446=CARTESIAN_POINT ( 'NONE',  ( 27.00000000000000355, 199.4375000012290400, -3.306546357697854128E-15 ) ) ;
#27452=CARTESIAN_POINT ( 'NONE',  ( 18.12178482187499640, 246.1843750006145228, -4.985214923628404904 ) ) ;
#27456=FACE_BOUND ( 'NONE', #20968, .T. ) ;
#27470=CARTESIAN_POINT ( 'NONE',  ( 20.99999999999999645, 185.0294372515228645, 5.999999999999999112 ) ) ;
#27476=CARTESIAN_POINT ( 'NONE',  ( 18.12178482187500350, 240.3718750006145228, 4.985214923628407568 ) ) ;
#27480=CARTESIAN_POINT ( 'NONE',  ( 13.62178482187499640, 198.8093750006145513, -23.59362340125807123 ) ) ;
#27484=CARTESIAN_POINT ( 'NONE',  ( 26.75643035624999655, 242.9218750006145626, -3.323476615752271712 ) ) ;
#27493=CARTESIAN_POINT ( 'NONE',  ( 15.24356964374999990, 247.9468750006145115, 0.000000000000000000 ) ) ;
#27496=VECTOR ( 'NONE', #1810, 1000.000000000000000 ) ;
#27508=CARTESIAN_POINT ( 'NONE',  ( 20.99999999999999645, 246.4843750006145058, -6.646953231504538984 ) ) ;
#27512=CARTESIAN_POINT ( 'NONE',  ( 19.39230484541326049, 245.8575961894323427, -5.999999999999997335 ) ) ;
#27529=CARTESIAN_POINT ( 'NONE',  ( 13.62178482187501416, 197.3093750006145513, 23.59362340125806767 ) ) ;
#27530=CARTESIAN_POINT ( 'NONE',  ( 15.00000000000000000, 250.0000000000000000, 0.000000000000000000 ) ) ;
#27534=CARTESIAN_POINT ( 'NONE',  ( 15.00000000000000000, 244.6562500012290400, 0.000000000000000000 ) ) ;
#27537=CARTESIAN_POINT ( 'NONE',  ( 20.99999999999995381, 242.9124999999999943, 5.999999999999998224 ) ) ;
#27540=ORIENTED_EDGE ( 'NONE', *, *, #30260, .T. ) ;
#27542=CARTESIAN_POINT ( 'NONE',  ( 18.12178482187499640, 243.8218750006145399, -4.985214923628404904 ) ) ;
#27562=ORIENTED_EDGE ( 'NONE', *, *, #5692, .F. ) ;
#27572=CARTESIAN_POINT ( 'NONE',  ( 15.24356964375000167, 244.4968750006145513, 3.323476615752272600 ) ) ;
#27575=LINE ( 'NONE', #32558, #13239 ) ;
#27579=CARTESIAN_POINT ( 'NONE',  ( 19.95811783012620566, 240.0005235271234483, -5.908847734042487865 ) ) ;
#27593=CARTESIAN_POINT ( 'NONE',  ( 17.99309595496610470, 218.0184107867572720, 5.206989594055762893 ) ) ;
#27602=CARTESIAN_POINT ( 'NONE',  ( -1.926257025242585782E-15, 196.5406250006145399, -31.45816453501075927 ) ) ;
#27618=CARTESIAN_POINT ( 'NONE',  ( 20.99999999999999645, 250.0000000000000000, 0.000000000000000000 ) ) ;
#27619=EDGE_CURVE ( 'NONE', #3985, #253, #37148, .T. ) ;
#27622=CARTESIAN_POINT ( 'NONE',  ( 13.50000000000001421, 199.2500000000000000, 23.38268590217984055 ) ) ;
#27625=DIRECTION ( 'NONE',  ( 0.000000000000000000, 0.000000000000000000, -1.000000000000000000 ) ) ;
#27630=CARTESIAN_POINT ( 'NONE',  ( 18.00000000000000355, 246.4749999999999943, 5.196152422706632912 ) ) ;
#27636=EDGE_LOOP ( 'NONE', ( #26728, #28539, #19444, #11230 ) ) ;
#27637=CARTESIAN_POINT ( 'NONE',  ( -13.49999999999998401, 198.8375000012290457, 23.38268590217985476 ) ) ;
#27642=CARTESIAN_POINT ( 'NONE',  ( 26.75643035624999655, 245.9968750006145513, 3.323476615752267715 ) ) ;
#27643=ADVANCED_FACE ( 'NONE', ( #22764 ), #19929, .F. ) ;
#27650=CARTESIAN_POINT ( 'NONE',  ( 15.24356964374999990, 239.8093750006145228, -3.323476615752268604 ) ) ;
#27652=( BOUNDED_CURVE ( )  B_SPLINE_CURVE ( 2, ( #32554, #3745, #23854, #12088, #6784, #15511, #15319, #3936, #24040 ),
 .UNSPECIFIED., .F., .F. ) 
 B_SPLINE_CURVE_WITH_KNOTS ( ( 3, 2, 2, 2, 3 ),
 ( 0.2291666666666666574, 0.2361111111111111049, 0.2500000000000000000, 0.2638888888888888951, 0.2708333333333333703 ),
 .UNSPECIFIED. ) 
 CURVE ( )  GEOMETRIC_REPRESENTATION_ITEM ( )  RATIONAL_B_SPLINE_CURVE ( ( 0.9330127018922194093, 0.9330127018922194093, 1.000000000000000000, 0.8660254037844387076, 1.000000000000000000, 0.8660254037844387076, 1.000000000000000000, 0.9330127018922190762, 0.9330127018922194093 ) ) 
 REPRESENTATION_ITEM ( '' )  );
#27655=DIRECTION ( 'NONE',  ( -0.000000000000000000, 1.000000000000000000, -0.000000000000000000 ) ) ;
#27665=CARTESIAN_POINT ( 'NONE',  ( 23.87821517812499650, 249.7093750006145285, -4.985214923628404904 ) ) ;
#27669=CARTESIAN_POINT ( 'NONE',  ( -27.24356964375000345, 196.7093750006145569, 0.000000000000000000 ) ) ;
#27671=CARTESIAN_POINT ( 'NONE',  ( 26.75643035624999655, 243.3343750006145285, -7.049594010296217766E-16 ) ) ;
#27678=CARTESIAN_POINT ( 'NONE',  ( 15.24356964374999990, 243.4468750006145115, 0.000000000000000000 ) ) ;
#27691=CARTESIAN_POINT ( 'NONE',  ( 18.12178482187499640, 247.8718750006145228, -4.985214923628404904 ) ) ;
#27694=CARTESIAN_POINT ( 'NONE',  ( 26.99999999999999645, 240.2874999999999943, 3.464101615137751278 ) ) ;
#27713=CARTESIAN_POINT ( 'NONE',  ( -13.62178482187500528, 198.8843750006145399, -23.59362340125807123 ) ) ;
#27718=ORIENTED_EDGE ( 'NONE', *, *, #33864, .T. ) ;
#27719=CARTESIAN_POINT ( 'NONE',  ( 15.00000000000000178, 241.5437500012290570, 3.464101615137757051 ) ) ;
#27720=CIRCLE ( 'NONE', #2012, 28.99999999999999645 ) ;
#27723=CARTESIAN_POINT ( 'NONE',  ( -13.62178482187500528, 199.7281250006145399, -23.59362340125807123 ) ) ;
#27727=CIRCLE ( 'NONE', #11378, 28.99999999999999645 ) ;
#27733=CARTESIAN_POINT ( 'NONE',  ( -27.00000000000000355, 196.4000000000000057, 0.000000000000000000 ) ) ;
#27753=DIRECTION ( 'NONE',  ( 0.000000000000000000, 0.000000000000000000, 1.000000000000000000 ) ) ;
#27755=CARTESIAN_POINT ( 'NONE',  ( 26.75643035624999655, 248.3218750006145399, -3.323476615752271712 ) ) ;
#27757=CARTESIAN_POINT ( 'NONE',  ( 26.75643035624999655, 243.3343750006145285, -7.049594010296217766E-16 ) ) ;
#27758=VERTEX_POINT ( 'NONE', #31651 ) ;
#27765=CARTESIAN_POINT ( 'NONE',  ( 26.99999999999999645, 240.7937500012290570, 3.464101615137751278 ) ) ;
#27771=ORIENTED_EDGE ( 'NONE', *, *, #17291, .F. ) ;
#27773=CARTESIAN_POINT ( 'NONE',  ( 21.00000000000000000, 242.0687500012289775, 5.999999999999998224 ) ) ;
#27779=EDGE_CURVE ( 'NONE', #23066, #20369, #10954, .T. ) ;
#27781=CARTESIAN_POINT ( 'NONE',  ( 14.99999999999999822, 225.9999999999999716, -0.1963495407219250366 ) ) ;
#27784=CARTESIAN_POINT ( 'NONE',  ( 20.99999999999999645, 185.0294372515228645, -5.999999999999999112 ) ) ;
#27790=CARTESIAN_POINT ( 'NONE',  ( 27.24356964375000700, 197.2906250006145399, 15.72908226750537075 ) ) ;
#27806=CARTESIAN_POINT ( 'NONE',  ( 2.999999999999997335, 244.5000000000000000, -2.499999999999999556 ) ) ;
#27808=CARTESIAN_POINT ( 'NONE',  ( -13.49999999999998401, 199.6250000000000284, 23.38268590217985476 ) ) ;
#27817=CARTESIAN_POINT ( 'NONE',  ( 26.99999999999999645, 246.1750000000000114, -7.347880794884117764E-16 ) ) ;
#27821=ORIENTED_EDGE ( 'NONE', *, *, #33561, .T. ) ;
#27822=ORIENTED_EDGE ( 'NONE', *, *, #36115, .F. ) ;
#27823=CARTESIAN_POINT ( 'NONE',  ( 27.00000000000001066, 199.4000000012290172, 15.58845726811988897 ) ) ;
#27826=CARTESIAN_POINT ( 'NONE',  ( 26.75643035624999655, 246.0718750006145115, -3.323476615752271712 ) ) ;
#27832=CARTESIAN_POINT ( 'NONE',  ( 27.24356964375000700, 198.2468750006145513, 15.72908226750537075 ) ) ;
#27836=CARTESIAN_POINT ( 'NONE',  ( 19.39230484541327471, 247.3924038105677141, 6.000000000000002665 ) ) ;
#27849=CARTESIAN_POINT ( 'NONE',  ( 13.62178482187501416, 198.2093750006145285, 23.59362340125806767 ) ) ;
#27853=CARTESIAN_POINT ( 'NONE',  ( 21.00000000000000000, 243.6718750006145058, 6.646953231504538984 ) ) ;
#27860=CARTESIAN_POINT ( 'NONE',  ( 23.87821517812500005, 243.5968750006145171, 4.985214923628404016 ) ) ;
#27867=ORIENTED_EDGE ( 'NONE', *, *, #16847, .T. ) ;
#27874=CARTESIAN_POINT ( 'NONE',  ( 23.87821517812500005, 244.9468750006145115, 4.985214923628404016 ) ) ;
#27875=CARTESIAN_POINT ( 'NONE',  ( -27.00000000000000355, 197.4125000012290343, 0.000000000000000000 ) ) ;
#27882=CARTESIAN_POINT ( 'NONE',  ( 20.99999999999999289, 244.4874999999999829, -5.999999999999997335 ) ) ;
#27886=EDGE_CURVE ( 'NONE', #18467, #2746, #31834, .T. ) ;
#27888=VERTEX_POINT ( 'NONE', #28984 ) ;
#27895=CARTESIAN_POINT ( 'NONE',  ( -13.62178482187498396, 198.5843750006145569, 23.59362340125808188 ) ) ;
#27896=CARTESIAN_POINT ( 'NONE',  ( 9.262227810926050964, 194.9999999999998579, 25.63589452377446065 ) ) ;
#27897=ADVANCED_FACE ( 'NONE', ( #3025 ), #549, .F. ) ;
#27901=CARTESIAN_POINT ( 'NONE',  ( 26.99999999999999645, 242.6312500012290343, -7.347880794884117764E-16 ) ) ;
#27904=CARTESIAN_POINT ( 'NONE',  ( -1.926257025242585782E-15, 198.3406250006145228, -31.45816453501075927 ) ) ;
#27924=CYLINDRICAL_SURFACE ( 'NONE', #15336, 5.999999999999999112 ) ;
#27928=CARTESIAN_POINT ( 'NONE',  ( -28.99999999999999645, 201.9999999999999716, -1.007612034238798379E-23 ) ) ;
#27936=LINE ( 'NONE', #11061, #5109 ) ;
#27937=CARTESIAN_POINT ( 'NONE',  ( 18.00000000000000000, 247.6750000000000114, -5.196152422706630247 ) ) ;
#27938=CARTESIAN_POINT ( 'NONE',  ( 15.24356964374999990, 248.5093750006145399, 0.000000000000000000 ) ) ;
#27940=CARTESIAN_POINT ( 'NONE',  ( 15.24356964374999990, 243.0718750006145399, -3.323476615752268604 ) ) ;
#27943=CARTESIAN_POINT ( 'NONE',  ( 24.00000000000000000, 248.4062500012290400, 5.196152422706629359 ) ) ;
#27962=CARTESIAN_POINT ( 'NONE',  ( 4.999999999999997335, 215.9999999999999716, -0.1963495407219245925 ) ) ;
#27964=CIRCLE ( 'NONE', #11608, 8.000000000000000000 ) ;
#27965=LINE ( 'NONE', #27784, #6296 ) ;
#27971=CARTESIAN_POINT ( 'NONE',  ( 27.24356964375000345, 195.9781250006145399, -3.336375036156643733E-15 ) ) ;
#27989=CARTESIAN_POINT ( 'NONE',  ( 13.49999999999999645, 198.5000000000000000, -23.38268590217984766 ) ) ;
#27993=FACE_OUTER_BOUND ( 'NONE', #7798, .T. ) ;
#27998=CARTESIAN_POINT ( 'NONE',  ( 21.00000000000000000, 242.6875000000000284, -6.928203230275506996 ) ) ;
#28000=( BOUNDED_CURVE ( )  B_SPLINE_CURVE ( 2, ( #35198, #145, #23655, #29517, #3365, #18163, #32546, #15120, #11709 ),
 .UNSPECIFIED., .F., .F. ) 
 B_SPLINE_CURVE_WITH_KNOTS ( ( 3, 2, 2, 2, 3 ),
 ( 0.4891304347826087029, 0.4927536231884058204, 0.5000000000000000000, 0.5072463768115942351, 0.5108695652173913526 ),
 .UNSPECIFIED. ) 
 CURVE ( )  GEOMETRIC_REPRESENTATION_ITEM ( )  RATIONAL_B_SPLINE_CURVE ( ( 0.9330127018922194093, 0.9330127018922194093, 1.000000000000000000, 0.8660254037844387076, 1.000000000000000000, 0.8660254037844387076, 1.000000000000000000, 0.9330127018922182991, 0.9330127018922192983 ) ) 
 REPRESENTATION_ITEM ( '' )  );
#28005=CARTESIAN_POINT ( 'NONE',  ( -13.49999999999998401, 197.9375000012290400, 23.38268590217985476 ) ) ;
#28009=CARTESIAN_POINT ( 'NONE',  ( 15.24356964374999990, 242.6218750006145228, -3.323476615752268604 ) ) ;
#28014=VECTOR ( 'NONE', #15802, 1000.000000000000000 ) ;
#28016=CARTESIAN_POINT ( 'NONE',  ( 27.24356964375000345, 198.7343750006145626, -3.336375036156643733E-15 ) ) ;
#28035=ORIENTED_EDGE ( 'NONE', *, *, #21252, .F. ) ;
#28038=CARTESIAN_POINT ( 'NONE',  ( -27.24356964374999279, 198.0968750006145456, 15.72908226750539384 ) ) ;
#28042=CARTESIAN_POINT ( 'NONE',  ( 26.99999999999999645, 249.8124999999999716, -3.464101615137755275 ) ) ;
#28046=ORIENTED_EDGE ( 'NONE', *, *, #2962, .T. ) ;
#28048=CARTESIAN_POINT ( 'NONE',  ( 23.87821517812500005, 244.4968750006145228, 4.985214923628404016 ) ) ;
#28055=ORIENTED_EDGE ( 'NONE', *, *, #8524, .F. ) ;
#28060=CARTESIAN_POINT ( 'NONE',  ( 20.99999999999999645, 244.2343750006145626, -6.646953231504538984 ) ) ;
#28061=FACE_OUTER_BOUND ( 'NONE', #37448, .T. ) ;
#28068=CARTESIAN_POINT ( 'NONE',  ( -7.234628195640302017, 199.6424038105676857, 27.00000000000000711 ) ) ;
#28073=ORIENTED_EDGE ( 'NONE', *, *, #12017, .F. ) ;
#28080=CARTESIAN_POINT ( 'NONE',  ( -13.62178482187498396, 197.2343750006145626, 23.59362340125808188 ) ) ;
#28083=CARTESIAN_POINT ( 'NONE',  ( 22.60769515458672885, 242.0325961894323257, 5.999999999999997335 ) ) ;
#28086=ORIENTED_EDGE ( 'NONE', *, *, #34278, .T. ) ;
#28087=CARTESIAN_POINT ( 'NONE',  ( 21.00000000000000000, 242.0687500012290343, 6.928203230275506996 ) ) ;
#28090=CARTESIAN_POINT ( 'NONE',  ( -27.24356964374999990, 199.3156250006145171, -15.72908226750537786 ) ) ;
#28093=ORIENTED_EDGE ( 'NONE', *, *, #28167, .T. ) ;
#28119=CARTESIAN_POINT ( 'NONE',  ( 0.000000000000000000, 210.0000000000000284, 0.000000000000000000 ) ) ;
#28123=CARTESIAN_POINT ( 'NONE',  ( 19.39230484541326049, 247.6575961894323541, -5.999999999999994671 ) ) ;
#28124=CARTESIAN_POINT ( 'NONE',  ( 26.75643035624999655, 247.3843750006145399, -7.049594010296217766E-16 ) ) ;
#28126=CARTESIAN_POINT ( 'NONE',  ( 15.24356964374999990, 240.8218750006145683, -3.323476615752268604 ) ) ;
#28128=CARTESIAN_POINT ( 'NONE',  ( 20.99999999999999645, 185.0294372515228645, 0.000000000000000000 ) ) ;
#28130=CARTESIAN_POINT ( 'NONE',  ( 23.99999999999999645, 248.1062500012290570, -5.196152422706631135 ) ) ;
#28134=CARTESIAN_POINT ( 'NONE',  ( 24.00000000000000000, 240.7562500012290627, 5.196152422706629359 ) ) ;
#28138=ORIENTED_EDGE ( 'NONE', *, *, #12715, .T. ) ;
#28143=CARTESIAN_POINT ( 'NONE',  ( 26.75643035624999655, 248.2093750006145285, -3.323476615752271712 ) ) ;
#28146=CARTESIAN_POINT ( 'NONE',  ( 15.15359421270861340, 225.5904154327739661, 1.363118671454984554 ) ) ;
#28150=EDGE_CURVE ( 'NONE', #17896, #6008, #25230, .T. ) ;
#28154=CARTESIAN_POINT ( 'NONE',  ( 13.62178482187499640, 195.6031250006145115, -23.59362340125807123 ) ) ;
#28167=EDGE_CURVE ( 'NONE', #22802, #6301, #9518, .T. ) ;
#28174=CARTESIAN_POINT ( 'NONE',  ( -13.50000000000000533, 198.5749999999999886, -23.38268590217984411 ) ) ;
#28180=DIRECTION ( 'NONE',  ( -0.000000000000000000, -0.000000000000000000, 1.000000000000000000 ) ) ;
#28184=CARTESIAN_POINT ( 'NONE',  ( 15.00000000000000000, 242.7625000000000171, -3.464101615137752166 ) ) ;
#28185=CARTESIAN_POINT ( 'NONE',  ( 20.99999999999999289, 243.6437500012290229, -5.999999999999997335 ) ) ;
#28189=ORIENTED_EDGE ( 'NONE', *, *, #11222, .T. ) ;
#28191=CARTESIAN_POINT ( 'NONE',  ( 13.50000000000001421, 195.7625000012290570, 23.38268590217984055 ) ) ;
#28192=DIRECTION ( 'NONE',  ( -0.000000000000000000, 1.000000000000000000, -0.000000000000000000 ) ) ;
#28196=CARTESIAN_POINT ( 'NONE',  ( 23.87821517812499650, 242.5093750006145399, -4.985214923628404904 ) ) ;
#28205=CARTESIAN_POINT ( 'NONE',  ( 13.62178482187501416, 199.1093750006145342, 23.59362340125806767 ) ) ;
#28218=( BOUNDED_CURVE ( )  B_SPLINE_CURVE ( 2, ( #3080, #2890, #8588, #237, #26200, #11612, #23187, #34920, #422 ),
 .UNSPECIFIED., .F., .F. ) 
 B_SPLINE_CURVE_WITH_KNOTS ( ( 3, 2, 2, 2, 3 ),
 ( 0.6041666666666667407, 0.6111111111111111605, 0.6250000000000000000, 0.6388888888888888395, 0.6458333333333333703 ),
 .UNSPECIFIED. ) 
 CURVE ( )  GEOMETRIC_REPRESENTATION_ITEM ( )  RATIONAL_B_SPLINE_CURVE ( ( 0.9330127018922192983, 0.9330127018922198534, 1.000000000000000000, 0.8660254037844387076, 1.000000000000000000, 0.8660254037844387076, 1.000000000000000000, 0.9330127018922187432, 0.9330127018922192983 ) ) 
 REPRESENTATION_ITEM ( '' )  );
#28221=CARTESIAN_POINT ( 'NONE',  ( 20.99999999999999289, 248.5937500012290400, -5.999999999999997335 ) ) ;
#28225=CARTESIAN_POINT ( 'NONE',  ( 27.24356964374999279, 196.9718750006145456, -15.72908226750539207 ) ) ;
#28228=CYLINDRICAL_SURFACE ( 'NONE', #7766, 8.000000000000000000 ) ;
#28229=CARTESIAN_POINT ( 'NONE',  ( 26.75643035624999655, 241.4968750006145228, 3.323476615752267715 ) ) ;
#28233=ORIENTED_EDGE ( 'NONE', *, *, #31699, .T. ) ;
#28235=CARTESIAN_POINT ( 'NONE',  ( 26.75643035624999655, 245.4343750006145228, 3.323476615752267715 ) ) ;
#28241=CARTESIAN_POINT ( 'NONE',  ( 26.99999999999999645, 244.4124999999999943, -3.464101615137755275 ) ) ;
#28247=ADVANCED_FACE ( 'NONE', ( #1294 ), #35602, .F. ) ;
#28249=CARTESIAN_POINT ( 'NONE',  ( 20.99999999999999645, 244.0093750006145115, 6.646953231504538984 ) ) ;
#28261=CARTESIAN_POINT ( 'NONE',  ( 22.60769515458672174, 245.6888461906614225, 6.000000000000004441 ) ) ;
#28263=DIRECTION ( 'NONE',  ( 0.000000000000000000, 0.000000000000000000, -1.000000000000000000 ) ) ;
#28267=CARTESIAN_POINT ( 'NONE',  ( 18.00000000000000000, 246.8312500012290513, -5.196152422706630247 ) ) ;
#28268=CARTESIAN_POINT ( 'NONE',  ( -13.62178482187500528, 197.9843750006145626, -23.59362340125807123 ) ) ;
#28269=DIRECTION ( 'NONE',  ( 0.000000000000000000, 0.000000000000000000, -1.000000000000000000 ) ) ;
#28273=CARTESIAN_POINT ( 'NONE',  ( 26.99999999999999645, 241.3187500012290627, -3.464101615137755275 ) ) ;
#28280=AXIS2_PLACEMENT_3D ( 'NONE', #18193, #32956, #30308 ) ;
#28290=CARTESIAN_POINT ( 'NONE',  ( -28.99999999999999289, 201.9999999999999432, 0.5242534236750171495 ) ) ;
#28291=CARTESIAN_POINT ( 'NONE',  ( -13.66544594067261720, 216.1537252680216739, -5.164798763356904132 ) ) ;
#28300=ORIENTED_EDGE ( 'NONE', *, *, #22225, .F. ) ;
#28306=CARTESIAN_POINT ( 'NONE',  ( 20.99999999999999645, 192.3000000000000398, 0.000000000000000000 ) ) ;
#28307=CARTESIAN_POINT ( 'NONE',  ( 15.24356964375000167, 248.0968750006145456, 3.323476615752272600 ) ) ;
#28309=CARTESIAN_POINT ( 'NONE',  ( 26.75643035624999655, 241.4968750006144944, 3.323476615752267271 ) ) ;
#28311=ORIENTED_EDGE ( 'NONE', *, *, #25444, .F. ) ;
#28313=CARTESIAN_POINT ( 'NONE',  ( -27.00000000000000355, 199.9625000000000057, -15.58845726811989429 ) ) ;
#28319=ORIENTED_EDGE ( 'NONE', *, *, #2507, .F. ) ;
#28321=VERTEX_POINT ( 'NONE', #921 ) ;
#28325=CARTESIAN_POINT ( 'NONE',  ( 20.99999999999998579, 248.0875000000000057, -5.999999999999997335 ) ) ;
#28326=CARTESIAN_POINT ( 'NONE',  ( 18.12178482187499640, 249.6718750006145342, -4.985214923628404904 ) ) ;
#28329=CARTESIAN_POINT ( 'NONE',  ( 5.840947329778490626, 215.6846447513327121, -1.929602858956001032 ) ) ;
#28339=CARTESIAN_POINT ( 'NONE',  ( -1.926257025242585782E-15, 195.6406250006145058, -31.45816453501075927 ) ) ;
#28354=CARTESIAN_POINT ( 'NONE',  ( 15.00000000000000000, 249.0999999999999943, 0.000000000000000000 ) ) ;
#28356=CARTESIAN_POINT ( 'NONE',  ( 27.00000000000000355, 197.0749999999999886, -3.306546357697854128E-15 ) ) ;
#28360=CARTESIAN_POINT ( 'NONE',  ( 15.24356964374999990, 249.8593750006145342, 0.000000000000000000 ) ) ;
#28361=ORIENTED_EDGE ( 'NONE', *, *, #14499, .T. ) ;
#28367=CARTESIAN_POINT ( 'NONE',  ( 26.99999999999999645, 243.4749999999999943, -7.347880794884117764E-16 ) ) ;
#28370=ORIENTED_EDGE ( 'NONE', *, *, #29328, .F. ) ;
#28372=CARTESIAN_POINT ( 'NONE',  ( -13.50000000000000533, 195.5375000012290343, -23.38268590217984411 ) ) ;
#28376=CARTESIAN_POINT ( 'NONE',  ( 23.87821517812500005, 242.8093750006145228, 4.985214923628404016 ) ) ;
#28378=EDGE_CURVE ( 'NONE', #9298, #25022, #14829, .T. ) ;
#28384=CARTESIAN_POINT ( 'NONE',  ( 27.24356964374999635, 198.7718750006145569, -15.72908226750539029 ) ) ;
#28387=LINE ( 'NONE', #5634, #6849 ) ;
#28396=CARTESIAN_POINT ( 'NONE',  ( 24.00000000000000000, 248.7999999999999829, 5.196152422706629359 ) ) ;
#28401=CARTESIAN_POINT ( 'NONE',  ( 13.62178482187499640, 195.2093750006145569, -23.59362340125807123 ) ) ;
#28405=CARTESIAN_POINT ( 'NONE',  ( 26.75643035624999655, 241.0843750006145285, -7.049594010296217766E-16 ) ) ;
#28406=CARTESIAN_POINT ( 'NONE',  ( -27.24356964375000345, 199.3156250006145171, -15.72908226750537786 ) ) ;
#28411=CARTESIAN_POINT ( 'NONE',  ( 15.24356964374999990, 244.7593750006145115, -3.323476615752268604 ) ) ;
#28414=( BOUNDED_CURVE ( )  B_SPLINE_CURVE ( 2, ( #36954, #25404, #11001, #34119, #21830, #27694, #24847, #2832, #34491 ),
 .UNSPECIFIED., .F., .F. ) 
 B_SPLINE_CURVE_WITH_KNOTS ( ( 3, 2, 2, 2, 3 ),
 ( 0.9239130434782608647, 0.9275362318840579823, 0.9347826086956522174, 0.9420289855072463414, 0.9456521739130434590 ),
 .UNSPECIFIED. ) 
 CURVE ( )  GEOMETRIC_REPRESENTATION_ITEM ( )  RATIONAL_B_SPLINE_CURVE ( ( 0.9330127018922194093, 0.9330127018922194093, 1.000000000000000000, 0.8660254037844387076, 1.000000000000000000, 0.8660254037844387076, 1.000000000000000000, 0.9330127018922194093, 0.9330127018922194093 ) ) 
 REPRESENTATION_ITEM ( '' )  );
#28422=CARTESIAN_POINT ( 'NONE',  ( 15.24356964375000167, 244.3843750006145115, 3.323476615752272600 ) ) ;
#28430=CARTESIAN_POINT ( 'NONE',  ( 20.99999999999999289, 240.0437500012290570, -5.999999999999997335 ) ) ;
#28439=ORIENTED_EDGE ( 'NONE', *, *, #31868, .F. ) ;
#28443=ADVANCED_FACE ( 'NONE', ( #27456, #13058 ), #24615, .F. ) ;
#28446=CARTESIAN_POINT ( 'NONE',  ( -27.24356964375000345, 195.3593750006145342, 0.000000000000000000 ) ) ;
#28448=EDGE_CURVE ( 'NONE', #2167, #2407, #36535, .T. ) ;
#28451=CARTESIAN_POINT ( 'NONE',  ( 20.99999999999999645, 239.8187500012290059, 5.999999999999998224 ) ) ;
#28453=CARTESIAN_POINT ( 'NONE',  ( 24.00000000000000000, 242.5562500012290457, 5.196152422706629359 ) ) ;
#28462=CARTESIAN_POINT ( 'NONE',  ( 15.00000000000000178, 246.0437500012290570, 3.464101615137757051 ) ) ;
#28480=CARTESIAN_POINT ( 'NONE',  ( 20.99999999999999645, 240.6624999999999943, 5.999999999999998224 ) ) ;
#28485=CYLINDRICAL_SURFACE ( 'NONE', #35953, 27.00000000000000000 ) ;
#28488=CARTESIAN_POINT ( 'NONE',  ( 21.00000000000000000, 245.6968750006145399, -6.646953231504538984 ) ) ;
#28490=CARTESIAN_POINT ( 'NONE',  ( 20.99999999999999645, 241.6468750006145285, -6.646953231504538984 ) ) ;
#28492=ORIENTED_EDGE ( 'NONE', *, *, #21063, .T. ) ;
#28495=CARTESIAN_POINT ( 'NONE',  ( 15.00000000000000000, 249.1187500012290741, -3.464101615137752166 ) ) ;
#28503=ORIENTED_EDGE ( 'NONE', *, *, #13446, .F. ) ;
#28506=CARTESIAN_POINT ( 'NONE',  ( -27.00000000000000355, 199.8312500006145171, 0.000000000000000000 ) ) ;
#28508=CARTESIAN_POINT ( 'NONE',  ( 18.12178482187499640, 248.3218750006145115, -4.985214923628404904 ) ) ;
#28511=CARTESIAN_POINT ( 'NONE',  ( 5.536961926789909505, 215.7986392774538729, 1.553813268097265832 ) ) ;
#28534=CARTESIAN_POINT ( 'NONE',  ( 13.49999999999999645, 197.5999999999999943, -23.38268590217984766 ) ) ;
#28535=DIRECTION ( 'NONE',  ( -1.000000000000000000, -0.000000000000000000, -0.000000000000000000 ) ) ;
#28538=CARTESIAN_POINT ( 'NONE',  ( 15.24356964374999990, 248.9593750006145285, 0.000000000000000000 ) ) ;
#28539=ORIENTED_EDGE ( 'NONE', *, *, #11717, .T. ) ;
#28546=CARTESIAN_POINT ( 'NONE',  ( 26.99999999999999645, 242.5374999999999943, 3.464101615137751278 ) ) ;
#28547=CARTESIAN_POINT ( 'NONE',  ( 1.069080835302379631E-14, 199.2125000000000057, 27.00000000000000000 ) ) ;
#28552=CARTESIAN_POINT ( 'NONE',  ( -27.00000000000000355, 196.5125000012290570, 0.000000000000000000 ) ) ;
#28553=CARTESIAN_POINT ( 'NONE',  ( -5.732297079746171420, 222.9518338469886203, -2.500000000000000000 ) ) ;
#28556=CARTESIAN_POINT ( 'NONE',  ( 21.00000000000000000, 241.6468750006145285, -6.646953231504538984 ) ) ;
#28562=EDGE_CURVE ( 'NONE', #7301, #11787, #19728, .T. ) ;
#28564=CARTESIAN_POINT ( 'NONE',  ( 24.55568120905228113, 195.0000000000000853, 11.66401174564247789 ) ) ;
#28565=CARTESIAN_POINT ( 'NONE',  ( -27.24356964374999990, 198.9218750006145626, -15.72908226750537786 ) ) ;
#28570=CARTESIAN_POINT ( 'NONE',  ( 20.99999999999999645, 248.3687500012290457, 5.999999999999998224 ) ) ;
#28574=CARTESIAN_POINT ( 'NONE',  ( -3.253724281355068545E-15, 197.3000000012290229, -27.00000000000000000 ) ) ;
#28579=CARTESIAN_POINT ( 'NONE',  ( 20.99999999999999289, 249.8874999999999886, -5.999999999999997335 ) ) ;
#28584=CARTESIAN_POINT ( 'NONE',  ( -13.62178482187498396, 196.3343750006145285, 23.59362340125808188 ) ) ;
#28587=FACE_OUTER_BOUND ( 'NONE', #25275, .T. ) ;
#28588=CARTESIAN_POINT ( 'NONE',  ( 15.24356964374999990, 239.9218750006145626, -3.323476615752268604 ) ) ;
#28589=CARTESIAN_POINT ( 'NONE',  ( 27.24356964375000700, 199.0906250006145228, 15.72908226750537075 ) ) ;
#28593=ORIENTED_EDGE ( 'NONE', *, *, #34661, .T. ) ;
#28594=ORIENTED_EDGE ( 'NONE', *, *, #32287, .T. ) ;
#28595=CARTESIAN_POINT ( 'NONE',  ( 21.00000000000000000, 241.0843750006145285, -6.646953231504538984 ) ) ;
#28605=CARTESIAN_POINT ( 'NONE',  ( 18.12178482187499640, 244.7218750006145171, -4.985214923628404904 ) ) ;
#28606=CARTESIAN_POINT ( 'NONE',  ( 23.99999999999999645, 246.7562500012290627, -5.196152422706631135 ) ) ;
#28613=CYLINDRICAL_SURFACE ( 'NONE', #29891, 27.00000000000000000 ) ;
#28621=CARTESIAN_POINT ( 'NONE',  ( 20.99999999999997868, 245.6687500012291139, 5.999999999999999112 ) ) ;
#28630=CARTESIAN_POINT ( 'NONE',  ( -27.24356964375000345, 196.2593750006145399, 0.000000000000000000 ) ) ;
#28635=VERTEX_POINT ( 'NONE', #22337 ) ;
#28636=ORIENTED_EDGE ( 'NONE', *, *, #22077, .F. ) ;
#28637=CARTESIAN_POINT ( 'NONE',  ( 15.24356964375000167, 248.8843750006145399, 3.323476615752272600 ) ) ;
#28655=ORIENTED_EDGE ( 'NONE', *, *, #5296, .T. ) ;
#28661=VECTOR ( 'NONE', #24591, 1000.000000000000000 ) ;
#28669=CARTESIAN_POINT ( 'NONE',  ( 18.00000000000000000, 240.0812500012290513, -5.196152422706630247 ) ) ;
#28670=CARTESIAN_POINT ( 'NONE',  ( 15.24356964375000167, 245.3968750006145285, 3.323476615752272600 ) ) ;
#28672=CARTESIAN_POINT ( 'NONE',  ( 23.87821517812500005, 241.0093750006145399, 4.985214923628404016 ) ) ;
#28673=ORIENTED_EDGE ( 'NONE', *, *, #11736, .F. ) ;
#28676=CARTESIAN_POINT ( 'NONE',  ( 15.00000000000000000, 246.9062500012290400, 0.000000000000000000 ) ) ;
#28693=CARTESIAN_POINT ( 'NONE',  ( 0.000000000000000000, 210.0000000000000284, -28.99999999999999645 ) ) ;
#28695=AXIS2_PLACEMENT_3D ( 'NONE', #16780, #22842, #29393 ) ;
#28696=EDGE_CURVE ( 'NONE', #29694, #36021, #29304, .T. ) ;
#28722=CARTESIAN_POINT ( 'NONE',  ( 27.00000000000001066, 198.3875000000000171, 15.58845726811988897 ) ) ;
#28725=CARTESIAN_POINT ( 'NONE',  ( 26.75643035624999655, 248.6968750006145115, 3.323476615752267271 ) ) ;
#28732=CARTESIAN_POINT ( 'NONE',  ( 15.00000000000000178, 243.7374999999999829, 3.464101615137757051 ) ) ;
#28735=VERTEX_POINT ( 'NONE', #20426 ) ;
#28738=CARTESIAN_POINT ( 'NONE',  ( -1.909035429704832693E-15, 195.9500000012290002, -31.17691453623979214 ) ) ;
#28742=CARTESIAN_POINT ( 'NONE',  ( 26.75643035624999655, 243.3718750006145228, -3.323476615752271712 ) ) ;
#28748=VECTOR ( 'NONE', #36335, 1000.000000000000000 ) ;
#28751=CARTESIAN_POINT ( 'NONE',  ( 21.07789340583945403, 194.9999999999999716, 17.32733911463861887 ) ) ;
#28752=CARTESIAN_POINT ( 'NONE',  ( -27.24356964375000345, 196.7093750006145569, 0.000000000000000000 ) ) ;
#28762=CARTESIAN_POINT ( 'NONE',  ( 13.50000000000001421, 197.1125000012290513, 23.38268590217984055 ) ) ;
#28768=VERTEX_POINT ( 'NONE', #8303 ) ;
#28771=CARTESIAN_POINT ( 'NONE',  ( 26.99999999999999645, 196.2125000000000057, -15.58845726811990495 ) ) ;
#28775=CARTESIAN_POINT ( 'NONE',  ( 21.00000000000000000, 241.4218750006145626, 6.646953231504538984 ) ) ;
#28776=CARTESIAN_POINT ( 'NONE',  ( 27.24356964374999279, 198.2656250006145058, -15.72908226750539207 ) ) ;
#28778=AXIS2_PLACEMENT_3D ( 'NONE', #1695, #13083, #1509 ) ;
#28784=CARTESIAN_POINT ( 'NONE',  ( 13.62178482187501416, 197.2531250006145456, 23.59362340125806767 ) ) ;
#28785=CARTESIAN_POINT ( 'NONE',  ( 26.75643035624999655, 242.7343750006145342, 3.323476615752267715 ) ) ;
#28792=CARTESIAN_POINT ( 'NONE',  ( 15.24356964374999990, 242.5093750006145115, -3.323476615752268604 ) ) ;
#28800=CARTESIAN_POINT ( 'NONE',  ( 26.99999999999999645, 239.9312500012290457, -7.347880794884117764E-16 ) ) ;
#28805=CARTESIAN_POINT ( 'NONE',  ( 26.99999999999999645, 244.4312500012290457, -7.347880794884117764E-16 ) ) ;
#28807=CARTESIAN_POINT ( 'NONE',  ( 26.99999999999999645, 245.7812500012290400, -7.347880794884117764E-16 ) ) ;
#28813=CARTESIAN_POINT ( 'NONE',  ( 24.00000000000000000, 241.1500000000000057, 5.196152422706629359 ) ) ;
#28814=CARTESIAN_POINT ( 'NONE',  ( 19.39230484541324273, 242.4986538117967427, 5.999999999999987566 ) ) ;
#28816=CARTESIAN_POINT ( 'NONE',  ( 0.000000000000000000, 195.0000000000000000, 0.000000000000000000 ) ) ;
#28817=ADVANCED_FACE ( 'NONE', ( #9039 ), #25725, .F. ) ;
#28822=ORIENTED_EDGE ( 'NONE', *, *, #2652, .T. ) ;
#28823=CARTESIAN_POINT ( 'NONE',  ( 15.24356964374999990, 248.3968750006145285, 0.000000000000000000 ) ) ;
#28828=VECTOR ( 'NONE', #16818, 1000.000000000000000 ) ;
#28836=EDGE_CURVE ( 'NONE', #25022, #5908, #31316, .T. ) ;
#28837=CARTESIAN_POINT ( 'NONE',  ( -26.27693753440958702, 194.9999999999998863, 6.788958541037892758 ) ) ;
#28859=CARTESIAN_POINT ( 'NONE',  ( 18.12178482187500350, 246.3343750006145285, 4.985214923628407568 ) ) ;
#28861=CARTESIAN_POINT ( 'NONE',  ( 26.75643035624999655, 240.6718750006145910, -3.323476615752271268 ) ) ;
#28862=ORIENTED_EDGE ( 'NONE', *, *, #4553, .F. ) ;
#28864=CARTESIAN_POINT ( 'NONE',  ( 20.99999999999999645, 250.0000000000000000, 0.000000000000000000 ) ) ;
#28866=CARTESIAN_POINT ( 'NONE',  ( 23.99999999999999645, 246.7562500012290627, -5.196152422706631135 ) ) ;
#28880=CARTESIAN_POINT ( 'NONE',  ( 20.99999999999999289, 241.8437500012290400, -5.999999999999997335 ) ) ;
#28881=CARTESIAN_POINT ( 'NONE',  ( 18.12178482187499640, 246.5218750006145001, -4.985214923628404904 ) ) ;
#28884=B_SPLINE_CURVE_WITH_KNOTS ( 'NONE', 3,
 ( #11040, #34163, #16925, #23169, #5714, #14264, #17861, #219, #29, #26000, #2688, #8571, #11414, #25815, #31873, #17295, #14444, #35086, #34902, #22982, #17484, #28837, #3437, #5904, #29016, #34532, #2871, #3062, #15006, #11594, #34712, #26181, #11968, #9136, #3250, #35267, #19960, #14631, #11783, #31503, #8758, #20331 ),
 .UNSPECIFIED., .F., .F.,
 ( 4, 2, 2, 2, 2, 2, 2, 2, 2, 2, 2, 2, 2, 2, 2, 2, 2, 2, 2, 2, 4 ),
 ( 0.000000000000000000, 0.003356155942727553562, 0.006712311885455107124, 0.01006846782818265548, 0.01174654579954642966, 0.01342462377091020211, 0.01678077971363774179, 0.02013693565636528321, 0.02349309159909282116, 0.02517116957045658840, 0.02684924754182035564, 0.03020540348454789359, 0.03188348145591166777, 0.03356155942727542807, 0.03691771537000296949, 0.03859579334136674367, 0.04027387131273051091, 0.04363002725545805233, 0.04530810522682182651, 0.04698618319818559375, 0.05369849508364069046 ),
 .UNSPECIFIED. ) ;
#28909=CARTESIAN_POINT ( 'NONE',  ( 27.24356964375000345, 199.6343750006145399, -3.336375036156643733E-15 ) ) ;
#28912=CARTESIAN_POINT ( 'NONE',  ( 18.12178482187499640, 249.7843750006145456, -4.985214923628404904 ) ) ;
#28915=PRODUCT ( 'head', 'head', '', ( #13016 ) ) ;
#28921=CARTESIAN_POINT ( 'NONE',  ( 18.00000000000000355, 241.0750000000000171, 5.196152422706632912 ) ) ;
#28925=ORIENTED_EDGE ( 'NONE', *, *, #33554, .T. ) ;
#28927=CARTESIAN_POINT ( 'NONE',  ( -13.49999999999998401, 195.2375000012290229, 23.38268590217985476 ) ) ;
#28933=CARTESIAN_POINT ( 'NONE',  ( 23.87821517812499650, 240.7093750006145285, -4.985214923628404904 ) ) ;
#28941=CARTESIAN_POINT ( 'NONE',  ( -13.62178482187500528, 195.7343750006145626, -23.59362340125807123 ) ) ;
#28946=DIRECTION ( 'NONE',  ( 0.000000000000000000, 1.000000000000000000, 0.000000000000000000 ) ) ;
#28951=CARTESIAN_POINT ( 'NONE',  ( -4.694659320240884604E-14, 197.0750000012290570, 27.00000000000000000 ) ) ;
#28956=DIRECTION ( 'NONE',  ( 0.000000000000000000, 0.000000000000000000, 1.000000000000000000 ) ) ;
#28957=EDGE_LOOP ( 'NONE', ( #4510, #3285, #35914 ) ) ;
#28960=CARTESIAN_POINT ( 'NONE',  ( 13.62178482187501416, 195.5093750006145399, 23.59362340125806767 ) ) ;
#28963=CARTESIAN_POINT ( 'NONE',  ( 26.99999999999999645, 248.8374999999999773, 3.464101615137751278 ) ) ;
#28964=CARTESIAN_POINT ( 'NONE',  ( -1.926257025242585782E-15, 198.3406250006145228, -31.45816453501076637 ) ) ;
#28969=CARTESIAN_POINT ( 'NONE',  ( -27.24356964374999990, 197.0656250006145171, -15.72908226750537786 ) ) ;
#28970=CARTESIAN_POINT ( 'NONE',  ( 15.24356964375000167, 242.1343750006145399, 3.323476615752272600 ) ) ;
#28973=CARTESIAN_POINT ( 'NONE',  ( 18.12178482187500350, 248.5843750006145285, 4.985214923628407568 ) ) ;
#28977=( BOUNDED_SURFACE ( )  B_SPLINE_SURFACE ( 1, 2, ( 
 ( #13923, #25473, #19255, #31530, #19812, #13358, #7675, #22086, #36840, #16952, #2538, #33636, #17140, #28495, #10695, #30794, #8417, #5373, #37024, #5555, #11256, #5003, #1974, #16585, #1790, #11070, #7862, #31170, #4817, #19986, #16397, #19436, #27943, #8237, #22644, #14104, #30985, #13546, #34190, #25099, #28130, #25656, #22272, #33825, #2159, #16767, #31346, #13742, #34003, #25288, #37209, #22828, #34376, #10883, #22456, #26209, #23008, #17510, #9161, #31716, #17697, #14850, #35113, #432, #17887, #34744, #6504, #26399, #17323, #5931, #29432, #2900, #28676, #11621, #32087, #6119, #28866, #23379, #14473, #3468, #20729, #32272, #6315, #11997, #245, #34558, #29046, #15037, #5743, #29237, #23568, #32461, #26026, #23756, #34928, #20544, #26585, #23196, #8787, #8973, #54, #20359, #31902, #14658, #3090, #2714, #11809, #14290, #614, #3277, #12183, #35295, #9351, #25842, #20922, #37391, #11441, #8597, #20168, #36239, #6693, #21668, #15419, #15603, #35679, #10281, #15795, #35489, #4217, #36055, #21492, #21855, #27534, #10098, #18264, #4031, #26965, #33222, #27159, #806, #7261, #18836, #12946, #30382, #27345, #18650, #3841, #21303, #1182, #30002, #12756, #1376, #994, #24324, #7082, #24507, #33408, #35866, #4403, #23947, #9539, #15226, #9908, #1559, #15986, #12570, #24137, #30191, #13131, #21113, #24685, #18079, #9731, #12377, #29620, #29808, #32652, #32839, #6884, #3655, #18459, #33032, #26775, #13883, #5146, #34147, #27901, #33782, #28453, #22602, #1932, #7820, #2490, #8194, #36984, #22414, #5335, #2119, #19397, #19211, #19577, #28087, #13500, #7446, #14065, #16727, #30940, #30756, #4779, #25058, #19770, #7634, #16170, #36797, #22231, #27719, #13696, #10841, #4959, #36423, #1749, #28273, #16352, #33595, #16541, #31307, #16913, #11027, #25614, #36611, #8004, #10466, #2309, #25247, #22784, #37171, #33962, #31129, #30577, #25431, #11212, #13316, #10652, #19020, #22044, #4593, #24874, #25986, #11956, #9121, #3424, #8559, #23526, #11772, #6272, #34333, #17659, #26170, #8746, #32043, #20317, #14992, #29194, #17849, #29005, #37348, #16, #3236, #35072 ),
 ( #29387, #34889, #8929, #572, #20687, #32233, #26543, #206, #23157, #11582, #17098, #34699, #23338, #20506, #14250, #12139, #14809, #8378, #2675, #31489, #31858, #19949, #5513, #28637, #25799, #11400, #5702, #22971, #34518, #390, #6073, #20126, #31673, #5892, #17282, #17470, #28823, #26354, #2858, #14618, #14432, #3048, #21260, #9683, #3617, #33180, #24281, #35825, #27493, #36014, #12902, #1333, #15561, #12528, #953, #6464, #24091, #12710, #9866, #15183, #15942, #4179, #35255, #29579, #20881, #32799, #24467, #10053, #32420, #1516, #21629, #32611, #26730, #30338, #27301, #21447, #23714, #7224, #26923, #23906, #35636, #9310, #32987, #29765, #3987, #18035, #4362, #764, #3796, #12332, #30151, #7040, #18797, #15374, #35448, #18607, #9496, #6835, #21072, #6649, #18225, #18413, #27118, #1141, #29959, #15751, #36382, #25390, #31086, #5110, #16689, #36760, #10612, #7404, #1892, #28235, #16127, #2082, #10801, #16875, #10429, #8157, #19357, #4919, #22375, #7593, #33552, #7779, #24830, #19167, #30717, #36570, #4737, #28411, #22191, #24645, #19539, #30898, #13655, #16500, #28048, #10239, #31268, #13463, #2264, #13843, #33738, #5294, #1704, #36941, #22002, #25207, #16313, #13090, #33923, #30532, #7965, #10986, #22558, #36195, #34105, #19731, #13276, #21815, #27860, #33367, #18975, #4552, #27678, #25015, #17431, #11916, #2451, #23302, #31817, #14393, #164, #25950, #20650, #34849, #23483, #34659, #5475, #5663, #8887, #29152, #35035, #28785, #11363, #32196, #32006, #20466, #14769, #11730, #3010, #25760, #17243, #37493, #11544, #23116, #6036, #37312, #8704, #28970, #17623, #6230, #20278, #3193, #8340, #19910, #37128, #5853, #9080, #26132, #22934, #8522, #14580, #26314, #31451, #351, #17804, #20089, #34297, #14025, #2632, #17057, #22748, #34479, #25574, #31633, #2822, #28595, #11174, #14211, #18568, #12292, #18182, #12858, #6998, #21404, #6794, #27263, #24051, #29723, #3577, #3947, #12483, #23864, #29346, #24426, #27077, #3757, #15137, #26690, #35403, #4140, #29537, #532, #21218, #6607, #12099, #35597, #32758, #15331, #20839, #23673, #1103, #719, #17993 ) ),
 .UNSPECIFIED., .F., .F., .T. ) 
 B_SPLINE_SURFACE_WITH_KNOTS ( ( 2, 2 ),
 ( 3, 2, 2, 2, 2, 2, 2, 2, 2, 2, 2, 2, 2, 2, 2, 2, 2, 2, 2, 2, 2, 2, 2, 2, 2, 2, 2, 2, 2, 2, 2, 2, 2, 2, 2, 2, 2, 2, 2, 2, 2, 2, 2, 2, 2, 2, 2, 2, 2, 2, 2, 2, 2, 2, 2, 2, 2, 2, 2, 2, 2, 2, 2, 2, 2, 2, 2, 2, 2, 2, 2, 2, 2, 2, 2, 2, 2, 2, 2, 2, 2, 2, 2, 2, 2, 2, 2, 2, 2, 2, 2, 2, 2, 2, 2, 2, 2, 2, 2, 2, 2, 2, 2, 2, 2, 2, 2, 2, 2, 2, 2, 2, 2, 2, 2, 2, 2, 2, 2, 2, 2, 2, 2, 2, 2, 2, 2, 2, 2, 2, 2, 2, 2, 2, 3 ),
 ( 0.000000000000000000, 1.000000000000000000 ),
 ( 0.000000000000000000, 0.007246376811594202987, 0.01449275362318840597, 0.02173913043478260809, 0.02898550724637681195, 0.03623188405797101580, 0.04347826086956521618, 0.05072463768115942351, 0.05797101449275362389, 0.06521739130434782428, 0.07246376811594203160, 0.07971014492753622505, 0.08695652173913043237, 0.09420289855072463969, 0.1014492753623188470, 0.1086956521739130405, 0.1159420289855072478, 0.1231884057971014551, 0.1304347826086956486, 0.1376811594202898559, 0.1449275362318840632, 0.1521739130434782705, 0.1594202898550724501, 0.1666666666666666574, 0.1739130434782608647, 0.1811594202898550721, 0.1884057971014492794, 0.1956521739130434867, 0.2028985507246376940, 0.2101449275362318736, 0.2173913043478260809, 0.2246376811594202882, 0.2318840579710144956, 0.2391304347826087029, 0.2463768115942029102, 0.2536231884057971175, 0.2608695652173912971, 0.2681159420289855322, 0.2753623188405797118, 0.2826086956521738913, 0.2898550724637681264, 0.2971014492753623060, 0.3043478260869565410, 0.3115942028985507206, 0.3188405797101449002, 0.3260869565217391353, 0.3333333333333333148, 0.3405797101449275499, 0.3478260869565217295, 0.3550724637681159646, 0.3623188405797101441, 0.3695652173913043237, 0.3768115942028985588, 0.3840579710144927383, 0.3913043478260869734, 0.3985507246376811530, 0.4057971014492753881, 0.4130434782608695676, 0.4202898550724637472, 0.4275362318840579823, 0.4347826086956521618, 0.4420289855072463969, 0.4492753623188405765, 0.4565217391304347561, 0.4637681159420289911, 0.4710144927536231707, 0.4782608695652174058, 0.4855072463768115854, 0.4927536231884058204, 0.5000000000000000000, 0.5072463768115942351, 0.5144927536231883591, 0.5217391304347825942, 0.5289855072463768293, 0.5362318840579710644, 0.5434782608695651884, 0.5507246376811594235, 0.5579710144927536586, 0.5652173913043477826, 0.5724637681159420177, 0.5797101449275362528, 0.5869565217391304879, 0.5942028985507246119, 0.6014492753623188470, 0.6086956521739130821, 0.6159420289855072062, 0.6231884057971014412, 0.6304347826086956763, 0.6376811594202898004, 0.6449275362318840354, 0.6521739130434782705, 0.6594202898550725056, 0.6666666666666666297, 0.6739130434782608647, 0.6811594202898550998, 0.6884057971014492239, 0.6956521739130434590, 0.7028985507246376940, 0.7101449275362319291, 0.7173913043478260532, 0.7246376811594202882, 0.7318840579710145233, 0.7391304347826086474, 0.7463768115942028825, 0.7536231884057971175, 0.7608695652173913526, 0.7681159420289854767, 0.7753623188405797118, 0.7826086956521739468, 0.7898550724637680709, 0.7971014492753623060, 0.8043478260869565410, 0.8115942028985507761, 0.8188405797101449002, 0.8260869565217391353, 0.8333333333333333703, 0.8405797101449274944, 0.8478260869565217295, 0.8550724637681159646, 0.8623188405797101996, 0.8695652173913043237, 0.8768115942028985588, 0.8840579710144927938, 0.8913043478260869179, 0.8985507246376811530, 0.9057971014492753881, 0.9130434782608695121, 0.9202898550724637472, 0.9275362318840579823, 0.9347826086956522174, 0.9420289855072463414, 0.9492753623188405765, 0.9565217391304348116, 0.9637681159420289356, 0.9662082966761270653 ),
 .UNSPECIFIED. ) 
 GEOMETRIC_REPRESENTATION_ITEM ( )  RATIONAL_B_SPLINE_SURFACE ( (
 ( 1.000000000000000000, 0.8660254037844387076, 1.000000000000000000, 0.8660254037844387076, 1.000000000000000000, 0.8660254037844387076, 1.000000000000000000, 0.8660254037844387076, 1.000000000000000000, 0.8660254037844387076, 1.000000000000000000, 0.8660254037844387076, 1.000000000000000000, 0.8660254037844387076, 1.000000000000000000, 0.8660254037844387076, 1.000000000000000000, 0.8660254037844387076, 1.000000000000000000, 0.8660254037844387076, 1.000000000000000000, 0.8660254037844387076, 1.000000000000000000, 0.8660254037844387076, 1.000000000000000000, 0.8660254037844387076, 1.000000000000000000, 0.8660254037844387076, 1.000000000000000000, 0.8660254037844387076, 1.000000000000000000, 0.8660254037844387076, 1.000000000000000000, 0.8660254037844387076, 1.000000000000000000, 0.8660254037844387076, 1.000000000000000000, 0.8660254037844387076, 1.000000000000000000, 0.8660254037844387076, 1.000000000000000000, 0.8660254037844387076, 1.000000000000000000, 0.8660254037844387076, 1.000000000000000000, 0.8660254037844387076, 1.000000000000000000, 0.8660254037844387076, 1.000000000000000000, 0.8660254037844387076, 1.000000000000000000, 0.8660254037844387076, 1.000000000000000000, 0.8660254037844387076, 1.000000000000000000, 0.8660254037844387076, 1.000000000000000000, 0.8660254037844387076, 1.000000000000000000, 0.8660254037844387076, 1.000000000000000000, 0.8660254037844387076, 1.000000000000000000, 0.8660254037844387076, 1.000000000000000000, 0.8660254037844387076, 1.000000000000000000, 0.8660254037844387076, 1.000000000000000000, 0.8660254037844387076, 1.000000000000000000, 0.8660254037844387076, 1.000000000000000000, 0.8660254037844387076, 1.000000000000000000, 0.8660254037844387076, 1.000000000000000000, 0.8660254037844387076, 1.000000000000000000, 0.8660254037844387076, 1.000000000000000000, 0.8660254037844387076, 1.000000000000000000, 0.8660254037844387076, 1.000000000000000000, 0.8660254037844387076, 1.000000000000000000, 0.8660254037844387076, 1.000000000000000000, 0.8660254037844387076, 1.000000000000000000, 0.8660254037844387076, 1.000000000000000000, 0.8660254037844387076, 1.000000000000000000, 0.8660254037844387076, 1.000000000000000000, 0.8660254037844387076, 1.000000000000000000, 0.8660254037844387076, 1.000000000000000000, 0.8660254037844387076, 1.000000000000000000, 0.8660254037844387076, 1.000000000000000000, 0.8660254037844387076, 1.000000000000000000, 0.8660254037844387076, 1.000000000000000000, 0.8660254037844387076, 1.000000000000000000, 0.8660254037844387076, 1.000000000000000000, 0.8660254037844387076, 1.000000000000000000, 0.8660254037844387076, 1.000000000000000000, 0.8660254037844387076, 1.000000000000000000, 0.8660254037844387076, 1.000000000000000000, 0.8660254037844387076, 1.000000000000000000, 0.8660254037844387076, 1.000000000000000000, 0.8660254037844387076, 1.000000000000000000, 0.8660254037844387076, 1.000000000000000000, 0.8660254037844387076, 1.000000000000000000, 0.8660254037844387076, 1.000000000000000000, 0.8660254037844387076, 1.000000000000000000, 0.8660254037844387076, 1.000000000000000000, 0.8660254037844387076, 1.000000000000000000, 0.8660254037844387076, 1.000000000000000000, 0.8660254037844387076, 1.000000000000000000, 0.8660254037844387076, 1.000000000000000000, 0.8660254037844387076, 1.000000000000000000, 0.8660254037844387076, 1.000000000000000000, 0.8660254037844387076, 1.000000000000000000, 0.8660254037844387076, 1.000000000000000000, 0.8660254037844387076, 1.000000000000000000, 0.8660254037844387076, 1.000000000000000000, 0.8660254037844387076, 1.000000000000000000, 0.8660254037844387076, 1.000000000000000000, 0.8660254037844387076, 1.000000000000000000, 0.8660254037844387076, 1.000000000000000000, 0.8660254037844387076, 1.000000000000000000, 0.8660254037844387076, 1.000000000000000000, 0.8660254037844387076, 1.000000000000000000, 0.8660254037844387076, 1.000000000000000000, 0.8660254037844387076, 1.000000000000000000, 0.8660254037844387076, 1.000000000000000000, 0.8660254037844387076, 1.000000000000000000, 0.8660254037844387076, 1.000000000000000000, 0.8660254037844387076, 1.000000000000000000, 0.8660254037844387076, 1.000000000000000000, 0.8660254037844387076, 1.000000000000000000, 0.8660254037844387076, 1.000000000000000000, 0.8660254037844387076, 1.000000000000000000, 0.8660254037844387076, 1.000000000000000000, 0.8660254037844387076, 1.000000000000000000, 0.8660254037844387076, 1.000000000000000000, 0.8660254037844387076, 1.000000000000000000, 0.8660254037844387076, 1.000000000000000000, 0.8660254037844387076, 1.000000000000000000, 0.8660254037844387076, 1.000000000000000000, 0.8660254037844387076, 1.000000000000000000, 0.8660254037844387076, 1.000000000000000000, 0.8660254037844387076, 1.000000000000000000, 0.8660254037844387076, 1.000000000000000000, 0.8660254037844387076, 1.000000000000000000, 0.8660254037844387076, 1.000000000000000000, 0.8660254037844387076, 1.000000000000000000, 0.8660254037844387076, 1.000000000000000000, 0.8660254037844387076, 1.000000000000000000, 0.8660254037844387076, 1.000000000000000000, 0.8660254037844387076, 1.000000000000000000, 0.8660254037844387076, 1.000000000000000000, 0.8660254037844387076, 1.000000000000000000, 0.8660254037844387076, 1.000000000000000000, 0.8660254037844387076, 1.000000000000000000, 0.8660254037844387076, 1.000000000000000000, 0.8660254037844387076, 1.000000000000000000, 0.8660254037844387076, 1.000000000000000000, 0.8660254037844387076, 1.000000000000000000, 0.8660254037844387076, 1.000000000000000000, 0.8660254037844387076, 1.000000000000000000, 0.8660254037844387076, 1.000000000000000000, 0.8660254037844387076, 1.000000000000000000, 0.8660254037844387076, 1.000000000000000000, 0.8660254037844387076, 1.000000000000000000, 0.8660254037844387076, 1.000000000000000000, 0.8660254037844387076, 1.000000000000000000, 0.8660254037844387076, 1.000000000000000000, 0.8660254037844387076, 1.000000000000000000, 0.8660254037844387076, 1.000000000000000000, 0.8660254037844387076, 1.000000000000000000, 0.9548847324609573972, 0.9401541411607521326),
 ( 1.000000000000000000, 0.8660254037844387076, 1.000000000000000000, 0.8660254037844387076, 1.000000000000000000, 0.8660254037844387076, 1.000000000000000000, 0.8660254037844387076, 1.000000000000000000, 0.8660254037844387076, 1.000000000000000000, 0.8660254037844387076, 1.000000000000000000, 0.8660254037844387076, 1.000000000000000000, 0.8660254037844387076, 1.000000000000000000, 0.8660254037844387076, 1.000000000000000000, 0.8660254037844387076, 1.000000000000000000, 0.8660254037844387076, 1.000000000000000000, 0.8660254037844387076, 1.000000000000000000, 0.8660254037844387076, 1.000000000000000000, 0.8660254037844387076, 1.000000000000000000, 0.8660254037844387076, 1.000000000000000000, 0.8660254037844387076, 1.000000000000000000, 0.8660254037844387076, 1.000000000000000000, 0.8660254037844387076, 1.000000000000000000, 0.8660254037844387076, 1.000000000000000000, 0.8660254037844387076, 1.000000000000000000, 0.8660254037844387076, 1.000000000000000000, 0.8660254037844387076, 1.000000000000000000, 0.8660254037844387076, 1.000000000000000000, 0.8660254037844387076, 1.000000000000000000, 0.8660254037844387076, 1.000000000000000000, 0.8660254037844387076, 1.000000000000000000, 0.8660254037844387076, 1.000000000000000000, 0.8660254037844387076, 1.000000000000000000, 0.8660254037844387076, 1.000000000000000000, 0.8660254037844387076, 1.000000000000000000, 0.8660254037844387076, 1.000000000000000000, 0.8660254037844387076, 1.000000000000000000, 0.8660254037844387076, 1.000000000000000000, 0.8660254037844387076, 1.000000000000000000, 0.8660254037844387076, 1.000000000000000000, 0.8660254037844387076, 1.000000000000000000, 0.8660254037844387076, 1.000000000000000000, 0.8660254037844387076, 1.000000000000000000, 0.8660254037844387076, 1.000000000000000000, 0.8660254037844387076, 1.000000000000000000, 0.8660254037844387076, 1.000000000000000000, 0.8660254037844387076, 1.000000000000000000, 0.8660254037844387076, 1.000000000000000000, 0.8660254037844387076, 1.000000000000000000, 0.8660254037844387076, 1.000000000000000000, 0.8660254037844387076, 1.000000000000000000, 0.8660254037844387076, 1.000000000000000000, 0.8660254037844387076, 1.000000000000000000, 0.8660254037844387076, 1.000000000000000000, 0.8660254037844387076, 1.000000000000000000, 0.8660254037844387076, 1.000000000000000000, 0.8660254037844387076, 1.000000000000000000, 0.8660254037844387076, 1.000000000000000000, 0.8660254037844387076, 1.000000000000000000, 0.8660254037844387076, 1.000000000000000000, 0.8660254037844387076, 1.000000000000000000, 0.8660254037844387076, 1.000000000000000000, 0.8660254037844387076, 1.000000000000000000, 0.8660254037844387076, 1.000000000000000000, 0.8660254037844387076, 1.000000000000000000, 0.8660254037844387076, 1.000000000000000000, 0.8660254037844387076, 1.000000000000000000, 0.8660254037844387076, 1.000000000000000000, 0.8660254037844387076, 1.000000000000000000, 0.8660254037844387076, 1.000000000000000000, 0.8660254037844387076, 1.000000000000000000, 0.8660254037844387076, 1.000000000000000000, 0.8660254037844387076, 1.000000000000000000, 0.8660254037844387076, 1.000000000000000000, 0.8660254037844387076, 1.000000000000000000, 0.8660254037844387076, 1.000000000000000000, 0.8660254037844387076, 1.000000000000000000, 0.8660254037844387076, 1.000000000000000000, 0.8660254037844387076, 1.000000000000000000, 0.8660254037844387076, 1.000000000000000000, 0.8660254037844387076, 1.000000000000000000, 0.8660254037844387076, 1.000000000000000000, 0.8660254037844387076, 1.000000000000000000, 0.8660254037844387076, 1.000000000000000000, 0.8660254037844387076, 1.000000000000000000, 0.8660254037844387076, 1.000000000000000000, 0.8660254037844387076, 1.000000000000000000, 0.8660254037844387076, 1.000000000000000000, 0.8660254037844387076, 1.000000000000000000, 0.8660254037844387076, 1.000000000000000000, 0.8660254037844387076, 1.000000000000000000, 0.8660254037844387076, 1.000000000000000000, 0.8660254037844387076, 1.000000000000000000, 0.8660254037844387076, 1.000000000000000000, 0.8660254037844387076, 1.000000000000000000, 0.8660254037844387076, 1.000000000000000000, 0.8660254037844387076, 1.000000000000000000, 0.8660254037844387076, 1.000000000000000000, 0.8660254037844387076, 1.000000000000000000, 0.8660254037844387076, 1.000000000000000000, 0.8660254037844387076, 1.000000000000000000, 0.8660254037844387076, 1.000000000000000000, 0.8660254037844387076, 1.000000000000000000, 0.8660254037844387076, 1.000000000000000000, 0.8660254037844387076, 1.000000000000000000, 0.8660254037844387076, 1.000000000000000000, 0.8660254037844387076, 1.000000000000000000, 0.8660254037844387076, 1.000000000000000000, 0.8660254037844387076, 1.000000000000000000, 0.8660254037844387076, 1.000000000000000000, 0.8660254037844387076, 1.000000000000000000, 0.8660254037844387076, 1.000000000000000000, 0.8660254037844387076, 1.000000000000000000, 0.8660254037844387076, 1.000000000000000000, 0.8660254037844387076, 1.000000000000000000, 0.8660254037844387076, 1.000000000000000000, 0.8660254037844387076, 1.000000000000000000, 0.8660254037844387076, 1.000000000000000000, 0.8660254037844387076, 1.000000000000000000, 0.8660254037844387076, 1.000000000000000000, 0.8660254037844387076, 1.000000000000000000, 0.8660254037844387076, 1.000000000000000000, 0.8660254037844387076, 1.000000000000000000, 0.8660254037844387076, 1.000000000000000000, 0.8660254037844387076, 1.000000000000000000, 0.8660254037844387076, 1.000000000000000000, 0.8660254037844387076, 1.000000000000000000, 0.8660254037844387076, 1.000000000000000000, 0.8660254037844387076, 1.000000000000000000, 0.8660254037844387076, 1.000000000000000000, 0.8660254037844387076, 1.000000000000000000, 0.8660254037844387076, 1.000000000000000000, 0.8660254037844387076, 1.000000000000000000, 0.8660254037844387076, 1.000000000000000000, 0.8660254037844387076, 1.000000000000000000, 0.8660254037844387076, 1.000000000000000000, 0.8660254037844387076, 1.000000000000000000, 0.8660254037844387076, 1.000000000000000000, 0.9548847324609573972, 0.9401541411607521326) ) ) 
 REPRESENTATION_ITEM ( '' )  SURFACE ( )  );
#28978=CARTESIAN_POINT ( 'NONE',  ( 20.99999999999999645, 243.1093750006145342, 6.646953231504538984 ) ) ;
#28984=CARTESIAN_POINT ( 'NONE',  ( -29.00000000000002487, 210.0000000000000000, 8.000000000000000000 ) ) ;
#28985=CARTESIAN_POINT ( 'NONE',  ( 15.00000000000000000, 241.0562500012290457, 0.000000000000000000 ) ) ;
#28988=CARTESIAN_POINT ( 'NONE',  ( 0.000000000000000000, 210.0000000000000284, -27.00000000000000000 ) ) ;
#28992=CARTESIAN_POINT ( 'NONE',  ( 18.12178482187500350, 242.1718750006145058, 4.985214923628407568 ) ) ;
#28993=ORIENTED_EDGE ( 'NONE', *, *, #14737, .T. ) ;
#28997=CARTESIAN_POINT ( 'NONE',  ( 0.000000000000000000, 210.0000000000000284, 0.000000000000000000 ) ) ;
#28998=CARTESIAN_POINT ( 'NONE',  ( 15.00000000000000000, 242.3687500012290741, -3.464101615137752610 ) ) ;
#29000=CARTESIAN_POINT ( 'NONE',  ( -13.49999999999998401, 197.0375000012290627, 23.38268590217985476 ) ) ;
#29005=CARTESIAN_POINT ( 'NONE',  ( 15.00000000000000000, 239.7062500012290513, 0.000000000000000000 ) ) ;
#29015=CARTESIAN_POINT ( 'NONE',  ( 20.99999999999999645, 249.6343750006145399, -6.646953231504538984 ) ) ;
#29016=CARTESIAN_POINT ( 'NONE',  ( -26.88106477066232713, 195.0000000000000568, 3.495181417218032660 ) ) ;
#29024=VECTOR ( 'NONE', #22632, 1000.000000000000000 ) ;
#29030=EDGE_CURVE ( 'NONE', #13411, #24114, #19685, .T. ) ;
#29033=CARTESIAN_POINT ( 'NONE',  ( 15.00000000000000178, 242.3875000000000171, 3.464101615137757051 ) ) ;
#29037=CARTESIAN_POINT ( 'NONE',  ( 13.50000000000001421, 197.4500000000000171, 23.38268590217984055 ) ) ;
#29039=CARTESIAN_POINT ( 'NONE',  ( 18.12178482187500350, 244.9843750006145342, 4.985214923628407568 ) ) ;
#29041=LINE ( 'NONE', #21111, #19093 ) ;
#29046=CARTESIAN_POINT ( 'NONE',  ( 18.00000000000000000, 246.3812500012290343, -5.196152422706630247 ) ) ;
#29053=ORIENTED_EDGE ( 'NONE', *, *, #8031, .F. ) ;
#29059=CARTESIAN_POINT ( 'NONE',  ( 23.87821517812500005, 245.8468750006145171, 4.985214923628404016 ) ) ;
#29062=CARTESIAN_POINT ( 'NONE',  ( 16.47967912936614709, 222.0541889883613749, -3.964960503604720632 ) ) ;
#29068=( BOUNDED_CURVE ( )  B_SPLINE_CURVE ( 2, ( #5635, #27836, #1867, #34081, #3358, #25924, #29319, #23836, #23277 ),
 .UNSPECIFIED., .F., .F. ) 
 B_SPLINE_CURVE_WITH_KNOTS ( ( 3, 2, 2, 2, 3 ),
 ( 0.2500000000000000000, 0.2536231884057971175, 0.2608695652173912971, 0.2681159420289855322, 0.2717391304347825942 ),
 .UNSPECIFIED. ) 
 CURVE ( )  GEOMETRIC_REPRESENTATION_ITEM ( )  RATIONAL_B_SPLINE_CURVE ( ( 0.9330127018922194093, 0.9330127018922190762, 1.000000000000000000, 0.8660254037844387076, 1.000000000000000000, 0.8660254037844387076, 1.000000000000000000, 0.9330127018922198534, 0.9330127018922191873 ) ) 
 REPRESENTATION_ITEM ( '' )  );
#29089=CARTESIAN_POINT ( 'NONE',  ( -27.00000000000000355, 195.4625000000000057, -15.58845726811989429 ) ) ;
#29092=CARTESIAN_POINT ( 'NONE',  ( 26.75643035624999655, 245.9968750006145513, 3.323476615752267271 ) ) ;
#29093=ORIENTED_EDGE ( 'NONE', *, *, #7630, .F. ) ;
#29095=CARTESIAN_POINT ( 'NONE',  ( 24.00000000000000000, 243.4000000000000057, 5.196152422706629359 ) ) ;
#29096=EDGE_CURVE ( 'NONE', #8916, #18637, #14387, .T. ) ;
#29100=CARTESIAN_POINT ( 'NONE',  ( 15.00000000000000178, 241.9375000000000000, 3.464101615137757051 ) ) ;
#29105=CARTESIAN_POINT ( 'NONE',  ( 20.99999999999995026, 240.9437500012290911, -5.999999999999998224 ) ) ;
#29106=CYLINDRICAL_SURFACE ( 'NONE', #30610, 5.999999999999999112 ) ;
#29110=CARTESIAN_POINT ( 'NONE',  ( 15.24356964374999990, 241.3093750006145228, 0.000000000000000000 ) ) ;
#29111=AXIS2_PLACEMENT_3D ( 'NONE', #12359, #20904, #24492 ) ;
#29119=DIRECTION ( 'NONE',  ( 0.000000000000000000, 0.000000000000000000, -1.000000000000000000 ) ) ;
#29120=CARTESIAN_POINT ( 'NONE',  ( 13.62178482187499640, 196.5593750006145513, -23.59362340125807123 ) ) ;
#29122=ADVANCED_FACE ( 'NONE', ( #6755 ), #18329, .F. ) ;
#29125=CARTESIAN_POINT ( 'NONE',  ( -4.632842373742755981, 226.1292383950976159, -2.500000000000000000 ) ) ;
#29129=( BOUNDED_CURVE ( )  B_SPLINE_CURVE ( 2, ( #7104, #18484, #21513, #7468, #33427, #30598, #9932, #4613, #27180 ),
 .UNSPECIFIED., .F., .T. ) 
 B_SPLINE_CURVE_WITH_KNOTS ( ( 3, 2, 2, 2, 3 ),
 ( 0.02083333333333333565, 0.02777777777777777624, 0.04166666666666666435, 0.05555555555555555247, 0.06250000000000000000 ),
 .UNSPECIFIED. ) 
 CURVE ( )  GEOMETRIC_REPRESENTATION_ITEM ( )  RATIONAL_B_SPLINE_CURVE ( ( 0.9330127018922194093, 0.9330127018922194093, 1.000000000000000000, 0.8660254037844387076, 1.000000000000000000, 0.8660254037844387076, 1.000000000000000000, 0.9330127018922194093, 0.9330127018922194093 ) ) 
 REPRESENTATION_ITEM ( '' )  );
#29134=DIRECTION ( 'NONE',  ( 0.000000000000000000, 0.000000000000000000, 1.000000000000000000 ) ) ;
#29138=DIRECTION ( 'NONE',  ( 0.000000000000000000, 0.000000000000000000, -1.000000000000000000 ) ) ;
#29139=ORIENTED_EDGE ( 'NONE', *, *, #8349, .F. ) ;
#29144=CARTESIAN_POINT ( 'NONE',  ( -27.00000000000000355, 198.1625000000000227, -15.58845726811989429 ) ) ;
#29145=CARTESIAN_POINT ( 'NONE',  ( 26.99999999999999645, 248.4624999999999773, -3.464101615137755275 ) ) ;
#29146=CARTESIAN_POINT ( 'NONE',  ( 27.24356964375000700, 198.6406250006145342, 15.72908226750537075 ) ) ;
#29151=CARTESIAN_POINT ( 'NONE',  ( 27.24356964375000345, 199.1281250006145171, -3.336375036156643733E-15 ) ) ;
#29152=CARTESIAN_POINT ( 'NONE',  ( 26.75643035624999655, 242.8093750006144944, -3.323476615752271712 ) ) ;
#29155=CARTESIAN_POINT ( 'NONE',  ( 26.75643035624999655, 246.4468750006144830, 3.323476615752267715 ) ) ;
#29156=AXIS2_PLACEMENT_3D ( 'NONE', #12881, #9479, #18393 ) ;
#29161=CARTESIAN_POINT ( 'NONE',  ( 26.75643035624999655, 242.3218750006145399, -7.049594010296217766E-16 ) ) ;
#29170=CARTESIAN_POINT ( 'NONE',  ( 15.00000000000000178, 241.0937500012290400, 3.464101615137757051 ) ) ;
#29180=CARTESIAN_POINT ( 'NONE',  ( 18.12178482187499640, 241.5718750006145399, -4.985214923628404904 ) ) ;
#29185=CARTESIAN_POINT ( 'NONE',  ( 20.99999999999999289, 241.7874999999999659, -5.999999999999997335 ) ) ;
#29186=CARTESIAN_POINT ( 'NONE',  ( 20.99999999999995026, 243.1375000000000455, -5.999999999999998224 ) ) ;
#29187=CARTESIAN_POINT ( 'NONE',  ( 5.778771075727756162E-15, 195.4718750006145456, 31.45816453501075927 ) ) ;
#29188=CARTESIAN_POINT ( 'NONE',  ( -6.245661213598732608, 195.0000000000000853, 26.53257588854514637 ) ) ;
#29189=CARTESIAN_POINT ( 'NONE',  ( -4.694659320240884604E-14, 197.0750000012290570, 27.00000000000000000 ) ) ;
#29193=ORIENTED_EDGE ( 'NONE', *, *, #5043, .F. ) ;
#29194=CARTESIAN_POINT ( 'NONE',  ( 18.00000000000000355, 239.7812500012290400, 5.196152422706632912 ) ) ;
#29200=CARTESIAN_POINT ( 'NONE',  ( 21.00000000000000000, 247.8624999999999545, 5.999999999999998224 ) ) ;
#29201=ORIENTED_EDGE ( 'NONE', *, *, #1909, .F. ) ;
#29207=CARTESIAN_POINT ( 'NONE',  ( 26.75643035624999655, 248.6218750006145228, -7.049594010296217766E-16 ) ) ;
#29214=CARTESIAN_POINT ( 'NONE',  ( 22.60769515458672885, 241.6388461906613259, 5.999999999999997335 ) ) ;
#29227=CARTESIAN_POINT ( 'NONE',  ( 26.99999999999999645, 195.8750000012290400, -15.58845726811990495 ) ) ;
#29229=CARTESIAN_POINT ( 'NONE',  ( 20.99999999999999645, 192.3000000000000398, 8.000000000000000000 ) ) ;
#29232=CARTESIAN_POINT ( 'NONE',  ( 15.24356964374999990, 244.8718750006145513, -3.323476615752268604 ) ) ;
#29237=CARTESIAN_POINT ( 'NONE',  ( 26.99999999999999645, 246.2687500012290513, -3.464101615137755275 ) ) ;
#29246=EDGE_LOOP ( 'NONE', ( #29957, #23925, #23206, #29584, #24758, #3944, #14902, #35657 ) ) ;
#29249=CARTESIAN_POINT ( 'NONE',  ( 15.24356964374999990, 246.5593750006144944, -3.323476615752268604 ) ) ;
#29261=CARTESIAN_POINT ( 'NONE',  ( -27.24356964375001056, 194.8294844423495533, -9.915847621322177119 ) ) ;
#29278=CARTESIAN_POINT ( 'NONE',  ( 27.00000000000001066, 196.1375000000000171, 15.58845726811988897 ) ) ;
#29281=CARTESIAN_POINT ( 'NONE',  ( 15.24356964374999990, 245.7718750006145001, -3.323476615752268604 ) ) ;
#29289=CARTESIAN_POINT ( 'NONE',  ( 18.91622499444735084, 240.0135471875693725, -5.725135169889072451 ) ) ;
#29293=ORIENTED_EDGE ( 'NONE', *, *, #10802, .T. ) ;
#29297=CARTESIAN_POINT ( 'NONE',  ( 26.99999999999999645, 195.3125000000000000, -15.58845726811990495 ) ) ;
#29302=CARTESIAN_POINT ( 'NONE',  ( 18.12178482187500350, 240.0343750006145171, 4.985214923628407568 ) ) ;
#29304=LINE ( 'NONE', #14912, #36128 ) ;
#29312=CARTESIAN_POINT ( 'NONE',  ( -27.24356964375000345, 195.3593750006145342, 0.000000000000000000 ) ) ;
#29318=CARTESIAN_POINT ( 'NONE',  ( -5.327872176777560753, 223.7027713702217113, -2.499999999999999112 ) ) ;
#29319=CARTESIAN_POINT ( 'NONE',  ( 18.00000000000000000, 247.2249999999999943, -5.196152422706630247 ) ) ;
#29328=EDGE_CURVE ( 'NONE', #25480, #24534, #14075, .T. ) ;
#29331=CARTESIAN_POINT ( 'NONE',  ( -27.00000000000000355, 195.1625000012290343, 0.000000000000000000 ) ) ;
#29333=CARTESIAN_POINT ( 'NONE',  ( 22.60769515458672529, 244.9736538117967370, -6.000000000000004441 ) ) ;
#29339=CARTESIAN_POINT ( 'NONE',  ( 15.00000000000000178, 249.1374999999999886, 3.464101615137757051 ) ) ;
#29340=CARTESIAN_POINT ( 'NONE',  ( 27.24356964375000700, 196.8406250006145228, 15.72908226750537075 ) ) ;
#29344=ORIENTED_EDGE ( 'NONE', *, *, #8449, .T. ) ;
#29345=CARTESIAN_POINT ( 'NONE',  ( 5.778771075727756162E-15, 194.9656250006145228, 31.45816453501075927 ) ) ;
#29346=CARTESIAN_POINT ( 'NONE',  ( 23.87821517812500005, 240.4468750006145115, 4.985214923628404016 ) ) ;
#29350=CARTESIAN_POINT ( 'NONE',  ( 23.87821517812500005, 248.6593750006145171, 4.985214923628404016 ) ) ;
#29355=CARTESIAN_POINT ( 'NONE',  ( 18.12178482187500350, 241.7218750006145171, 4.985214923628407568 ) ) ;
#29367=CARTESIAN_POINT ( 'NONE',  ( 13.50000000000001421, 198.3499999999999943, 23.38268590217984055 ) ) ;
#29369=CARTESIAN_POINT ( 'NONE',  ( 7.234628195640318005, 199.0799038117967541, -26.99999999999999645 ) ) ;
#29373=CARTESIAN_POINT ( 'NONE',  ( 15.24356964375000167, 242.1343750006145399, 3.323476615752272600 ) ) ;
#29374=ORIENTED_EDGE ( 'NONE', *, *, #36354, .T. ) ;
#29377=CYLINDRICAL_SURFACE ( 'NONE', #34395, 27.00000000000000000 ) ;
#29386=ORIENTED_EDGE ( 'NONE', *, *, #17949, .T. ) ;
#29387=CARTESIAN_POINT ( 'NONE',  ( 15.24356964374999990, 249.7468750006145228, 0.000000000000000000 ) ) ;
#29392=ADVANCED_FACE ( 'NONE', ( #14262 ), #25261, .F. ) ;
#29393=DIRECTION ( 'NONE',  ( 0.000000000000000000, 0.000000000000000000, 1.000000000000000000 ) ) ;
#29394=ORIENTED_EDGE ( 'NONE', *, *, #34206, .T. ) ;
#29397=ORIENTED_EDGE ( 'NONE', *, *, #25579, .T. ) ;
#29400=AXIS2_PLACEMENT_3D ( 'NONE', #24274, #27111, #26348 ) ;
#29403=CARTESIAN_POINT ( 'NONE',  ( 18.12178482187500350, 248.9218750006145342, 4.985214923628407568 ) ) ;
#29411=CARTESIAN_POINT ( 'NONE',  ( -27.90475745684348752, 208.6802886524470750, 7.894770873222196172 ) ) ;
#29423=LINE ( 'NONE', #17879, #6536 ) ;
#29427=CARTESIAN_POINT ( 'NONE',  ( 23.87821517812499650, 243.8593750006145342, -4.985214923628404904 ) ) ;
#29432=CARTESIAN_POINT ( 'NONE',  ( 18.00000000000000355, 246.9812500012290570, 5.196152422706632912 ) ) ;
#29440=EDGE_LOOP ( 'NONE', ( #14667, #29474, #37286, #13230 ) ) ;
#29443=CARTESIAN_POINT ( 'NONE',  ( 21.00000000000000000, 246.4843750006145058, -6.646953231504538984 ) ) ;
#29447=CARTESIAN_POINT ( 'NONE',  ( 15.80103094669413366, 223.8639174754800365, -3.001545256183639321 ) ) ;
#29469=CARTESIAN_POINT ( 'NONE',  ( 22.60769515458671108, 241.1888461906613657, 6.000000000000010658 ) ) ;
#29473=CARTESIAN_POINT ( 'NONE',  ( 15.24356964374999990, 245.8093750006145228, 0.000000000000000000 ) ) ;
#29474=ORIENTED_EDGE ( 'NONE', *, *, #8947, .T. ) ;
#29476=CARTESIAN_POINT ( 'NONE',  ( 15.00000000000000000, 245.0687500012290343, -3.464101615137752610 ) ) ;
#29477=CARTESIAN_POINT ( 'NONE',  ( 10.49999999999999822, 210.0000000000000284, -2.500000000000000000 ) ) ;
#29480=CARTESIAN_POINT ( 'NONE',  ( 18.00000000000000000, 240.4749999999999943, -5.196152422706630247 ) ) ;
#29481=CARTESIAN_POINT ( 'NONE',  ( 20.99999999999999645, 185.0294372515228645, 5.999999999999999112 ) ) ;
#29487=CARTESIAN_POINT ( 'NONE',  ( 15.00000000000000000, 243.6999999999999886, 0.000000000000000000 ) ) ;
#29488=CARTESIAN_POINT ( 'NONE',  ( 20.99999999999997513, 246.7375000000000114, -5.999999999999999112 ) ) ;
#29489=CARTESIAN_POINT ( 'NONE',  ( 20.99999999999998579, 248.0875000000000057, -5.999999999999997335 ) ) ;
#29494=CARTESIAN_POINT ( 'NONE',  ( 15.24356964374999990, 239.9218750006145626, -3.323476615752268604 ) ) ;
#29502=CARTESIAN_POINT ( 'NONE',  ( 18.00000000000000000, 240.9250000000000114, -5.196152422706630247 ) ) ;
#29503=CARTESIAN_POINT ( 'NONE',  ( -27.24356964375000345, 197.1593750006145456, 0.000000000000000000 ) ) ;
#29508=CARTESIAN_POINT ( 'NONE',  ( 26.99999999999999645, 245.3312500012290513, -7.347880794884117764E-16 ) ) ;
#29510=CARTESIAN_POINT ( 'NONE',  ( 13.50000000000001421, 198.8000000000000114, 23.38268590217984055 ) ) ;
#29517=CARTESIAN_POINT ( 'NONE',  ( 26.99999999999999645, 244.8625000000000114, -3.464101615137755275 ) ) ;
#29518=EDGE_CURVE ( 'NONE', #32797, #36568, #35266, .T. ) ;
#29525=AXIS2_PLACEMENT_3D ( 'NONE', #4662, #16245, #37422 ) ;
#29530=CARTESIAN_POINT ( 'NONE',  ( 18.00000000000000355, 248.2750000000000057, 5.196152422706632912 ) ) ;
#29531=CARTESIAN_POINT ( 'NONE',  ( 27.24356964374999279, 196.0156250006145342, -15.72908226750539207 ) ) ;
#29534=VECTOR ( 'NONE', #14612, 1000.000000000000000 ) ;
#29535=ORIENTED_EDGE ( 'NONE', *, *, #425, .T. ) ;
#29536=CARTESIAN_POINT ( 'NONE',  ( -1.926257025242585782E-15, 195.6406250006145058, -31.45816453501075927 ) ) ;
#29537=CARTESIAN_POINT ( 'NONE',  ( 23.87821517812499650, 240.1468750006145285, -4.985214923628404904 ) ) ;
#29538=EDGE_CURVE ( 'NONE', #12071, #7872, #30114, .T. ) ;
#29541=CARTESIAN_POINT ( 'NONE',  ( 26.75643035624999655, 248.2843750006145456, -7.049594010296217766E-16 ) ) ;
#29548=CARTESIAN_POINT ( 'NONE',  ( 18.12178482187499640, 242.0218750006145001, -4.985214923628404904 ) ) ;
#29560=EDGE_CURVE ( 'NONE', #6368, #11787, #32306, .T. ) ;
#29563=CARTESIAN_POINT ( 'NONE',  ( 2.999999999999997335, 252.0000000000000000, 2.500000000000000000 ) ) ;
#29566=CARTESIAN_POINT ( 'NONE',  ( 26.75643035624999655, 241.3843750006145399, 3.323476615752267715 ) ) ;
#29579=CARTESIAN_POINT ( 'NONE',  ( 21.00000000000000000, 247.3843750006145399, -6.646953231504538984 ) ) ;
#29584=ORIENTED_EDGE ( 'NONE', *, *, #26971, .F. ) ;
#29589=ADVANCED_FACE ( 'NONE', ( #24061 ), #12680, .T. ) ;
#29591=CARTESIAN_POINT ( 'NONE',  ( 18.12178482187499640, 249.2218750006145171, -4.985214923628404904 ) ) ;
#29593=CARTESIAN_POINT ( 'NONE',  ( 0.000000000000000000, 195.0000000000000000, -27.00000000000000000 ) ) ;
#29597=EDGE_LOOP ( 'NONE', ( #30845, #6930, #37021, #6201 ) ) ;
#29598=CARTESIAN_POINT ( 'NONE',  ( -27.87851222004085017, 209.4701072313699797, 7.986820506746719950 ) ) ;
#29602=EDGE_CURVE ( 'NONE', #12569, #190, #5185, .T. ) ;
#29608=CARTESIAN_POINT ( 'NONE',  ( -27.87471972953270338, 210.0000000000000284, -8.000000000000000000 ) ) ;
#29620=CARTESIAN_POINT ( 'NONE',  ( 26.99999999999999645, 243.0812500012290513, -7.347880794884117764E-16 ) ) ;
#29623=DIRECTION ( 'NONE',  ( -0.000000000000000000, 1.000000000000000000, -0.000000000000000000 ) ) ;
#29627=ORIENTED_EDGE ( 'NONE', *, *, #13611, .F. ) ;
#29631=CARTESIAN_POINT ( 'NONE',  ( 21.00000000000000000, 246.2593750006145115, 6.646953231504538984 ) ) ;
#29633=( BOUNDED_CURVE ( )  B_SPLINE_CURVE ( 2, ( #16036, #27023, #29862, #20980, #18320, #7131, #1233, #33088, #3898 ),
 .UNSPECIFIED., .F., .F. ) 
 B_SPLINE_CURVE_WITH_KNOTS ( ( 3, 2, 2, 2, 3 ),
 ( 0.7291666666666667407, 0.7361111111111111605, 0.7500000000000000000, 0.7638888888888888395, 0.7708333333333333703 ),
 .UNSPECIFIED. ) 
 CURVE ( )  GEOMETRIC_REPRESENTATION_ITEM ( )  RATIONAL_B_SPLINE_CURVE ( ( 0.9330127018922192983, 0.9330127018922198534, 1.000000000000000000, 0.8660254037844387076, 1.000000000000000000, 0.8660254037844387076, 1.000000000000000000, 0.9330127018922187432, 0.9330127018922192983 ) ) 
 REPRESENTATION_ITEM ( '' )  );
#29648=ADVANCED_FACE ( 'NONE', ( #33151 ), #10067, .T. ) ;
#29657=CARTESIAN_POINT ( 'NONE',  ( 27.00000000000000355, 195.7250000000000227, -3.306546357697854128E-15 ) ) ;
#29659=CARTESIAN_POINT ( 'NONE',  ( 18.12178482187500350, 249.4843750006145342, 4.985214923628407568 ) ) ;
#29661=CARTESIAN_POINT ( 'NONE',  ( 26.75643035624999655, 245.5468750006145342, 3.323476615752267271 ) ) ;
#29663=VERTEX_POINT ( 'NONE', #8625 ) ;
#29670=CARTESIAN_POINT ( 'NONE',  ( -13.66537537263149282, 216.1427711317592752, 5.155187915310053270 ) ) ;
#29673=ORIENTED_EDGE ( 'NONE', *, *, #10728, .T. ) ;
#29674=CARTESIAN_POINT ( 'NONE',  ( 20.99999999999997868, 204.0000000000000000, 0.000000000000000000 ) ) ;
#29684=CARTESIAN_POINT ( 'NONE',  ( -4.605287895664654130, 226.1383394588005444, 2.499999999999999556 ) ) ;
#29691=CARTESIAN_POINT ( 'NONE',  ( 27.24356964375000700, 199.0906250006145228, 15.72908226750537075 ) ) ;
#29694=VERTEX_POINT ( 'NONE', #19835 ) ;
#29696=CARTESIAN_POINT ( 'NONE',  ( -4.712253383274792817, 225.7113004343964349, -2.500000000000000000 ) ) ;
#29707=CARTESIAN_POINT ( 'NONE',  ( 26.99999999999999645, 247.5437500012290570, 3.464101615137751278 ) ) ;
#29711=CARTESIAN_POINT ( 'NONE',  ( -27.00000000000000355, 195.6125000012290513, 0.000000000000000000 ) ) ;
#29715=FACE_OUTER_BOUND ( 'NONE', #24280, .T. ) ;
#29716=CARTESIAN_POINT ( 'NONE',  ( 15.00000000000000178, 247.7874999999999943, 3.464101615137757051 ) ) ;
#29717=CARTESIAN_POINT ( 'NONE',  ( 5.778771075727756162E-15, 195.8656250006145285, 31.45816453501076637 ) ) ;
#29722=CARTESIAN_POINT ( 'NONE',  ( -13.62178482187498396, 195.8281250006145342, 23.59362340125808188 ) ) ;
#29723=CARTESIAN_POINT ( 'NONE',  ( 21.00000000000000000, 240.6343750006145115, -6.646953231504538984 ) ) ;
#29727=CARTESIAN_POINT ( 'NONE',  ( 15.24356964375000167, 248.5468750006145342, 3.323476615752272600 ) ) ;
#29733=CARTESIAN_POINT ( 'NONE',  ( 26.75643035624999655, 240.4843750006145058, 3.323476615752267271 ) ) ;
#29735=DIRECTION ( 'NONE',  ( 0.000000000000000000, 0.000000000000000000, -1.000000000000000000 ) ) ;
#29740=DIRECTION ( 'NONE',  ( 0.000000000000000000, 0.000000000000000000, -1.000000000000000000 ) ) ;
#29746=CARTESIAN_POINT ( 'NONE',  ( 7.234628195640322446, 198.3325961894323370, 26.99999999999999645 ) ) ;
#29752=CARTESIAN_POINT ( 'NONE',  ( 15.24356964374999990, 242.5093750006144830, -3.323476615752268604 ) ) ;
#29756=CARTESIAN_POINT ( 'NONE',  ( 27.24356964375000345, 199.6343750006145399, -3.336375036156643733E-15 ) ) ;
#29758=CARTESIAN_POINT ( 'NONE',  ( 0.000000000000000000, 210.0000000000000284, -27.00000000000000000 ) ) ;
#29759=LINE ( 'NONE', #3789, #37386 ) ;
#29765=CARTESIAN_POINT ( 'NONE',  ( 15.24356964375000167, 246.6343750006145115, 3.323476615752272600 ) ) ;
#29771=ORIENTED_EDGE ( 'NONE', *, *, #21970, .F. ) ;
#29774=VERTEX_POINT ( 'NONE', #17166 ) ;
#29780=CARTESIAN_POINT ( 'NONE',  ( 20.99999999999999645, 246.0343750006144887, -6.646953231504538984 ) ) ;
#29787=CARTESIAN_POINT ( 'NONE',  ( 22.60769515458672885, 241.8236538117967029, -5.999999999999998224 ) ) ;
#29790=EDGE_CURVE ( 'NONE', #8565, #15992, #11351, .T. ) ;
#29808=CARTESIAN_POINT ( 'NONE',  ( 26.99999999999999645, 243.0437500012290570, 3.464101615137751278 ) ) ;
#29811=CARTESIAN_POINT ( 'NONE',  ( -27.24356964374999635, 199.3906250006145342, 15.72908226750539384 ) ) ;
#29817=CARTESIAN_POINT ( 'NONE',  ( 26.75643035624999655, 243.6343750006145115, 3.323476615752267715 ) ) ;
#29837=LINE ( 'NONE', #15446, #35517 ) ;
#29843=CARTESIAN_POINT ( 'NONE',  ( 1.069080835302379631E-14, 195.6124999999999829, 27.00000000000000000 ) ) ;
#29845=CARTESIAN_POINT ( 'NONE',  ( 21.00000000000000000, 249.7468750006145797, -6.646953231504538984 ) ) ;
#29847=CARTESIAN_POINT ( 'NONE',  ( 15.24356964375000167, 246.2968750006145626, 3.323476615752272600 ) ) ;
#29850=CARTESIAN_POINT ( 'NONE',  ( -1.045839947578415010E-13, 196.0625000000000284, 27.00000000000000355 ) ) ;
#29858=LINE ( 'NONE', #29481, #17267 ) ;
#29860=EDGE_LOOP ( 'NONE', ( #28862, #18741, #20786, #17417, #272 ) ) ;
#29862=CARTESIAN_POINT ( 'NONE',  ( -13.49999999999998401, 196.0250000000000057, 23.38268590217985476 ) ) ;
#29865=( GEOMETRIC_REPRESENTATION_CONTEXT ( 3 ) GLOBAL_UNCERTAINTY_ASSIGNED_CONTEXT ( ( #7068 ) ) GLOBAL_UNIT_ASSIGNED_CONTEXT ( ( #1195, #15617, #32291 ) ) REPRESENTATION_CONTEXT ( 'NONE', 'WORKASPACE' ) );
#29883=CARTESIAN_POINT ( 'NONE',  ( -13.62178482187498396, 198.5281250006145228, 23.59362340125808188 ) ) ;
#29886=VERTEX_POINT ( 'NONE', #1393 ) ;
#29891=AXIS2_PLACEMENT_3D ( 'NONE', #367, #34677, #32020 ) ;
#29896=LINE ( 'NONE', #35761, #1307 ) ;
#29902=CARTESIAN_POINT ( 'NONE',  ( 26.99999999999999645, 199.3625000000000114, -15.58845726811990495 ) ) ;
#29904=DIRECTION ( 'NONE',  ( 0.000000000000000000, 0.000000000000000000, 1.000000000000000000 ) ) ;
#29907=CARTESIAN_POINT ( 'NONE',  ( 20.99999999999999645, 185.0294372515228645, -5.999999999999999112 ) ) ;
#29910=CARTESIAN_POINT ( 'NONE',  ( 26.99999999999999645, 245.2375000000000114, 3.464101615137751278 ) ) ;
#29911=CARTESIAN_POINT ( 'NONE',  ( -13.62178482187500528, 196.1281250006145171, -23.59362340125807123 ) ) ;
#29914=ORIENTED_EDGE ( 'NONE', *, *, #33945, .F. ) ;
#29915=ORIENTED_EDGE ( 'NONE', *, *, #9631, .F. ) ;
#29916=CARTESIAN_POINT ( 'NONE',  ( -13.62178482187500528, 196.5781250006145342, -23.59362340125807123 ) ) ;
#29919=CARTESIAN_POINT ( 'NONE',  ( 26.75643035624999655, 245.5468750006145342, 3.323476615752267715 ) ) ;
#29930=CARTESIAN_POINT ( 'NONE',  ( 27.00000000000001421, 197.9375000000000284, 15.58845726811988897 ) ) ;
#29939=CARTESIAN_POINT ( 'NONE',  ( 1.120210788295102201E-13, 196.4000000012290741, -27.00000000000000711 ) ) ;
#29940=CARTESIAN_POINT ( 'NONE',  ( 20.99999999999998579, 248.0875000000000057, -5.999999999999997335 ) ) ;
#29941=CARTESIAN_POINT ( 'NONE',  ( 7.234628195640337545, 198.5174038105677141, -26.99999999999999289 ) ) ;
#29943=CARTESIAN_POINT ( 'NONE',  ( 21.00000000000000000, 248.3687500012290741, 5.999999999999998224 ) ) ;
#29946=CARTESIAN_POINT ( 'NONE',  ( 21.00000000000000000, 240.1843750006145513, -6.646953231504538984 ) ) ;
#29952=DIRECTION ( 'NONE',  ( 0.000000000000000000, 0.000000000000000000, 1.000000000000000000 ) ) ;
#29957=ORIENTED_EDGE ( 'NONE', *, *, #32309, .T. ) ;
#29959=CARTESIAN_POINT ( 'NONE',  ( 23.87821517812500005, 245.8468750006145171, 4.985214923628404016 ) ) ;
#29971=CARTESIAN_POINT ( 'NONE',  ( 26.75643035624999655, 246.4093750006144887, -3.323476615752271268 ) ) ;
#29977=VECTOR ( 'NONE', #12884, 1000.000000000000000 ) ;
#29978=CARTESIAN_POINT ( 'NONE',  ( -28.29648172771258885, 205.1140383288905298, 6.355902910654599225 ) ) ;
#29994=CARTESIAN_POINT ( 'NONE',  ( 27.00000000000001066, 195.2375000000000114, 15.58845726811988897 ) ) ;
#30000=EDGE_LOOP ( 'NONE', ( #13841, #36338, #11901, #33272 ) ) ;
#30002=CARTESIAN_POINT ( 'NONE',  ( 26.99999999999999645, 244.0187500012290513, -3.464101615137755275 ) ) ;
#30010=CARTESIAN_POINT ( 'NONE',  ( 18.12178482187499640, 244.7218750006145171, -4.985214923628404904 ) ) ;
#30033=CARTESIAN_POINT ( 'NONE',  ( 20.99999999999999645, 185.0294372515228645, 0.000000000000000000 ) ) ;
#30037=CARTESIAN_POINT ( 'NONE',  ( 23.87821517812499650, 249.7093750006145285, -4.985214923628404904 ) ) ;
#30039=CARTESIAN_POINT ( 'NONE',  ( 26.75643035624999655, 245.1718750006145058, -3.323476615752271268 ) ) ;
#30040=ORIENTED_EDGE ( 'NONE', *, *, #7960, .T. ) ;
#30042=CARTESIAN_POINT ( 'NONE',  ( 19.39230484541324628, 245.0138461906613543, -5.999999999999989342 ) ) ;
#30049=EDGE_LOOP ( 'NONE', ( #14248, #35646, #35059, #26407 ) ) ;
#30056=CARTESIAN_POINT ( 'NONE',  ( 22.60769515458671108, 242.9325961894323029, 6.000000000000010658 ) ) ;
#30070=CARTESIAN_POINT ( 'NONE',  ( 27.24356964375000345, 197.7781250006145228, -3.336375036156643733E-15 ) ) ;
#30087=ADVANCED_FACE ( 'NONE', ( #12588 ), #4051, .F. ) ;
#30088=DIRECTION ( 'NONE',  ( 0.000000000000000000, 0.000000000000000000, -1.000000000000000000 ) ) ;
#30091=CARTESIAN_POINT ( 'NONE',  ( 26.99999999999999645, 247.5812500012290513, -7.347880794884117764E-16 ) ) ;
#30101=CARTESIAN_POINT ( 'NONE',  ( 26.99999999999999645, 246.6250000000000000, -7.347880794884117764E-16 ) ) ;
#30102=CARTESIAN_POINT ( 'NONE',  ( -27.24356964375000345, 195.2656250006145342, -15.72908226750537786 ) ) ;
#30108=CARTESIAN_POINT ( 'NONE',  ( -13.62178482187500528, 196.1281250006145171, -23.59362340125807123 ) ) ;
#30113=CARTESIAN_POINT ( 'NONE',  ( 18.12178482187500350, 244.9843750006145342, 4.985214923628407568 ) ) ;
#30114=( BOUNDED_CURVE ( )  B_SPLINE_CURVE ( 2, ( #35461, #9322, #778, #5902, #35083, #32058, #9135, #14822, #401 ),
 .UNSPECIFIED., .F., .F. ) 
 B_SPLINE_CURVE_WITH_KNOTS ( ( 3, 2, 2, 2, 3 ),
 ( 0.3804347826086956763, 0.3840579710144927383, 0.3913043478260869734, 0.3985507246376811530, 0.4021739130434782705 ),
 .UNSPECIFIED. ) 
 CURVE ( )  GEOMETRIC_REPRESENTATION_ITEM ( )  RATIONAL_B_SPLINE_CURVE ( ( 0.9330127018922194093, 0.9330127018922198534, 1.000000000000000000, 0.8660254037844387076, 1.000000000000000000, 0.8660254037844387076, 1.000000000000000000, 0.9330127018922194093, 0.9330127018922194093 ) ) 
 REPRESENTATION_ITEM ( '' )  );
#30120=CARTESIAN_POINT ( 'NONE',  ( 20.99999999999999645, 240.4093750006145171, 6.646953231504538984 ) ) ;
#30129=CARTESIAN_POINT ( 'NONE',  ( 15.00000000000000000, 244.1500000000000057, 0.000000000000000000 ) ) ;
#30135=CARTESIAN_POINT ( 'NONE',  ( 15.24356964374999990, 248.9593750006145285, 0.000000000000000000 ) ) ;
#30136=ORIENTED_EDGE ( 'NONE', *, *, #17571, .T. ) ;
#30140=CARTESIAN_POINT ( 'NONE',  ( -13.62178482187500528, 199.3343750006145569, -23.59362340125807123 ) ) ;
#30144=CARTESIAN_POINT ( 'NONE',  ( 23.87821517812499650, 242.0593750006145228, -4.985214923628404904 ) ) ;
#30151=CARTESIAN_POINT ( 'NONE',  ( 26.75643035624999655, 246.3718750006145228, -7.049594010296217766E-16 ) ) ;
#30163=CARTESIAN_POINT ( 'NONE',  ( 20.99999999999999645, 246.9343750006145228, -6.646953231504538984 ) ) ;
#30174=CARTESIAN_POINT ( 'NONE',  ( 19.39230484541326405, 249.0638461906613657, -5.999999999999998224 ) ) ;
#30180=CARTESIAN_POINT ( 'NONE',  ( -1.045839947578415010E-13, 196.1750000012290229, 27.00000000000000355 ) ) ;
#30186=CARTESIAN_POINT ( 'NONE',  ( -13.50000000000000533, 195.4250000000000114, -23.38268590217984411 ) ) ;
#30190=VERTEX_POINT ( 'NONE', #24344 ) ;
#30191=CARTESIAN_POINT ( 'NONE',  ( 15.00000000000000178, 243.3437500012290400, 3.464101615137757051 ) ) ;
#30198=CARTESIAN_POINT ( 'NONE',  ( 20.99999999999999645, 185.0294372515228645, 5.999999999999999112 ) ) ;
#30199=CARTESIAN_POINT ( 'NONE',  ( 15.24356964374999990, 243.8968750006145285, 0.000000000000000000 ) ) ;
#30205=CYLINDRICAL_SURFACE ( 'NONE', #3647, 5.999999999999999112 ) ;
#30210=( BOUNDED_CURVE ( )  B_SPLINE_CURVE ( 3, ( #3419, #21439, #14987, #7033 ),
 .UNSPECIFIED., .F., .F. ) 
 B_SPLINE_CURVE_WITH_KNOTS ( ( 4, 4 ),
 ( 4.712388980384690562, 6.283185307179586232 ),
 .UNSPECIFIED. ) 
 CURVE ( )  GEOMETRIC_REPRESENTATION_ITEM ( )  RATIONAL_B_SPLINE_CURVE ( ( 1.000000000000000000, 0.8047378541243652705, 0.8047378541243652705, 1.000000000000000000 ) ) 
 REPRESENTATION_ITEM ( '' )  );
#30215=FACE_OUTER_BOUND ( 'NONE', #26880, .T. ) ;
#30220=CARTESIAN_POINT ( 'NONE',  ( -27.93311285808765732, 208.1767028850233885, -7.793846208402254838 ) ) ;
#30230=CARTESIAN_POINT ( 'NONE',  ( 9.000000000000003553, 242.0000000000000000, -5.999999999999998224 ) ) ;
#30232=CARTESIAN_POINT ( 'NONE',  ( 23.87821517812499650, 243.4093750006145171, -4.985214923628404904 ) ) ;
#30234=CARTESIAN_POINT ( 'NONE',  ( 15.00000000000000178, 245.1437500012290798, 3.464101615137757051 ) ) ;
#30246=CARTESIAN_POINT ( 'NONE',  ( 26.99999999999999645, 249.3812500012290343, -7.347880794884117764E-16 ) ) ;
#30247=DIRECTION ( 'NONE',  ( -0.000000000000000000, 1.000000000000000000, -0.000000000000000000 ) ) ;
#30251=CARTESIAN_POINT ( 'NONE',  ( 22.60769515458672885, 243.6236538117967143, -5.999999999999998224 ) ) ;
#30252=CARTESIAN_POINT ( 'NONE',  ( 18.34109276192021909, 217.0904193015437613, 5.392997762649728521 ) ) ;
#30260=EDGE_CURVE ( 'NONE', #36155, #5728, #7026, .T. ) ;
#30263=CARTESIAN_POINT ( 'NONE',  ( -1.926257025242585782E-15, 199.2406250006145285, -31.45816453501075927 ) ) ;
#30269=CARTESIAN_POINT ( 'NONE',  ( -27.00000000000000355, 197.7500000000000000, 0.000000000000000000 ) ) ;
#30279=CARTESIAN_POINT ( 'NONE',  ( -1.909035429704832693E-15, 199.4375000000000284, -31.17691453623979214 ) ) ;
#30284=EDGE_LOOP ( 'NONE', ( #37239, #30927, #36591, #24473, #14939, #27207 ) ) ;
#30286=VECTOR ( 'NONE', #17654, 1000.000000000000000 ) ;
#30290=CARTESIAN_POINT ( 'NONE',  ( 23.99999999999999645, 246.6999999999999886, -5.196152422706631135 ) ) ;
#30294=EDGE_LOOP ( 'NONE', ( #24734, #23406, #13748, #36287 ) ) ;
#30296=CARTESIAN_POINT ( 'NONE',  ( -27.00000000000000355, 199.2125000012290457, 0.000000000000000000 ) ) ;
#30297=CARTESIAN_POINT ( 'NONE',  ( 1.120210788295102201E-13, 196.7375000000000398, -27.00000000000000711 ) ) ;
#30300=CARTESIAN_POINT ( 'NONE',  ( 23.87821517812499650, 245.2093750006145569, -4.985214923628404904 ) ) ;
#30301=AXIS2_PLACEMENT_3D ( 'NONE', #33771, #24864, #5137 ) ;
#30304=EDGE_CURVE ( 'NONE', #36194, #16873, #33726, .T. ) ;
#30308=DIRECTION ( 'NONE',  ( 0.000000000000000000, -0.000000000000000000, 1.000000000000000000 ) ) ;
#30322=CARTESIAN_POINT ( 'NONE',  ( 20.99999999999999289, 249.4937500012290457, -5.999999999999998224 ) ) ;
#30323=CARTESIAN_POINT ( 'NONE',  ( 15.24356964374999990, 249.3718750006145228, -3.323476615752268604 ) ) ;
#30328=CARTESIAN_POINT ( 'NONE',  ( -27.24356964375000345, 198.0593750006145513, 0.000000000000000000 ) ) ;
#30331=CARTESIAN_POINT ( 'NONE',  ( 15.24356964375000167, 244.0468750006145342, 3.323476615752272600 ) ) ;
#30337=ORIENTED_EDGE ( 'NONE', *, *, #14770, .F. ) ;
#30338=CARTESIAN_POINT ( 'NONE',  ( 15.24356964374999990, 247.0093750006145115, -3.323476615752268604 ) ) ;
#30346=EDGE_CURVE ( 'NONE', #27758, #8211, #33802, .T. ) ;
#30352=AXIS2_PLACEMENT_3D ( 'NONE', #5495, #31655, #17450 ) ;
#30354=CARTESIAN_POINT ( 'NONE',  ( 26.75643035624999655, 247.2343750006145058, 3.323476615752267271 ) ) ;
#30364=DIRECTION ( 'NONE',  ( 0.000000000000000000, -0.000000000000000000, 1.000000000000000000 ) ) ;
#30367=VERTEX_POINT ( 'NONE', #22621 ) ;
#30370=( BOUNDED_CURVE ( )  B_SPLINE_CURVE ( 2, ( #25458, #6057, #37010, #8913, #34176, #17834, #11054, #556, #34872 ),
 .UNSPECIFIED., .F., .F. ) 
 B_SPLINE_CURVE_WITH_KNOTS ( ( 3, 2, 2, 2, 3 ),
 ( 0.1630434782608695676, 0.1666666666666666574, 0.1739130434782608647, 0.1811594202898550721, 0.1847826086956521618 ),
 .UNSPECIFIED. ) 
 CURVE ( )  GEOMETRIC_REPRESENTATION_ITEM ( )  RATIONAL_B_SPLINE_CURVE ( ( 0.9330127018922194093, 0.9330127018922196314, 1.000000000000000000, 0.8660254037844387076, 1.000000000000000000, 0.8660254037844387076, 1.000000000000000000, 0.9330127018922196314, 0.9330127018922194093 ) ) 
 REPRESENTATION_ITEM ( '' )  );
#30376=CARTESIAN_POINT ( 'NONE',  ( 27.24356964374999635, 197.8718750006145513, -15.72908226750539029 ) ) ;
#30382=CARTESIAN_POINT ( 'NONE',  ( 15.00000000000000178, 244.2437500012290457, 3.464101615137757051 ) ) ;
#30390=CARTESIAN_POINT ( 'NONE',  ( 15.24356964374999990, 244.7593750006145115, -3.323476615752268604 ) ) ;
#30405=DIRECTION ( 'NONE',  ( -0.000000000000000000, 1.000000000000000000, -0.000000000000000000 ) ) ;
#30409=CARTESIAN_POINT ( 'NONE',  ( -28.40689544173954673, 204.5242310104925707, -5.838094896048071192 ) ) ;
#30415=DIRECTION ( 'NONE',  ( 0.000000000000000000, 1.000000000000000000, 0.000000000000000000 ) ) ;
#30417=EDGE_CURVE ( 'NONE', #30424, #7705, #1314, .T. ) ;
#30418=CARTESIAN_POINT ( 'NONE',  ( -7.946041369334237991, 195.0000000000000000, 26.05901981062767092 ) ) ;
#30420=LINE ( 'NONE', #33258, #3241 ) ;
#30422=CARTESIAN_POINT ( 'NONE',  ( 26.75643035624999655, 244.7218750006145456, -3.323476615752271268 ) ) ;
#30424=VERTEX_POINT ( 'NONE', #37368 ) ;
#30426=DIRECTION ( 'NONE',  ( -0.000000000000000000, 1.000000000000000000, -0.000000000000000000 ) ) ;
#30435=ORIENTED_EDGE ( 'NONE', *, *, #31453, .F. ) ;
#30437=DIRECTION ( 'NONE',  ( 0.000000000000000000, -1.000000000000000000, 0.000000000000000000 ) ) ;
#30439=CARTESIAN_POINT ( 'NONE',  ( 23.99999999999999645, 249.4562500012290229, -5.196152422706631135 ) ) ;
#30445=CARTESIAN_POINT ( 'NONE',  ( 7.136082524518490011, 215.1989690533051487, 3.001545256184956934 ) ) ;
#30458=CARTESIAN_POINT ( 'NONE',  ( 27.24356964375000700, 196.8406250006145513, 15.72908226750537075 ) ) ;
#30472=DIRECTION ( 'NONE',  ( 0.000000000000000000, 1.000000000000000000, 0.000000000000000000 ) ) ;
#30475=CARTESIAN_POINT ( 'NONE',  ( -4.500000000000002665, 244.5000000000000000, 2.500000000000000000 ) ) ;
#30484=CARTESIAN_POINT ( 'NONE',  ( 26.99999999999999645, 245.2750000000000057, -7.347880794884117764E-16 ) ) ;
#30488=EDGE_LOOP ( 'NONE', ( #15425, #34000, #22462, #13829 ) ) ;
#30490=CARTESIAN_POINT ( 'NONE',  ( -26.99999999999998934, 198.3500000012290627, 15.58845726811991561 ) ) ;
#30491=CARTESIAN_POINT ( 'NONE',  ( -27.00000000000000355, 196.8125000000000000, -15.58845726811989429 ) ) ;
#30494=CARTESIAN_POINT ( 'NONE',  ( 15.24356964374999990, 244.4593750006145569, 0.000000000000000000 ) ) ;
#30495=AXIS2_PLACEMENT_3D ( 'NONE', #36456, #36270, #25090 ) ;
#30502=CARTESIAN_POINT ( 'NONE',  ( 15.24356964374999990, 239.8468750006145171, 0.000000000000000000 ) ) ;
#30517=CARTESIAN_POINT ( 'NONE',  ( 21.00000000000000000, 249.5218750006145285, 6.646953231504538984 ) ) ;
#30522=CARTESIAN_POINT ( 'NONE',  ( -1.926257025242585782E-15, 198.3968750006145285, -31.45816453501076637 ) ) ;
#30525=CARTESIAN_POINT ( 'NONE',  ( 15.24356964375000167, 243.1468750006145285, 3.323476615752272600 ) ) ;
#30528=ORIENTED_EDGE ( 'NONE', *, *, #22083, .F. ) ;
#30532=CARTESIAN_POINT ( 'NONE',  ( 15.24356964375000167, 243.9343750006145228, 3.323476615752272600 ) ) ;
#30537=MECHANICAL_DESIGN_GEOMETRIC_PRESENTATION_REPRESENTATION('',(#1459),#14183);
#30548=CARTESIAN_POINT ( 'NONE',  ( 15.24356964374999990, 247.4968750006145228, 0.000000000000000000 ) ) ;
#30550=DIRECTION ( 'NONE',  ( 0.000000000000000000, 0.000000000000000000, -1.000000000000000000 ) ) ;
#30566=CARTESIAN_POINT ( 'NONE',  ( 22.60769515458672885, 244.0736538117967029, -5.999999999999998224 ) ) ;
#30568=EDGE_CURVE ( 'NONE', #33602, #30621, #13948, .T. ) ;
#30570=CARTESIAN_POINT ( 'NONE',  ( 20.99999999999995026, 242.7437500012290741, -5.999999999999998224 ) ) ;
#30571=CARTESIAN_POINT ( 'NONE',  ( 27.24356964375000700, 199.1468750006145285, 15.72908226750537075 ) ) ;
#30577=CARTESIAN_POINT ( 'NONE',  ( 18.00000000000000355, 240.6812500012290457, 5.196152422706632912 ) ) ;
#30580=CARTESIAN_POINT ( 'NONE',  ( 13.62178482187499640, 199.6531250006145228, -23.59362340125807123 ) ) ;
#30587=AXIS2_PLACEMENT_3D ( 'NONE', #33907, #37477, #19894 ) ;
#30594=CARTESIAN_POINT ( 'NONE',  ( -8.871229729697644117, 219.1703717126474089, -3.236093818008944467 ) ) ;
#30598=CARTESIAN_POINT ( 'NONE',  ( 27.00000000000001421, 199.7375000000000114, 15.58845726811988897 ) ) ;
#30602=CARTESIAN_POINT ( 'NONE',  ( 19.39230484541324273, 244.2986538117967257, 5.999999999999987566 ) ) ;
#30609=CARTESIAN_POINT ( 'NONE',  ( 21.00000000000000000, 240.2687500012290513, 5.999999999999998224 ) ) ;
#30610=AXIS2_PLACEMENT_3D ( 'NONE', #9031, #5992, #12242 ) ;
#30611=CARTESIAN_POINT ( 'NONE',  ( 15.24356964375000167, 247.1968750006145115, 3.323476615752272600 ) ) ;
#30613=CARTESIAN_POINT ( 'NONE',  ( 20.99999999999999645, 243.4468750006145399, -6.646953231504538984 ) ) ;
#30616=CYLINDRICAL_SURFACE ( 'NONE', #24715, 5.999999999999999112 ) ;
#30621=VERTEX_POINT ( 'NONE', #2087 ) ;
#30624=ORIENTED_EDGE ( 'NONE', *, *, #36935, .F. ) ;
#30628=CARTESIAN_POINT ( 'NONE',  ( -1.045839947578415010E-13, 195.1625000000000512, 27.00000000000000355 ) ) ;
#30633=CARTESIAN_POINT ( 'NONE',  ( 15.81961138684334678, 215.1803886131542640, 3.965927053047088258 ) ) ;
#30641=CARTESIAN_POINT ( 'NONE',  ( -27.24356964374999990, 195.2656250006145342, -15.72908226750537786 ) ) ;
#30646=CYLINDRICAL_SURFACE ( 'NONE', #29525, 5.999999999999999112 ) ;
#30656=CARTESIAN_POINT ( 'NONE',  ( 19.39230484541324628, 246.3075961894322745, -5.999999999999989342 ) ) ;
#30658=DIRECTION ( 'NONE',  ( 0.000000000000000000, 1.000000000000000000, 0.000000000000000000 ) ) ;
#30664=EDGE_LOOP ( 'NONE', ( #34644, #10310, #3118 ) ) ;
#30668=CARTESIAN_POINT ( 'NONE',  ( 24.00000000000000000, 245.6500000000000057, 5.196152422706629359 ) ) ;
#30676=CARTESIAN_POINT ( 'NONE',  ( -13.49999999999998401, 198.3875000012290286, 23.38268590217985476 ) ) ;
#30679=CARTESIAN_POINT ( 'NONE',  ( 26.75643035624999655, 244.1968750006145399, 3.323476615752267715 ) ) ;
#30682=CARTESIAN_POINT ( 'NONE',  ( 20.99999999999999645, 185.0294372515228645, -5.999999999999999112 ) ) ;
#30687=CARTESIAN_POINT ( 'NONE',  ( 13.62178482187499640, 198.8093750006145513, -23.59362340125807123 ) ) ;
#30698=DIRECTION ( 'NONE',  ( -0.000000000000000000, -1.000000000000000000, -0.000000000000000000 ) ) ;
#30701=CARTESIAN_POINT ( 'NONE',  ( 21.00000000000000000, 240.8593750006145342, 6.646953231504538984 ) ) ;
#30702=VERTEX_POINT ( 'NONE', #36764 ) ;
#30705=AXIS2_PLACEMENT_3D ( 'NONE', #5166, #21690, #2138 ) ;
#30707=CARTESIAN_POINT ( 'NONE',  ( -27.24356964374999279, 198.9968750006145513, 15.72908226750539384 ) ) ;
#30710=CARTESIAN_POINT ( 'NONE',  ( 20.99999999999999645, 243.8125000000000284, 5.999999999999998224 ) ) ;
#30711=CARTESIAN_POINT ( 'NONE',  ( 15.24356964375000167, 242.2468750006145228, 3.323476615752272600 ) ) ;
#30715=ORIENTED_EDGE ( 'NONE', *, *, #33294, .F. ) ;
#30717=CARTESIAN_POINT ( 'NONE',  ( 18.12178482187500350, 244.8718750006145228, 4.985214923628407568 ) ) ;
#30729=CARTESIAN_POINT ( 'NONE',  ( 23.87821517812499650, 244.6468750006145285, -4.985214923628404904 ) ) ;
#30730=VECTOR ( 'NONE', #2618, 1000.000000000000000 ) ;
#30731=PLANE ( 'NONE',  #18842 ) ;
#30734=CARTESIAN_POINT ( 'NONE',  ( 18.00000000000000355, 246.0250000000000057, 5.196152422706632912 ) ) ;
#30745=FACE_OUTER_BOUND ( 'NONE', #31343, .T. ) ;
#30750=CARTESIAN_POINT ( 'NONE',  ( 13.62178482187499640, 197.4593750006145285, -23.59362340125807123 ) ) ;
#30752=DIRECTION ( 'NONE',  ( 0.000000000000000000, 1.000000000000000000, 0.000000000000000000 ) ) ;
#30756=CARTESIAN_POINT ( 'NONE',  ( 21.00000000000000000, 241.8437500012290400, -6.928203230275506996 ) ) ;
#30757=VECTOR ( 'NONE', #36130, 999.9999999999998863 ) ;
#30760=CARTESIAN_POINT ( 'NONE',  ( -27.24356964375000345, 198.4531250006145342, 0.000000000000000000 ) ) ;
#30781=CARTESIAN_POINT ( 'NONE',  ( -28.98576012241837319, 202.0511556252696721, -1.045925494027194702 ) ) ;
#30787=CARTESIAN_POINT ( 'NONE',  ( 13.49999999999999645, 195.4625000012290172, -23.38268590217984766 ) ) ;
#30790=CARTESIAN_POINT ( 'NONE',  ( 21.00000000000000000, 248.8468750006145456, -6.646953231504538984 ) ) ;
#30792=CARTESIAN_POINT ( 'NONE',  ( 15.24356964375000167, 244.0468750006145342, 3.323476615752272600 ) ) ;
#30794=CARTESIAN_POINT ( 'NONE',  ( 21.00000000000000000, 249.0437500012290570, -6.928203230275506996 ) ) ;
#30804=VERTEX_POINT ( 'NONE', #22359 ) ;
#30807=CARTESIAN_POINT ( 'NONE',  ( 26.99999999999999645, 249.3437500012290400, 3.464101615137751278 ) ) ;
#30809=CARTESIAN_POINT ( 'NONE',  ( 26.75643035624999655, 249.0343750006145456, 3.323476615752267715 ) ) ;
#30812=EDGE_CURVE ( 'NONE', #25531, #23197, #34092, .T. ) ;
#30814=CARTESIAN_POINT ( 'NONE',  ( 5.128366027876307243, 215.9518627395465558, -0.7835069059934931524 ) ) ;
#30823=CARTESIAN_POINT ( 'NONE',  ( -27.24356964374999990, 196.6156250006145285, -15.72908226750537786 ) ) ;
#30838=CARTESIAN_POINT ( 'NONE',  ( 20.99999999999999289, 243.1937500012290343, -5.999999999999997335 ) ) ;
#30840=CARTESIAN_POINT ( 'NONE',  ( -13.49999999999998401, 197.8249999999999886, 23.38268590217985476 ) ) ;
#30844=CARTESIAN_POINT ( 'NONE',  ( 26.99999999999999645, 198.5750000012290570, -15.58845726811990495 ) ) ;
#30845=ORIENTED_EDGE ( 'NONE', *, *, #19625, .F. ) ;
#30850=CARTESIAN_POINT ( 'NONE',  ( 18.00000000000000355, 242.8750000000000000, 5.196152422706632912 ) ) ;
#30856=CARTESIAN_POINT ( 'NONE',  ( 26.99999999999999645, 198.5750000012290286, -15.58845726811990495 ) ) ;
#30860=CARTESIAN_POINT ( 'NONE',  ( 18.12178482187500350, 242.7343750006145342, 4.985214923628407568 ) ) ;
#30868=CARTESIAN_POINT ( 'NONE',  ( 13.62178482187501416, 197.3093750006145513, 23.59362340125806767 ) ) ;
#30876=AXIS2_PLACEMENT_3D ( 'NONE', #32628, #18240, #15392 ) ;
#30879=( BOUNDED_SURFACE ( )  B_SPLINE_SURFACE ( 3, 2, ( 
 ( #33283, #7507, #24564 ),
 ( #6753, #21174, #36117 ),
 ( #18327, #24382, #13194 ),
 ( #35927, #24747, #15477 ),
 ( #12629, #24194, #21915 ),
 ( #7321, #19081, #30252 ),
 ( #4096, #30633, #27593 ),
 ( #869, #12441, #35739 ),
 ( #32901, #9785, #18895 ),
 ( #16045, #21362, #6954 ),
 ( #18522, #15667, #1623 ),
 ( #27218, #18713, #15855 ),
 ( #30445, #36676, #16969 ),
 ( #13377, #34022, #19455 ),
 ( #10900, #19273, #34393 ),
 ( #22288, #22473, #8066 ),
 ( #22846, #31364, #14122 ),
 ( #28511, #4837, #5208 ),
 ( #25119, #33842, #28146 ),
 ( #20003, #13758, #16230 ),
 ( #19643, #31185, #16785 ),
 ( #37229, #37041, #7880 ),
 ( #2554, #16603, #25304 ),
 ( #27962, #13566, #27781 ),
 ( #7692, #11277, #11089 ),
 ( #30814, #24931, #33653 ),
 ( #2367, #31003, #16415 ),
 ( #25678, #5389, #36856 ),
 ( #36484, #10714, #1993 ),
 ( #28329, #22665, #34209 ),
 ( #13940, #5023, #2177 ),
 ( #25489, #8253, #19827 ),
 ( #8434, #4649, #1808 ),
 ( #10528, #22104, #29447 ),
 ( #31919, #5762, #6134 ),
 ( #14489, #31548, #15051 ),
 ( #8616, #12198, #29062 ),
 ( #6331, #31735, #2735 ),
 ( #8804, #14308, #261 ),
 ( #23772, #20185, #11638 ),
 ( #11825, #26046, #35311 ),
 ( #23396, #3293, #73 ),
 ( #26224, #17342, #23213 ),
 ( #17528, #34762, #9366 ),
 ( #5572, #446, #34944 ),
 ( #17157, #23027, #26600 ) ),
 .UNSPECIFIED., .F., .F., .F. ) 
 B_SPLINE_SURFACE_WITH_KNOTS ( ( 4, 2, 2, 2, 2, 2, 2, 2, 2, 2, 2, 2, 2, 2, 2, 2, 2, 2, 2, 2, 2, 2, 4 ),
 ( 3, 3 ),
 ( 4.712388980384689674, 4.908738521234051966, 5.105088062083414258, 5.301437602932775661, 5.497787143782137953, 5.694136684631500245, 5.792311455056180947, 5.890486225480861648, 5.988660995905542350, 6.086835766330223940, 6.185010536754905530, 6.283185307179586232, 6.381360077604266934, 6.479534848028948524, 6.577709618453630114, 6.675884388878310816, 6.774059159302991517, 6.872233929727672219, 7.068583470577034511, 7.264933011426396803, 7.461282552275758206, 7.657632093125120498, 7.853981633974482790 ),
 ( 0.000000000000000000, 1.000000000000000000 ),
 .UNSPECIFIED. ) 
 GEOMETRIC_REPRESENTATION_ITEM ( )  RATIONAL_B_SPLINE_SURFACE ( (
 ( 1.000000000000000000, 1.000000000000000000, 1.000000000000000000),
 ( 1.000000000000000000, 1.000009746410878364, 1.000000000000000000),
 ( 1.000000000000000000, 0.9967613244605102452, 1.000000000000000000),
 ( 1.000000000000000000, 0.9841171504872305853, 1.000000000000000000),
 ( 1.000000000000000000, 0.9747108043634977737, 1.000000000000000000),
 ( 1.000000000000000000, 0.9506740353988157866, 1.000000000000000000),
 ( 1.000000000000000000, 0.9360421842704774731, 1.000000000000000000),
 ( 1.000000000000000000, 0.9031650994159179380, 1.000000000000000000),
 ( 1.000000000000000000, 0.8849191471317067181, 1.000000000000000000),
 ( 1.000000000000000000, 0.8471316604371722514, 1.000000000000000000),
 ( 1.000000000000000000, 0.8275942695927370751, 1.000000000000000000),
 ( 1.000000000000000000, 0.7995620738861383137, 1.000000000000000000),
 ( 1.000000000000000000, 0.7904353558348173880, 1.000000000000000000),
 ( 1.000000000000000000, 0.7730318702305081224, 1.000000000000000000),
 ( 1.000000000000000000, 0.7647559708311986171, 1.000000000000000000),
 ( 1.000000000000000000, 0.7494742688660065433, 1.000000000000000000),
 ( 1.000000000000000000, 0.7424696633570816440, 1.000000000000000000),
 ( 1.000000000000000000, 0.7301234195064296717, 1.000000000000000000),
 ( 1.000000000000000000, 0.7247831711438370572, 1.000000000000000000),
 ( 1.000000000000000000, 0.7160917253994798504, 1.000000000000000000),
 ( 1.000000000000000000, 0.7127418075764269112, 1.000000000000000000),
 ( 1.000000000000000000, 0.7082489452424536314, 1.000000000000000000),
 ( 1.000000000000000000, 0.7071067811865475727, 1.000000000000000000),
 ( 1.000000000000000000, 0.7071067811865475727, 1.000000000000000000),
 ( 1.000000000000000000, 0.7082489452424827192, 1.000000000000000000),
 ( 1.000000000000000000, 0.7127418075763976013, 1.000000000000000000),
 ( 1.000000000000000000, 0.7160917253994796283, 1.000000000000000000),
 ( 1.000000000000000000, 0.7247831711438368352, 1.000000000000000000),
 ( 1.000000000000000000, 0.7301234195064293386, 1.000000000000000000),
 ( 1.000000000000000000, 0.7424696633570813109, 1.000000000000000000),
 ( 1.000000000000000000, 0.7494742688657879404, 1.000000000000000000),
 ( 1.000000000000000000, 0.7647559708314156657, 1.000000000000000000),
 ( 1.000000000000000000, 0.7730318702303776712, 1.000000000000000000),
 ( 1.000000000000000000, 0.7904353558349440645, 1.000000000000000000),
 ( 1.000000000000000000, 0.7995620738860717003, 1.000000000000000000),
 ( 1.000000000000000000, 0.8275942695928699688, 1.000000000000000000),
 ( 1.000000000000000000, 0.8471316604371704750, 1.000000000000000000),
 ( 1.000000000000000000, 0.8849191471317049418, 1.000000000000000000),
 ( 1.000000000000000000, 0.9031650994159176049, 1.000000000000000000),
 ( 1.000000000000000000, 0.9360421842704771400, 1.000000000000000000),
 ( 1.000000000000000000, 0.9506740353988152314, 1.000000000000000000),
 ( 1.000000000000000000, 0.9747108043634972185, 1.000000000000000000),
 ( 1.000000000000000000, 0.9841171504871490949, 1.000000000000000000),
 ( 1.000000000000000000, 0.9967613244605915135, 1.000000000000000000),
 ( 1.000000000000000000, 1.000009746410817302, 1.000000000000000000),
 ( 1.000000000000000000, 1.000000000000000000, 1.000000000000000000) ) ) 
 REPRESENTATION_ITEM ( '' )  SURFACE ( )  );
#30883=ORIENTED_EDGE ( 'NONE', *, *, #29518, .F. ) ;
#30886=CARTESIAN_POINT ( 'NONE',  ( 27.24356964375000345, 197.8343750006145569, -3.336375036156643733E-15 ) ) ;
#30889=CARTESIAN_POINT ( 'NONE',  ( 18.00000000000000355, 239.7812500012290400, 5.196152422706632912 ) ) ;
#30890=CARTESIAN_POINT ( 'NONE',  ( 26.75643035624999655, 240.6343750006145115, -7.049594010296217766E-16 ) ) ;
#30898=CARTESIAN_POINT ( 'NONE',  ( 26.75643035624999655, 244.6093750006145342, -3.323476615752271712 ) ) ;
#30910=EDGE_CURVE ( 'NONE', #18816, #11333, #33321, .T. ) ;
#30912=CARTESIAN_POINT ( 'NONE',  ( 15.24356964375000167, 245.2843750006145171, 3.323476615752272600 ) ) ;
#30917=EDGE_CURVE ( 'NONE', #23609, #4638, #33759, .T. ) ;
#30927=ORIENTED_EDGE ( 'NONE', *, *, #198, .T. ) ;
#30928=CARTESIAN_POINT ( 'NONE',  ( -29.00000000000002487, 210.0000000000000000, 0.000000000000000000 ) ) ;
#30934=CARTESIAN_POINT ( 'NONE',  ( -27.24356964374999635, 198.9968750006145228, 15.72908226750539384 ) ) ;
#30940=CARTESIAN_POINT ( 'NONE',  ( 18.00000000000000000, 241.8812500012290343, -5.196152422706630247 ) ) ;
#30942=EDGE_CURVE ( 'NONE', #28321, #190, #25375, .T. ) ;
#30944=CARTESIAN_POINT ( 'NONE',  ( -13.62178482187500528, 197.4781250006145399, -23.59362340125807123 ) ) ;
#30955=EDGE_CURVE ( 'NONE', #23622, #22557, #25560, .T. ) ;
#30956=CARTESIAN_POINT ( 'NONE',  ( -27.00000000000000355, 196.3625000000000114, -15.58845726811989429 ) ) ;
#30979=CARTESIAN_POINT ( 'NONE',  ( 23.87821517812499650, 247.4593750006145285, -4.985214923628404904 ) ) ;
#30981=CARTESIAN_POINT ( 'NONE',  ( 26.75643035624999655, 241.0843750006145285, -7.049594010296217766E-16 ) ) ;
#30982=EDGE_LOOP ( 'NONE', ( #18629, #8606, #36201, #23204 ) ) ;
#30985=CARTESIAN_POINT ( 'NONE',  ( 15.00000000000000000, 248.2562500012290627, 0.000000000000000000 ) ) ;
#30992=ORIENTED_EDGE ( 'NONE', *, *, #13066, .F. ) ;
#31000=CARTESIAN_POINT ( 'NONE',  ( 21.00000000000000000, 248.2843750006145171, -6.646953231504538984 ) ) ;
#31003=CARTESIAN_POINT ( 'NONE',  ( 14.82946893053589221, 216.1705310694575246, 0.5774388102998520012 ) ) ;
#31011=CARTESIAN_POINT ( 'NONE',  ( -27.24356964374999635, 195.7906250006145115, 15.72908226750539384 ) ) ;
#31028=CARTESIAN_POINT ( 'NONE',  ( 13.49999999999999645, 196.7000000000000171, -23.38268590217984766 ) ) ;
#31032=CARTESIAN_POINT ( 'NONE',  ( 20.99999999999999645, 247.9468750006144830, -6.646953231504538984 ) ) ;
#31039=CARTESIAN_POINT ( 'NONE',  ( 24.00000000000000000, 243.8500000000000227, 5.196152422706629359 ) ) ;
#31041=ADVANCED_FACE ( 'NONE', ( #32365 ), #26674, .F. ) ;
#31046=CARTESIAN_POINT ( 'NONE',  ( -1.909035429704832693E-15, 198.2000000012290286, -31.17691453623979214 ) ) ;
#31050=CARTESIAN_POINT ( 'NONE',  ( 18.12178482187499640, 242.1343750006145115, -4.985214923628404904 ) ) ;
#31057=CARTESIAN_POINT ( 'NONE',  ( 27.24356964374999635, 199.2218750006145456, -15.72908226750539029 ) ) ;
#31061=CARTESIAN_POINT ( 'NONE',  ( 26.99999999999999645, 245.2375000000000114, 3.464101615137751278 ) ) ;
#31072=CARTESIAN_POINT ( 'NONE',  ( 24.00000000000000000, 240.3062500012290457, 5.196152422706629359 ) ) ;
#31073=ORIENTED_EDGE ( 'NONE', *, *, #17731, .F. ) ;
#31076=CARTESIAN_POINT ( 'NONE',  ( 27.24356964374999279, 197.8718750006145513, -15.72908226750539207 ) ) ;
#31079=CARTESIAN_POINT ( 'NONE',  ( -29.00000000000002487, 210.0000000000000000, 0.000000000000000000 ) ) ;
#31080=CARTESIAN_POINT ( 'NONE',  ( 18.12178482187500350, 240.4843750006145342, 4.985214923628407568 ) ) ;
#31081=CARTESIAN_POINT ( 'NONE',  ( 20.99999999999997868, 210.0000000000000000, 0.000000000000000000 ) ) ;
#31085=EDGE_LOOP ( 'NONE', ( #7365, #22696, #23742, #36666 ) ) ;
#31086=CARTESIAN_POINT ( 'NONE',  ( 15.24356964374999990, 245.6968750006145115, 0.000000000000000000 ) ) ;
#31093=EDGE_CURVE ( 'NONE', #24290, #27888, #37355, .T. ) ;
#31100=CARTESIAN_POINT ( 'NONE',  ( 26.75643035624999655, 244.0843750006145285, 3.323476615752267271 ) ) ;
#31106=AXIS2_PLACEMENT_3D ( 'NONE', #32311, #26812, #27003 ) ;
#31109=CARTESIAN_POINT ( 'NONE',  ( -27.00000000000000355, 199.5124999999999886, -15.58845726811989429 ) ) ;
#31115=DIRECTION ( 'NONE',  ( -0.000000000000000000, 1.000000000000000000, -0.000000000000000000 ) ) ;
#31122=CARTESIAN_POINT ( 'NONE',  ( 27.24356964374999635, 196.9718750006145456, -15.72908226750539029 ) ) ;
#31124=CIRCLE ( 'NONE', #14779, 5.999999999999999112 ) ;
#31129=CARTESIAN_POINT ( 'NONE',  ( 21.00000000000000000, 240.7187500012290400, 6.928203230275506996 ) ) ;
#31147=CARTESIAN_POINT ( 'NONE',  ( -5.732297079746171420, 222.9518338469886203, -2.500000000000000000 ) ) ;
#31162=CARTESIAN_POINT ( 'NONE',  ( 18.00000000000000355, 247.8249999999999886, 5.196152422706632912 ) ) ;
#31163=CARTESIAN_POINT ( 'NONE',  ( 26.75643035624999655, 246.8968750006145285, 3.323476615752267715 ) ) ;
#31165=CARTESIAN_POINT ( 'NONE',  ( 18.12178482187499640, 241.6843750006145513, -4.985214923628404904 ) ) ;
#31169=EDGE_CURVE ( 'NONE', #32379, #10385, #7420, .T. ) ;
#31170=CARTESIAN_POINT ( 'NONE',  ( 21.00000000000000000, 248.5937500012290116, -6.928203230275506996 ) ) ;
#31181=LINE ( 'NONE', #28506, #10631 ) ;
#31185=CARTESIAN_POINT ( 'NONE',  ( 14.89154389910886600, 216.1084561008947844, -0.4848545222721730164 ) ) ;
#31187=LINE ( 'NONE', #1995, #27496 ) ;
#31193=CARTESIAN_POINT ( 'NONE',  ( 27.24356964375000345, 196.8781250006145171, -3.336375036156643733E-15 ) ) ;
#31208=CARTESIAN_POINT ( 'NONE',  ( 13.49999999999999645, 197.1500000000000057, -23.38268590217984766 ) ) ;
#31212=CARTESIAN_POINT ( 'NONE',  ( 15.24356964375000167, 248.5468750006145342, 3.323476615752272600 ) ) ;
#31219=CARTESIAN_POINT ( 'NONE',  ( 21.00000000000000000, 243.5875000000000057, -6.928203230275506996 ) ) ;
#31225=CARTESIAN_POINT ( 'NONE',  ( -26.99999999999998934, 194.7500000012290400, 15.58845726811991561 ) ) ;
#31229=AXIS2_PLACEMENT_3D ( 'NONE', #35818, #6827, #29952 ) ;
#31230=CARTESIAN_POINT ( 'NONE',  ( 26.75643035624999655, 241.9843750006145342, -7.049594010296217766E-16 ) ) ;
#31237=CARTESIAN_POINT ( 'NONE',  ( 13.62178482187499640, 199.2593750006145399, -23.59362340125807123 ) ) ;
#31253=CARTESIAN_POINT ( 'NONE',  ( 1.120210788295102201E-13, 195.8375000000000057, -27.00000000000000711 ) ) ;
#31254=CARTESIAN_POINT ( 'NONE',  ( 21.00000000000000000, 248.3687500012290741, 5.999999999999998224 ) ) ;
#31255=ORIENTED_EDGE ( 'NONE', *, *, #12973, .T. ) ;
#31258=CARTESIAN_POINT ( 'NONE',  ( -27.24356964375000345, 195.3593750006145342, 0.000000000000000000 ) ) ;
#31262=CARTESIAN_POINT ( 'NONE',  ( 21.00000000000000000, 241.1968750006145399, -6.646953231504538984 ) ) ;
#31268=CARTESIAN_POINT ( 'NONE',  ( 18.12178482187500350, 244.4218750006145058, 4.985214923628407568 ) ) ;
#31280=CARTESIAN_POINT ( 'NONE',  ( 26.75643035624999655, 243.7093750006144717, -3.323476615752271268 ) ) ;
#31281=CARTESIAN_POINT ( 'NONE',  ( -29.00000000000002487, 222.9518338469886203, 12.50000000000000000 ) ) ;
#31285=EDGE_CURVE ( 'NONE', #14644, #6593, #3532, .T. ) ;
#31299=( BOUNDED_CURVE ( )  B_SPLINE_CURVE ( 2, ( #24746, #30251, #35554, #4278, #9599, #21361, #18326, #1054, #36116 ),
 .UNSPECIFIED., .F., .F. ) 
 B_SPLINE_CURVE_WITH_KNOTS ( ( 3, 2, 2, 2, 3 ),
 ( 0.5760869565217391353, 0.5797101449275362528, 0.5869565217391304879, 0.5942028985507246119, 0.5978260869565217295 ),
 .UNSPECIFIED. ) 
 CURVE ( )  GEOMETRIC_REPRESENTATION_ITEM ( )  RATIONAL_B_SPLINE_CURVE ( ( 0.9330127018922194093, 0.9330127018922194093, 1.000000000000000000, 0.8660254037844387076, 1.000000000000000000, 0.8660254037844387076, 1.000000000000000000, 0.9330127018922194093, 0.9330127018922194093 ) ) 
 REPRESENTATION_ITEM ( '' )  );
#31301=CARTESIAN_POINT ( 'NONE',  ( -1.926257025242585782E-15, 196.1468750006145285, -31.45816453501075927 ) ) ;
#31303=DIRECTION ( 'NONE',  ( -0.000000000000000000, 1.000000000000000000, -0.000000000000000000 ) ) ;
#31306=ORIENTED_EDGE ( 'NONE', *, *, #4954, .F. ) ;
#31307=CARTESIAN_POINT ( 'NONE',  ( 21.00000000000000000, 241.1687500012290570, 6.928203230275506996 ) ) ;
#31314=CARTESIAN_POINT ( 'NONE',  ( 15.00000000000000000, 246.0062500012290627, 0.000000000000000000 ) ) ;
#31316=( BOUNDED_CURVE ( )  B_SPLINE_CURVE ( 2, ( #11325, #25912, #22895, #37457, #34442, #31598, #11507, #34622, #23263 ),
 .UNSPECIFIED., .F., .F. ) 
 B_SPLINE_CURVE_WITH_KNOTS ( ( 3, 2, 2, 2, 3 ),
 ( 0.6413043478260869179, 0.6449275362318840354, 0.6521739130434782705, 0.6594202898550725056, 0.6630434782608695121 ),
 .UNSPECIFIED. ) 
 CURVE ( )  GEOMETRIC_REPRESENTATION_ITEM ( )  RATIONAL_B_SPLINE_CURVE ( ( 0.9330127018922194093, 0.9330127018922194093, 1.000000000000000000, 0.8660254037844387076, 1.000000000000000000, 0.8660254037844387076, 1.000000000000000000, 0.9330127018922202975, 0.9330127018922192983 ) ) 
 REPRESENTATION_ITEM ( '' )  );
#31337=( NAMED_UNIT ( * ) SI_UNIT ( $, .STERADIAN. ) SOLID_ANGLE_UNIT ( ) );
#31340=CARTESIAN_POINT ( 'NONE',  ( 26.75643035624999655, 247.8718750006145228, -3.323476615752271712 ) ) ;
#31342=CARTESIAN_POINT ( 'NONE',  ( 15.24356964375000167, 242.2468750006145228, 3.323476615752272600 ) ) ;
#31343=EDGE_LOOP ( 'NONE', ( #33695, #4880, #12709, #27299, #17331 ) ) ;
#31346=CARTESIAN_POINT ( 'NONE',  ( 18.00000000000000355, 247.8812500012290343, 5.196152422706632912 ) ) ;
#31355=ORIENTED_EDGE ( 'NONE', *, *, #14775, .F. ) ;
#31361=CARTESIAN_POINT ( 'NONE',  ( 21.00000000000000000, 248.7343750006145342, -6.646953231504538984 ) ) ;
#31364=CARTESIAN_POINT ( 'NONE',  ( 14.43174379454686829, 216.5682562054522009, -0.6968546016497452200 ) ) ;
#31380=CARTESIAN_POINT ( 'NONE',  ( 20.99999999999999289, 242.2937500012290570, -5.999999999999997335 ) ) ;
#31383=EDGE_CURVE ( 'NONE', #11836, #6657, #2531, .T. ) ;
#31389=DIRECTION ( 'NONE',  ( 0.000000000000000000, 0.000000000000000000, 1.000000000000000000 ) ) ;
#31393=CARTESIAN_POINT ( 'NONE',  ( -27.00000000000000355, 198.1625000000000227, -15.58845726811989429 ) ) ;
#31398=CARTESIAN_POINT ( 'NONE',  ( 23.87821517812499650, 248.8093750006145228, -4.985214923628404904 ) ) ;
#31401=CARTESIAN_POINT ( 'NONE',  ( 14.99999999999999289, 204.0000000000000000, 0.000000000000000000 ) ) ;
#31405=CARTESIAN_POINT ( 'NONE',  ( 18.00000000000000355, 244.6750000000000114, 5.196152422706632912 ) ) ;
#31410=CARTESIAN_POINT ( 'NONE',  ( -26.99999999999998934, 196.5500000012290229, 15.58845726811991561 ) ) ;
#31411=CARTESIAN_POINT ( 'NONE',  ( 20.99999999999999645, 243.4187500012290002, 5.999999999999998224 ) ) ;
#31412=ADVANCED_FACE ( 'NONE', ( #7351 ), #6778, .F. ) ;
#31415=CARTESIAN_POINT ( 'NONE',  ( 21.00000000000000000, 242.5468750006145342, -6.646953231504538984 ) ) ;
#31422=CARTESIAN_POINT ( 'NONE',  ( 22.69185864259442198, 195.0000000000000284, -14.73983514314510401 ) ) ;
#31423=CARTESIAN_POINT ( 'NONE',  ( 27.24356964375000700, 197.3468750006145740, 15.72908226750537075 ) ) ;
#31425=ADVANCED_FACE ( 'NONE', ( #18353 ), #15506, .F. ) ;
#31427=CARTESIAN_POINT ( 'NONE',  ( 15.00000000000000178, 240.5875000000000057, 3.464101615137757051 ) ) ;
#31432=CARTESIAN_POINT ( 'NONE',  ( 26.99999999999999645, 197.2250000012290343, -15.58845726811990495 ) ) ;
#31434=CARTESIAN_POINT ( 'NONE',  ( 19.39230484541326049, 249.4575961894323655, -5.999999999999997335 ) ) ;
#31438=EDGE_LOOP ( 'NONE', ( #13695, #19856, #9127, #29386, #14836 ) ) ;
#31441=CARTESIAN_POINT ( 'NONE',  ( -13.62178482187500528, 195.2843750006145456, -23.59362340125807123 ) ) ;
#31445=CARTESIAN_POINT ( 'NONE',  ( 26.75643035624999655, 241.5718750006145115, -3.323476615752271712 ) ) ;
#31446=CARTESIAN_POINT ( 'NONE',  ( -27.24356964375000345, 197.5531250006145285, 0.000000000000000000 ) ) ;
#31451=CARTESIAN_POINT ( 'NONE',  ( 18.12178482187499640, 241.5718750006145399, -4.985214923628404904 ) ) ;
#31453=EDGE_CURVE ( 'NONE', #3975, #25890, #15696, .T. ) ;
#31460=CARTESIAN_POINT ( 'NONE',  ( 26.75643035624999655, 245.0218750006145001, -7.049594010296217766E-16 ) ) ;
#31468=CARTESIAN_POINT ( 'NONE',  ( 20.99999999999995026, 240.9437500012290911, -5.999999999999998224 ) ) ;
#31482=CARTESIAN_POINT ( 'NONE',  ( -27.24356964374999635, 195.3968750006145569, 15.72908226750539384 ) ) ;
#31483=EDGE_CURVE ( 'NONE', #5552, #23197, #17825, .T. ) ;
#31484=CARTESIAN_POINT ( 'NONE',  ( 26.99999999999999645, 246.2124999999999773, -3.464101615137755275 ) ) ;
#31485=LINE ( 'NONE', #22966, #3021 ) ;
#31489=CARTESIAN_POINT ( 'NONE',  ( 26.75643035624999655, 249.0343750006145456, 3.323476615752267715 ) ) ;
#31503=CARTESIAN_POINT ( 'NONE',  ( -23.43450404749491156, 195.0000000000001137, -13.63327128574096037 ) ) ;
#31508=CARTESIAN_POINT ( 'NONE',  ( -28.78272864601244763, 202.8264516967929865, 3.550837175518763544 ) ) ;
#31515=VERTEX_POINT ( 'NONE', #30475 ) ;
#31523=CARTESIAN_POINT ( 'NONE',  ( 26.75643035624999655, 244.6468750006145285, 3.323476615752267715 ) ) ;
#31525=CARTESIAN_POINT ( 'NONE',  ( 26.75643035624999655, 242.8843750006145115, -7.049594010296217766E-16 ) ) ;
#31527=VERTEX_POINT ( 'NONE', #18551 ) ;
#31530=CARTESIAN_POINT ( 'NONE',  ( 21.00000000000000000, 249.4937500012290741, -6.928203230275506996 ) ) ;
#31531=ORIENTED_EDGE ( 'NONE', *, *, #17031, .F. ) ;
#31539=( BOUNDED_CURVE ( )  B_SPLINE_CURVE ( 2, ( #2511, #20337, #11044, #17489, #22620, #11420, #3067, #5720, #17301 ),
 .UNSPECIFIED., .F., .F. ) 
 B_SPLINE_CURVE_WITH_KNOTS ( ( 3, 2, 2, 2, 3 ),
 ( 0.3125000000000000000, 0.3194444444444444198, 0.3333333333333333148, 0.3472222222222222099, 0.3541666666666666852 ),
 .UNSPECIFIED. ) 
 CURVE ( )  GEOMETRIC_REPRESENTATION_ITEM ( )  RATIONAL_B_SPLINE_CURVE ( ( 0.9330127018922194093, 0.9330127018922194093, 1.000000000000000000, 0.8660254037844387076, 1.000000000000000000, 0.8660254037844387076, 1.000000000000000000, 0.9330127018922190762, 0.9330127018922194093 ) ) 
 REPRESENTATION_ITEM ( '' )  );
#31544=CARTESIAN_POINT ( 'NONE',  ( 15.24356964374999990, 248.3968750006145285, 0.000000000000000000 ) ) ;
#31548=CARTESIAN_POINT ( 'NONE',  ( 14.06021656787535434, 216.9397834321072480, -0.8200469388708427898 ) ) ;
#31560=CARTESIAN_POINT ( 'NONE',  ( 26.99999999999999645, 248.9312500012290457, -7.347880794884117764E-16 ) ) ;
#31571=CARTESIAN_POINT ( 'NONE',  ( 15.00000000000000178, 243.3437500012290400, 3.464101615137757051 ) ) ;
#31573=CARTESIAN_POINT ( 'NONE',  ( -13.50000000000000533, 197.6750000000000114, -23.38268590217984411 ) ) ;
#31574=CARTESIAN_POINT ( 'NONE',  ( 15.00000000000000178, 240.1375000000000171, 3.464101615137757051 ) ) ;
#31576=CARTESIAN_POINT ( 'NONE',  ( 26.75643035624999655, 249.2218750006145171, -3.323476615752271268 ) ) ;
#31584=CARTESIAN_POINT ( 'NONE',  ( 24.00000000000000000, 243.4000000000000057, 5.196152422706629359 ) ) ;
#31587=ORIENTED_EDGE ( 'NONE', *, *, #18960, .T. ) ;
#31588=ORIENTED_EDGE ( 'NONE', *, *, #12470, .T. ) ;
#31591=CARTESIAN_POINT ( 'NONE',  ( 13.49999999999999645, 196.3625000012290513, -23.38268590217984766 ) ) ;
#31596=CARTESIAN_POINT ( 'NONE',  ( 26.75643035624999655, 243.8218750006145399, -3.323476615752271712 ) ) ;
#31598=CARTESIAN_POINT ( 'NONE',  ( 15.00000000000000000, 242.8187500012290343, -3.464101615137752610 ) ) ;
#31602=CARTESIAN_POINT ( 'NONE',  ( 27.05874960237330384, 195.0000000000000000, 2.090475941528396220 ) ) ;
#31603=CARTESIAN_POINT ( 'NONE',  ( 27.24356964374999635, 195.6218750006145228, -15.72908226750539029 ) ) ;
#31607=CARTESIAN_POINT ( 'NONE',  ( 15.00000000000000000, 240.5500000000000114, 0.000000000000000000 ) ) ;
#31609=CARTESIAN_POINT ( 'NONE',  ( 20.99999999999999289, 241.7874999999999659, -5.999999999999997335 ) ) ;
#31617=CARTESIAN_POINT ( 'NONE',  ( 22.60769515458673951, 249.6825961894323882, 5.999999999999998224 ) ) ;
#31619=ORIENTED_EDGE ( 'NONE', *, *, #670, .F. ) ;
#31622=CARTESIAN_POINT ( 'NONE',  ( 3.373323998396211998, 195.0311615700027801, 29.51057501647288461 ) ) ;
#31626=CARTESIAN_POINT ( 'NONE',  ( 21.00000000000000000, 240.0718750006145399, 6.646953231504538984 ) ) ;
#31627=CARTESIAN_POINT ( 'NONE',  ( -13.62178482187500528, 199.7281250006145399, -23.59362340125807123 ) ) ;
#31632=CARTESIAN_POINT ( 'NONE',  ( 5.778771075727756162E-15, 197.6656250006145399, 31.45816453501075927 ) ) ;
#31633=CARTESIAN_POINT ( 'NONE',  ( 15.24356964374999990, 241.1593750006145171, -3.323476615752268604 ) ) ;
#31635=CARTESIAN_POINT ( 'NONE',  ( 15.00000000000000178, 243.7374999999999829, 3.464101615137757051 ) ) ;
#31644=CARTESIAN_POINT ( 'NONE',  ( 26.75643035624999655, 242.8093750006144944, -3.323476615752271268 ) ) ;
#31651=CARTESIAN_POINT ( 'NONE',  ( 5.438367727407757775E-14, 197.7500000012290400, -27.00000000000000355 ) ) ;
#31652=FACE_OUTER_BOUND ( 'NONE', #9872, .T. ) ;
#31655=DIRECTION ( 'NONE',  ( 0.000000000000000000, 1.000000000000000000, 0.000000000000000000 ) ) ;
#31663=VECTOR ( 'NONE', #7657, 1000.000000000000000 ) ;
#31664=DIRECTION ( 'NONE',  ( 0.000000000000000000, 0.000000000000000000, -1.000000000000000000 ) ) ;
#31673=CARTESIAN_POINT ( 'NONE',  ( 23.87821517812500005, 248.5468750006145058, 4.985214923628404016 ) ) ;
#31699=EDGE_CURVE ( 'NONE', #17695, #6301, #25334, .T. ) ;
#31701=ORIENTED_EDGE ( 'NONE', *, *, #11660, .T. ) ;
#31710=CARTESIAN_POINT ( 'NONE',  ( 23.87821517812500005, 245.0593750006145228, 4.985214923628404016 ) ) ;
#31712=CARTESIAN_POINT ( 'NONE',  ( 26.75643035624999655, 242.4718750006145456, -3.323476615752271268 ) ) ;
#31713=ORIENTED_EDGE ( 'NONE', *, *, #26383, .T. ) ;
#31716=CARTESIAN_POINT ( 'NONE',  ( 15.00000000000000178, 247.3937500012290229, 3.464101615137757051 ) ) ;
#31717=EDGE_LOOP ( 'NONE', ( #6093, #1690, #28138, #10332 ) ) ;
#31731=CARTESIAN_POINT ( 'NONE',  ( 26.75643035624999655, 247.7593750006145399, -3.323476615752271712 ) ) ;
#31735=CARTESIAN_POINT ( 'NONE',  ( 14.62176384545913699, 216.3782361545713400, -2.408991313803013679 ) ) ;
#31746=EDGE_LOOP ( 'NONE', ( #1232, #12363, #25642, #33084, #18804, #31073, #24279, #23533, #3615, #34240, #31355, #14577, #5941, #11630, #15710, #12097, #9766, #27205, #2307, #8377, #11982, #2349, #7336, #2397, #12803, #4691 ) ) ;
#31754=CARTESIAN_POINT ( 'NONE',  ( 20.99999999999999645, 240.2687500012290513, 5.999999999999998224 ) ) ;
#31758=CARTESIAN_POINT ( 'NONE',  ( -13.49999999999998401, 195.5749999999999886, 23.38268590217985476 ) ) ;
#31761=CARTESIAN_POINT ( 'NONE',  ( 26.75643035624999655, 249.1843750006145228, -7.049594010296217766E-16 ) ) ;
#31767=CARTESIAN_POINT ( 'NONE',  ( 18.00000000000000000, 242.2749999999999773, -5.196152422706630247 ) ) ;
#31772=CARTESIAN_POINT ( 'NONE',  ( -27.00000000000000355, 196.0625000012290400, 0.000000000000000000 ) ) ;
#31773=CARTESIAN_POINT ( 'NONE',  ( -13.49999999999998401, 196.5875000012290457, 23.38268590217985476 ) ) ;
#31775=CARTESIAN_POINT ( 'NONE',  ( 22.60769515458673595, 249.2325961894323711, 5.999999999999999112 ) ) ;
#31776=CARTESIAN_POINT ( 'NONE',  ( 18.12178482187500350, 240.4843750006145342, 4.985214923628407568 ) ) ;
#31785=CARTESIAN_POINT ( 'NONE',  ( 5.778771075727756162E-15, 196.8218750006145399, 31.45816453501075927 ) ) ;
#31787=EDGE_LOOP ( 'NONE', ( #37401, #36896 ) ) ;
#31790=CARTESIAN_POINT ( 'NONE',  ( 0.000000000000000000, 195.0000000000000000, 0.000000000000000000 ) ) ;
#31794=CARTESIAN_POINT ( 'NONE',  ( 20.99999999999997868, 244.7687500012290513, 5.999999999999999112 ) ) ;
#31797=CARTESIAN_POINT ( 'NONE',  ( 22.60769515458672885, 245.8174038105676971, -5.999999999999998224 ) ) ;
#31799=CARTESIAN_POINT ( 'NONE',  ( 26.99999999999999645, 249.8125000000000000, -3.464101615137755275 ) ) ;
#31805=CARTESIAN_POINT ( 'NONE',  ( -13.62178482187498396, 195.8843750006145399, 23.59362340125808188 ) ) ;
#31809=CARTESIAN_POINT ( 'NONE',  ( 21.00000000000000000, 247.1875000000000000, -6.928203230275506996 ) ) ;
#31810=CARTESIAN_POINT ( 'NONE',  ( -13.62178482187500528, 198.8281250006145342, -23.59362340125807123 ) ) ;
#31816=CARTESIAN_POINT ( 'NONE',  ( -27.24356964375000345, 199.3531250006145399, 0.000000000000000000 ) ) ;
#31817=CARTESIAN_POINT ( 'NONE',  ( 26.75643035624999655, 243.2218750006145171, -7.049594010296217766E-16 ) ) ;
#31822=CARTESIAN_POINT ( 'NONE',  ( 18.12178482187499640, 247.5343750006145456, -4.985214923628404904 ) ) ;
#31826=ADVANCED_FACE ( 'NONE', ( #19482 ), #2393, .F. ) ;
#31827=CARTESIAN_POINT ( 'NONE',  ( 15.24356964374999990, 242.5468750006145058, 0.000000000000000000 ) ) ;
#31834=LINE ( 'NONE', #5867, #19191 ) ;
#31840=( BOUNDED_CURVE ( )  B_SPLINE_CURVE ( 2, ( #22552, #8697, #31627, #2627, #9073, #32000, #14573, #11169, #25944, #5847, #22742, #11722, #20643, #28406, #6030, #5289, #17616, #16869, #20083, #28589, #37487, #2816, #37121, #26125, #2445, #26307, #31810, #5469, #14019, #25569, #23476, #29146, #34292, #5655, #34473, #8335, #22928, #14386, #11538, #28964, #8516, #28776, #23109, #11909, #11357, #19905, #3187, #17237, #14203, #3003, #34653, #20271, #25754, #157, #23296, #17425, #34841, #8881, #20459, #35029, #31446, #14762, #37307, #17051, #344, #526, #15515, #15325, #27257, #32375, #21025, #32938, #6992, #32560, #6413, #21212, #15132, #12093, #12286, #29340, #23667, #21398, #907, #27071, #35967, #35211, #1095, #6602, #23859, #12664, #35398, #9261, #14947, #32751, #9820, #24420, #18560, #3571, #29911, #9635, #9446, #29531, #6224, #18176, #35590, #29717, #26684, #24232, #3750, #26876, #12477, #24045, #714, #10005, #6788, #4134, #17988, #18363, #3940, #35776, #32190, #30102, #15706, #20833, #1280, #26494, #12851, #17797, #3378, #16644, #16455 ),
 .UNSPECIFIED., .F., .F. ) 
 B_SPLINE_CURVE_WITH_KNOTS ( ( 3, 2, 2, 2, 2, 2, 2, 2, 2, 2, 2, 2, 2, 2, 2, 2, 2, 2, 2, 2, 2, 2, 2, 2, 2, 2, 2, 2, 2, 2, 2, 2, 2, 2, 2, 2, 2, 2, 2, 2, 2, 2, 2, 2, 2, 2, 2, 2, 2, 2, 2, 2, 2, 2, 2, 2, 2, 2, 2, 2, 2, 2, 2, 2, 2, 3 ),
 ( 0.000000000000000000, 0.01388888888888888812, 0.02777777777777777624, 0.04166666666666666435, 0.05555555555555555247, 0.06944444444444444753, 0.08333333333333332871, 0.09722222222222223764, 0.1111111111111111049, 0.1250000000000000000, 0.1388888888888888951, 0.1527777777777777901, 0.1666666666666666574, 0.1805555555555555247, 0.1944444444444444753, 0.2083333333333333426, 0.2222222222222222099, 0.2361111111111111049, 0.2500000000000000000, 0.2638888888888888951, 0.2777777777777777901, 0.2916666666666666852, 0.3055555555555555802, 0.3194444444444444198, 0.3333333333333333148, 0.3472222222222222099, 0.3611111111111110494, 0.3750000000000000000, 0.3888888888888889506, 0.4027777777777777901, 0.4166666666666666852, 0.4305555555555555802, 0.4444444444444444198, 0.4583333333333333148, 0.4722222222222222099, 0.4861111111111110494, 0.5000000000000000000, 0.5138888888888888395, 0.5277777777777777901, 0.5416666666666666297, 0.5555555555555555802, 0.5694444444444444198, 0.5833333333333333703, 0.5972222222222222099, 0.6111111111111111605, 0.6250000000000001110, 0.6388888888888888395, 0.6527777777777777901, 0.6666666666666666297, 0.6805555555555555802, 0.6944444444444444198, 0.7083333333333333703, 0.7222222222222220989, 0.7361111111111111605, 0.7500000000000000000, 0.7638888888888888395, 0.7777777777777779011, 0.7916666666666666297, 0.8055555555555555802, 0.8194444444444444198, 0.8333333333333333703, 0.8472222222222222099, 0.8611111111111111605, 0.8749999999999998890, 0.8888888888888888395, 0.8895442836098168549 ),
 .UNSPECIFIED. ) 
 CURVE ( )  GEOMETRIC_REPRESENTATION_ITEM ( )  RATIONAL_B_SPLINE_CURVE ( ( 1.000000000000000000, 0.8660254037844387076, 1.000000000000000000, 0.8660254037844387076, 1.000000000000000000, 0.8660254037844387076, 1.000000000000000000, 0.8660254037844387076, 1.000000000000000000, 0.8660254037844387076, 1.000000000000000000, 0.8660254037844387076, 1.000000000000000000, 0.8660254037844387076, 1.000000000000000000, 0.8660254037844387076, 1.000000000000000000, 0.8660254037844387076, 1.000000000000000000, 0.8660254037844387076, 1.000000000000000000, 0.8660254037844387076, 1.000000000000000000, 0.8660254037844387076, 1.000000000000000000, 0.8660254037844387076, 1.000000000000000000, 0.8660254037844387076, 1.000000000000000000, 0.8660254037844387076, 1.000000000000000000, 0.8660254037844387076, 1.000000000000000000, 0.8660254037844387076, 1.000000000000000000, 0.8660254037844387076, 1.000000000000000000, 0.8660254037844387076, 1.000000000000000000, 0.8660254037844387076, 1.000000000000000000, 0.8660254037844387076, 1.000000000000000000, 0.8660254037844387076, 1.000000000000000000, 0.8660254037844387076, 1.000000000000000000, 0.8660254037844387076, 1.000000000000000000, 0.8660254037844387076, 1.000000000000000000, 0.8660254037844387076, 1.000000000000000000, 0.8660254037844387076, 1.000000000000000000, 0.8660254037844387076, 1.000000000000000000, 0.8660254037844387076, 1.000000000000000000, 0.8660254037844387076, 1.000000000000000000, 0.8660254037844387076, 1.000000000000000000, 0.8660254037844387076, 1.000000000000000000, 0.8660254037844387076, 1.000000000000000000, 0.8660254037844387076, 1.000000000000000000, 0.8660254037844387076, 1.000000000000000000, 0.8660254037844387076, 1.000000000000000000, 0.8660254037844387076, 1.000000000000000000, 0.8660254037844387076, 1.000000000000000000, 0.8660254037844387076, 1.000000000000000000, 0.8660254037844387076, 1.000000000000000000, 0.8660254037844387076, 1.000000000000000000, 0.8660254037844387076, 1.000000000000000000, 0.8660254037844387076, 1.000000000000000000, 0.8660254037844387076, 1.000000000000000000, 0.8660254037844387076, 1.000000000000000000, 0.8660254037844387076, 1.000000000000000000, 0.8660254037844387076, 1.000000000000000000, 0.8660254037844387076, 1.000000000000000000, 0.8660254037844387076, 1.000000000000000000, 0.8660254037844387076, 1.000000000000000000, 0.8660254037844387076, 1.000000000000000000, 0.8660254037844387076, 1.000000000000000000, 0.8660254037844387076, 1.000000000000000000, 0.8660254037844387076, 1.000000000000000000, 0.8660254037844387076, 1.000000000000000000, 0.8660254037844387076, 1.000000000000000000, 0.8660254037844387076, 1.000000000000000000, 0.8660254037844387076, 1.000000000000000000, 0.8660254037844387076, 1.000000000000000000, 0.8660254037844387076, 1.000000000000000000, 0.8660254037844387076, 1.000000000000000000, 0.8660254037844387076, 1.000000000000000000, 0.8660254037844387076, 1.000000000000000000, 0.8660254037844387076, 1.000000000000000000, 0.9936779504969338594, 0.9879525560471125178 ) ) 
 REPRESENTATION_ITEM ( '' )  );
#31843=CARTESIAN_POINT ( 'NONE',  ( 15.24356964374999990, 242.5468750006145058, 0.000000000000000000 ) ) ;
#31850=DIRECTION ( 'NONE',  ( -0.000000000000000000, 1.000000000000000000, -0.000000000000000000 ) ) ;
#31852=CARTESIAN_POINT ( 'NONE',  ( 0.6823418707358707147, 194.9999999999999716, 27.29152404244862495 ) ) ;
#31853=CARTESIAN_POINT ( 'NONE',  ( -27.00000000000000355, 196.9625000012290172, 0.000000000000000000 ) ) ;
#31858=CARTESIAN_POINT ( 'NONE',  ( 23.87821517812500005, 248.9968750006145228, 4.985214923628404016 ) ) ;
#31868=EDGE_CURVE ( 'NONE', #30804, #33968, #16995, .T. ) ;
#31870=CARTESIAN_POINT ( 'NONE',  ( 15.24356964375000167, 247.9843750006145058, 3.323476615752272600 ) ) ;
#31873=CARTESIAN_POINT ( 'NONE',  ( -22.74142690944354683, 194.9999999999999716, 14.88791141736823498 ) ) ;
#31891=CARTESIAN_POINT ( 'NONE',  ( -7.234628195640316228, 199.0075961894323200, -27.00000000000000000 ) ) ;
#31893=CARTESIAN_POINT ( 'NONE',  ( 27.00000000000001421, 197.4875000000000114, 15.58845726811988897 ) ) ;
#31895=CARTESIAN_POINT ( 'NONE',  ( 21.00000000000000000, 246.3718750006145228, 6.646953231504538984 ) ) ;
#31897=CARTESIAN_POINT ( 'NONE',  ( 26.75643035624999655, 240.1843750006145513, -7.049594010296217766E-16 ) ) ;
#31898=VERTEX_POINT ( 'NONE', #2946 ) ;
#31902=CARTESIAN_POINT ( 'NONE',  ( 26.99999999999999645, 245.7812500012290400, -7.347880794884117764E-16 ) ) ;
#31910=ORIENTED_EDGE ( 'NONE', *, *, #24664, .T. ) ;
#31915=CARTESIAN_POINT ( 'NONE',  ( 15.24356964374999990, 245.6593750006145171, -3.323476615752268604 ) ) ;
#31919=CARTESIAN_POINT ( 'NONE',  ( 7.405590309536301596, 215.0979036339257391, -3.170162721590327859 ) ) ;
#31929=EDGE_LOOP ( 'NONE', ( #11315, #3884, #2794, #3066, #1524, #485, #439, #691, #17196, #12341, #5379, #28594, #16396, #14208, #22229, #13170, #20276, #28093, #21765, #17621, #23480, #530, #19396, #29535, #15468, #6080, #14981, #32094, #7848, #5380, #18263, #32996, #11854, #10828, #34817, #29397, #22319, #20436, #26084, #21302, #5418, #23851, #7826, #12321, #14268, #5897, #35568, #16086 ) ) ;
#31933=CARTESIAN_POINT ( 'NONE',  ( 20.00041244883536606, 239.7473985345926053, -5.668978318349186196 ) ) ;
#31940=CARTESIAN_POINT ( 'NONE',  ( 26.99999999999999645, 241.3187500012290343, -3.464101615137755275 ) ) ;
#31942=CARTESIAN_POINT ( 'NONE',  ( -27.00000000000000355, 195.9125000000000796, -15.58845726811989429 ) ) ;
#31945=CARTESIAN_POINT ( 'NONE',  ( 26.75643035624999655, 246.9718750006145740, -3.323476615752271268 ) ) ;
#31953=CARTESIAN_POINT ( 'NONE',  ( 18.00000000000000355, 240.6250000000000000, 5.196152422706632912 ) ) ;
#31957=ORIENTED_EDGE ( 'NONE', *, *, #5683, .F. ) ;
#31961=CARTESIAN_POINT ( 'NONE',  ( -13.50000000000000533, 196.4375000012290400, -23.38268590217984411 ) ) ;
#31966=CARTESIAN_POINT ( 'NONE',  ( 24.00000000000000000, 249.2500000000000000, 5.196152422706629359 ) ) ;
#31967=CARTESIAN_POINT ( 'NONE',  ( 19.00081571707366379, 239.8729221881839635, -5.492723647597353320 ) ) ;
#31976=CYLINDRICAL_SURFACE ( 'NONE', #22796, 28.99999999999999645 ) ;
#31977=CARTESIAN_POINT ( 'NONE',  ( 27.24356964375000345, 196.0343750006145456, -3.336375036156643733E-15 ) ) ;
#31988=DIRECTION ( 'NONE',  ( -0.000000000000000000, 1.000000000000000000, -0.000000000000000000 ) ) ;
#31989=DIRECTION ( 'NONE',  ( 0.000000000000000000, 0.000000000000000000, -1.000000000000000000 ) ) ;
#31991=CARTESIAN_POINT ( 'NONE',  ( 3.253724281355069334E-15, 199.5500000012290513, -27.00000000000000000 ) ) ;
#31992=CARTESIAN_POINT ( 'NONE',  ( -26.99999999999999645, 195.0875000000000341, 15.58845726811991561 ) ) ;
#31996=DIRECTION ( 'NONE',  ( -0.000000000000000000, 1.000000000000000000, -0.000000000000000000 ) ) ;
#31999=CARTESIAN_POINT ( 'NONE',  ( 15.00000000000000178, 248.2375000000000114, 3.464101615137757051 ) ) ;
#32000=CARTESIAN_POINT ( 'NONE',  ( 27.24356964374999279, 199.6156250006145285, -15.72908226750539207 ) ) ;
#32004=EDGE_LOOP ( 'NONE', ( #26975, #7260, #28593, #6449 ) ) ;
#32005=CARTESIAN_POINT ( 'NONE',  ( 27.24356964374999635, 197.8156250006145171, -15.72908226750539029 ) ) ;
#32006=CARTESIAN_POINT ( 'NONE',  ( 18.12178482187500350, 242.6218750006145228, 4.985214923628407568 ) ) ;
#32009=CARTESIAN_POINT ( 'NONE',  ( 18.12178482187500350, 247.6843750006145228, 4.985214923628407568 ) ) ;
#32013=CARTESIAN_POINT ( 'NONE',  ( 23.87821517812499650, 242.8468750006145171, -4.985214923628404904 ) ) ;
#32020=DIRECTION ( 'NONE',  ( 0.000000000000000000, 0.000000000000000000, -1.000000000000000000 ) ) ;
#32023=LINE ( 'NONE', #5682, #14010 ) ;
#32027=EDGE_CURVE ( 'NONE', #8056, #2746, #19280, .T. ) ;
#32029=CARTESIAN_POINT ( 'NONE',  ( 26.75643035624999655, 242.7343750006145342, 3.323476615752267715 ) ) ;
#32036=CARTESIAN_POINT ( 'NONE',  ( 27.24356964375000345, 195.5843750006145285, -3.336375036156643733E-15 ) ) ;
#32038=DIRECTION ( 'NONE',  ( -0.000000000000000000, -0.000000000000000000, 1.000000000000000000 ) ) ;
#32042=ORIENTED_EDGE ( 'NONE', *, *, #9197, .T. ) ;
#32043=CARTESIAN_POINT ( 'NONE',  ( 26.99999999999999645, 239.8937500012290229, 3.464101615137751278 ) ) ;
#32058=CARTESIAN_POINT ( 'NONE',  ( 15.00000000000000000, 245.5187500012290513, -3.464101615137752610 ) ) ;
#32061=( BOUNDED_CURVE ( )  B_SPLINE_CURVE ( 2, ( #28579, #2617, #14193, #31799, #5645, #17415, #23099, #31617, #13640 ),
 .UNSPECIFIED., .F., .F. ) 
 B_SPLINE_CURVE_WITH_KNOTS ( ( 3, 2, 2, 2, 3 ),
 ( 0.01086956521739129711, 0.01449275362318840597, 0.02173913043478260809, 0.02898550724637681195, 0.03260869565217391908 ),
 .UNSPECIFIED. ) 
 CURVE ( )  GEOMETRIC_REPRESENTATION_ITEM ( )  RATIONAL_B_SPLINE_CURVE ( ( 0.9330127018922192983, 0.9330127018922191873, 1.000000000000000000, 0.8660254037844387076, 1.000000000000000000, 0.8660254037844387076, 1.000000000000000000, 0.9330127018922191873, 0.9330127018922192983 ) ) 
 REPRESENTATION_ITEM ( '' )  );
#32074=CARTESIAN_POINT ( 'NONE',  ( 15.00000000000000000, 242.3500000000000227, 0.000000000000000000 ) ) ;
#32078=DIRECTION ( 'NONE',  ( 0.000000000000000000, 1.000000000000000000, 0.000000000000000000 ) ) ;
#32079=FACE_OUTER_BOUND ( 'NONE', #1820, .T. ) ;
#32082=CARTESIAN_POINT ( 'NONE',  ( 21.00000000000000000, 244.7968750006145626, -6.646953231504538984 ) ) ;
#32084=DIRECTION ( 'NONE',  ( -0.000000000000000000, -1.000000000000000000, -0.000000000000000000 ) ) ;
#32087=CARTESIAN_POINT ( 'NONE',  ( 18.00000000000000000, 246.8312500012290513, -5.196152422706630247 ) ) ;
#32094=ORIENTED_EDGE ( 'NONE', *, *, #32992, .T. ) ;
#32099=CARTESIAN_POINT ( 'NONE',  ( 23.87821517812499650, 245.5468750006145058, -4.985214923628404904 ) ) ;
#32108=EDGE_CURVE ( 'NONE', #21071, #37055, #30420, .T. ) ;
#32121=ADVANCED_FACE ( 'NONE', ( #10135 ), #32688, .T. ) ;
#32127=CARTESIAN_POINT ( 'NONE',  ( -27.00000000000000355, 195.0500000000000114, 0.000000000000000000 ) ) ;
#32129=CARTESIAN_POINT ( 'NONE',  ( 18.12178482187500350, 246.3343750006145285, 4.985214923628407568 ) ) ;
#32132=CARTESIAN_POINT ( 'NONE',  ( 15.00000000000000000, 249.6062500012290570, 0.000000000000000000 ) ) ;
#32136=CARTESIAN_POINT ( 'NONE',  ( 21.00000000000000000, 241.3375000000000341, -6.928203230275506996 ) ) ;
#32137=CARTESIAN_POINT ( 'NONE',  ( -12.83063518929827751, 216.5618201379890309, 4.786185431830589643 ) ) ;
#32139=VERTEX_POINT ( 'NONE', #1034 ) ;
#32143=CARTESIAN_POINT ( 'NONE',  ( 15.00000000000000000, 248.2000000000000171, 0.000000000000000000 ) ) ;
#32149=VECTOR ( 'NONE', #3777, 1000.000000000000000 ) ;
#32157=CARTESIAN_POINT ( 'NONE',  ( 20.99999999999995381, 242.5187500012290513, 5.999999999999998224 ) ) ;
#32158=CARTESIAN_POINT ( 'NONE',  ( -27.24356964374999635, 195.8468750006145171, 15.72908226750539384 ) ) ;
#32171=AXIS2_PLACEMENT_3D ( 'NONE', #9397, #660, #34792 ) ;
#32189=CARTESIAN_POINT ( 'NONE',  ( 15.00000000000000000, 249.0999999999999943, 0.000000000000000000 ) ) ;
#32190=CARTESIAN_POINT ( 'NONE',  ( -27.24356964375000345, 195.3031250006145285, 0.000000000000000000 ) ) ;
#32193=ORIENTED_EDGE ( 'NONE', *, *, #32108, .F. ) ;
#32194=ORIENTED_EDGE ( 'NONE', *, *, #22111, .F. ) ;
#32195=CARTESIAN_POINT ( 'NONE',  ( 27.24356964375000700, 195.4906250006145001, 15.72908226750537075 ) ) ;
#32196=CARTESIAN_POINT ( 'NONE',  ( 21.00000000000000000, 242.6593750006145171, 6.646953231504538984 ) ) ;
#32199=CARTESIAN_POINT ( 'NONE',  ( 21.00000000000000000, 248.6218750006145228, 6.646953231504538984 ) ) ;
#32201=AXIS2_PLACEMENT_3D ( 'NONE', #2803, #20631, #8504 ) ;
#32205=CARTESIAN_POINT ( 'NONE',  ( 23.87821517812500005, 241.3468750006145171, 4.985214923628404016 ) ) ;
#32218=CARTESIAN_POINT ( 'NONE',  ( 26.99999999999999645, 199.0250000012290172, -15.58845726811990495 ) ) ;
#32221=CARTESIAN_POINT ( 'NONE',  ( 18.12178482187500350, 241.7218750006145171, 4.985214923628407568 ) ) ;
#32225=CARTESIAN_POINT ( 'NONE',  ( 26.99999999999999645, 241.7125000000000057, -3.464101615137755275 ) ) ;
#32228=CARTESIAN_POINT ( 'NONE',  ( -4.521054380870901390, 195.0000000000000853, 26.88021455572233620 ) ) ;
#32232=ORIENTED_EDGE ( 'NONE', *, *, #6847, .T. ) ;
#32233=CARTESIAN_POINT ( 'NONE',  ( 26.75643035624999655, 249.5593750006145228, -3.323476615752271712 ) ) ;
#32244=CARTESIAN_POINT ( 'NONE',  ( 26.75643035624999655, 249.0718750006145115, -7.049594010296217766E-16 ) ) ;
#32250=CARTESIAN_POINT ( 'NONE',  ( 26.99999999999999645, 248.0312500012290400, -7.347880794884117764E-16 ) ) ;
#32263=CARTESIAN_POINT ( 'NONE',  ( 27.00000000000000355, 195.8375000012290457, -3.306546357697854128E-15 ) ) ;
#32267=CARTESIAN_POINT ( 'NONE',  ( 15.24356964374999990, 244.9093750006145171, 0.000000000000000000 ) ) ;
#32272=CARTESIAN_POINT ( 'NONE',  ( 21.00000000000000000, 246.5687500012290343, 6.928203230275506996 ) ) ;
#32284=CARTESIAN_POINT ( 'NONE',  ( 18.12178482187499640, 247.4218750006145342, -4.985214923628404904 ) ) ;
#32287=EDGE_CURVE ( 'NONE', #6657, #11819, #10288, .T. ) ;
#32291=( NAMED_UNIT ( * ) SI_UNIT ( $, .STERADIAN. ) SOLID_ANGLE_UNIT ( ) );
#32306=( BOUNDED_CURVE ( )  B_SPLINE_CURVE ( 2, ( #2870, #23919, #17483, #29015, #21086, #20700, #34900, #15197, #3060, #11592, #18050, #6087, #14630, #32624, #29591, #9511, #6284, #14442, #32244, #17860, #8944, #6662, #29403, #15005, #23729, #20518, #23350, #26555, #26180, #17671, #29207, #26367, #3248, #584, #20891, #217, #32434, #6477, #11782, #18236, #26744, #25998, #27, #23168, #34710, #8756, #20329, #31870, #24845, #24659, #27691, #32811, #24480, #21461, #36026, #4192, #27318, #24108, #13104, #1530, #30548, #7605, #4377, #35652, #12728, #21274, #1720, #30354, #15955, #33569, #36210, #9881, #33002, #7053, #18621, #30163, #12542, #15767, #10253, #1345, #21829, #9697, #10069, #15574, #33383, #6852, #12917, #27508, #18810, #29971, #13289, #18428, #21641, #33194, #24296, #7422, #18992, #27130, #4001, #29780, #4565, #3810, #16141, #35839, #36396, #1156, #7236, #10442, #22016, #15388, #26936, #966, #8350, #25221, #34490, #5309, #7792, #33936, #19923, #30912, #19182, #33753, #19370, #37321, #16700, #13671, #31460, #4931, #27874, #34306, #22386, #16513, #11371, #5483, #28605, #22572, #30729, #25403, #36953, #36771, #22944, #10999, #34118, #28422, #10815, #2095, #13855, #28060, #7978, #19551, #5121, #31100, #4753, #28249, #16326, #25586, #8168, #19742, #17067, #2278, #1905, #31280, #16886, #25027, #25769, #2463, #14036, #2643, #14219, #37141, #10625, #13475, #36585, #11184, #22757, #22204, #3018, #28978, #3204, #20286, #14589, #23876, #26699, #20474, #32013, #31644, #26324, #6430, #2829, #26141, #8531, #35340, #31827, #28792, #12301, #5861, #18004, #6044, #29161, #23125, #23682, #23310, #14780, #11553, #3587, #3395, #29548, #34669, #360, #173, #11925, #17630, #23493, #14401, #29355, #17819, #9278, #35042, #5672, #730, #20658, #8715, #15149, #9089, #32205, #20097, #14964, #11741, #34856, #8897, #6241, #26512, #25958, #542, #12108, #35228, #20850, #17439, #32390, #17253, #26895, #925, #24250, #35985, #24436, #35608, #7377, #29733, #35794, #30120, #18379, #18766, #10021, #32769, #3767, #1677, #4332, #4151, #1299, #9837, #21414, #9652, #12495, #6804, #30502, #27650, #15912, #7196, #24619 ),
 .UNSPECIFIED., .F., .F. ) 
 B_SPLINE_CURVE_WITH_KNOTS ( ( 3, 2, 2, 2, 2, 2, 2, 2, 2, 2, 2, 2, 2, 2, 2, 2, 2, 2, 2, 2, 2, 2, 2, 2, 2, 2, 2, 2, 2, 2, 2, 2, 2, 2, 2, 2, 2, 2, 2, 2, 2, 2, 2, 2, 2, 2, 2, 2, 2, 2, 2, 2, 2, 2, 2, 2, 2, 2, 2, 2, 2, 2, 2, 2, 2, 2, 2, 2, 2, 2, 2, 2, 2, 2, 2, 2, 2, 2, 2, 2, 2, 2, 2, 2, 2, 2, 2, 2, 2, 2, 2, 2, 2, 2, 2, 2, 2, 2, 2, 2, 2, 2, 2, 2, 2, 2, 2, 2, 2, 2, 2, 2, 2, 2, 2, 2, 2, 2, 2, 2, 2, 2, 2, 2, 2, 2, 2, 2, 2, 2, 2, 2, 2, 2, 3 ),
 ( 0.000000000000000000, 0.007246376811594202987, 0.01449275362318840597, 0.02173913043478260809, 0.02898550724637681195, 0.03623188405797101580, 0.04347826086956521618, 0.05072463768115942351, 0.05797101449275362389, 0.06521739130434782428, 0.07246376811594203160, 0.07971014492753622505, 0.08695652173913043237, 0.09420289855072463969, 0.1014492753623188470, 0.1086956521739130405, 0.1159420289855072478, 0.1231884057971014551, 0.1304347826086956486, 0.1376811594202898559, 0.1449275362318840632, 0.1521739130434782705, 0.1594202898550724501, 0.1666666666666666574, 0.1739130434782608647, 0.1811594202898550721, 0.1884057971014492794, 0.1956521739130434867, 0.2028985507246376940, 0.2101449275362318736, 0.2173913043478260809, 0.2246376811594202882, 0.2318840579710144956, 0.2391304347826087029, 0.2463768115942029102, 0.2536231884057971175, 0.2608695652173912971, 0.2681159420289855322, 0.2753623188405797118, 0.2826086956521738913, 0.2898550724637681264, 0.2971014492753623615, 0.3043478260869565410, 0.3115942028985507206, 0.3188405797101449002, 0.3260869565217391353, 0.3333333333333333148, 0.3405797101449275499, 0.3478260869565217295, 0.3550724637681159646, 0.3623188405797101441, 0.3695652173913043237, 0.3768115942028985588, 0.3840579710144927383, 0.3913043478260869734, 0.3985507246376811530, 0.4057971014492753881, 0.4130434782608695676, 0.4202898550724637472, 0.4275362318840579823, 0.4347826086956521618, 0.4420289855072463969, 0.4492753623188405765, 0.4565217391304347561, 0.4637681159420289911, 0.4710144927536231707, 0.4782608695652174058, 0.4855072463768115854, 0.4927536231884058204, 0.5000000000000000000, 0.5072463768115942351, 0.5144927536231883591, 0.5217391304347825942, 0.5289855072463768293, 0.5362318840579710644, 0.5434782608695651884, 0.5507246376811594235, 0.5579710144927536586, 0.5652173913043477826, 0.5724637681159420177, 0.5797101449275362528, 0.5869565217391304879, 0.5942028985507247230, 0.6014492753623188470, 0.6086956521739130821, 0.6159420289855072062, 0.6231884057971014412, 0.6304347826086956763, 0.6376811594202898004, 0.6449275362318840354, 0.6521739130434782705, 0.6594202898550725056, 0.6666666666666666297, 0.6739130434782608647, 0.6811594202898550998, 0.6884057971014493349, 0.6956521739130434590, 0.7028985507246376940, 0.7101449275362319291, 0.7173913043478260532, 0.7246376811594202882, 0.7318840579710145233, 0.7391304347826086474, 0.7463768115942028825, 0.7536231884057971175, 0.7608695652173913526, 0.7681159420289854767, 0.7753623188405797118, 0.7826086956521739468, 0.7898550724637680709, 0.7971014492753623060, 0.8043478260869565410, 0.8115942028985507761, 0.8188405797101449002, 0.8260869565217391353, 0.8333333333333333703, 0.8405797101449274944, 0.8478260869565217295, 0.8550724637681159646, 0.8623188405797101996, 0.8695652173913043237, 0.8768115942028985588, 0.8840579710144927938, 0.8913043478260869179, 0.8985507246376811530, 0.9057971014492753881, 0.9130434782608695121, 0.9202898550724637472, 0.9275362318840579823, 0.9347826086956522174, 0.9420289855072463414, 0.9492753623188405765, 0.9565217391304348116, 0.9637681159420289356, 0.9662082966761270653 ),
 .UNSPECIFIED. ) 
 CURVE ( )  GEOMETRIC_REPRESENTATION_ITEM ( )  RATIONAL_B_SPLINE_CURVE ( ( 1.000000000000000000, 0.8660254037844387076, 1.000000000000000000, 0.8660254037844387076, 1.000000000000000000, 0.8660254037844387076, 1.000000000000000000, 0.8660254037844387076, 1.000000000000000000, 0.8660254037844387076, 1.000000000000000000, 0.8660254037844387076, 1.000000000000000000, 0.8660254037844387076, 1.000000000000000000, 0.8660254037844387076, 1.000000000000000000, 0.8660254037844387076, 1.000000000000000000, 0.8660254037844387076, 1.000000000000000000, 0.8660254037844387076, 1.000000000000000000, 0.8660254037844387076, 1.000000000000000000, 0.8660254037844387076, 1.000000000000000000, 0.8660254037844387076, 1.000000000000000000, 0.8660254037844387076, 1.000000000000000000, 0.8660254037844387076, 1.000000000000000000, 0.8660254037844387076, 1.000000000000000000, 0.8660254037844387076, 1.000000000000000000, 0.8660254037844387076, 1.000000000000000000, 0.8660254037844387076, 1.000000000000000000, 0.8660254037844387076, 1.000000000000000000, 0.8660254037844387076, 1.000000000000000000, 0.8660254037844387076, 1.000000000000000000, 0.8660254037844387076, 1.000000000000000000, 0.8660254037844387076, 1.000000000000000000, 0.8660254037844387076, 1.000000000000000000, 0.8660254037844387076, 1.000000000000000000, 0.8660254037844387076, 1.000000000000000000, 0.8660254037844387076, 1.000000000000000000, 0.8660254037844387076, 1.000000000000000000, 0.8660254037844387076, 1.000000000000000000, 0.8660254037844387076, 1.000000000000000000, 0.8660254037844387076, 1.000000000000000000, 0.8660254037844387076, 1.000000000000000000, 0.8660254037844387076, 1.000000000000000000, 0.8660254037844387076, 1.000000000000000000, 0.8660254037844387076, 1.000000000000000000, 0.8660254037844387076, 1.000000000000000000, 0.8660254037844387076, 1.000000000000000000, 0.8660254037844387076, 1.000000000000000000, 0.8660254037844387076, 1.000000000000000000, 0.8660254037844387076, 1.000000000000000000, 0.8660254037844387076, 1.000000000000000000, 0.8660254037844387076, 1.000000000000000000, 0.8660254037844387076, 1.000000000000000000, 0.8660254037844387076, 1.000000000000000000, 0.8660254037844387076, 1.000000000000000000, 0.8660254037844387076, 1.000000000000000000, 0.8660254037844387076, 1.000000000000000000, 0.8660254037844387076, 1.000000000000000000, 0.8660254037844387076, 1.000000000000000000, 0.8660254037844387076, 1.000000000000000000, 0.8660254037844387076, 1.000000000000000000, 0.8660254037844387076, 1.000000000000000000, 0.8660254037844387076, 1.000000000000000000, 0.8660254037844387076, 1.000000000000000000, 0.8660254037844387076, 1.000000000000000000, 0.8660254037844387076, 1.000000000000000000, 0.8660254037844387076, 1.000000000000000000, 0.8660254037844387076, 1.000000000000000000, 0.8660254037844387076, 1.000000000000000000, 0.8660254037844387076, 1.000000000000000000, 0.8660254037844387076, 1.000000000000000000, 0.8660254037844387076, 1.000000000000000000, 0.8660254037844387076, 1.000000000000000000, 0.8660254037844387076, 1.000000000000000000, 0.8660254037844387076, 1.000000000000000000, 0.8660254037844387076, 1.000000000000000000, 0.8660254037844387076, 1.000000000000000000, 0.8660254037844387076, 1.000000000000000000, 0.8660254037844387076, 1.000000000000000000, 0.8660254037844387076, 1.000000000000000000, 0.8660254037844387076, 1.000000000000000000, 0.8660254037844387076, 1.000000000000000000, 0.8660254037844387076, 1.000000000000000000, 0.8660254037844387076, 1.000000000000000000, 0.8660254037844387076, 1.000000000000000000, 0.8660254037844387076, 1.000000000000000000, 0.8660254037844387076, 1.000000000000000000, 0.8660254037844387076, 1.000000000000000000, 0.8660254037844387076, 1.000000000000000000, 0.8660254037844387076, 1.000000000000000000, 0.8660254037844387076, 1.000000000000000000, 0.8660254037844387076, 1.000000000000000000, 0.8660254037844387076, 1.000000000000000000, 0.8660254037844387076, 1.000000000000000000, 0.8660254037844387076, 1.000000000000000000, 0.8660254037844387076, 1.000000000000000000, 0.8660254037844387076, 1.000000000000000000, 0.8660254037844387076, 1.000000000000000000, 0.8660254037844387076, 1.000000000000000000, 0.8660254037844387076, 1.000000000000000000, 0.8660254037844387076, 1.000000000000000000, 0.8660254037844387076, 1.000000000000000000, 0.8660254037844387076, 1.000000000000000000, 0.8660254037844387076, 1.000000000000000000, 0.8660254037844387076, 1.000000000000000000, 0.8660254037844387076, 1.000000000000000000, 0.8660254037844387076, 1.000000000000000000, 0.8660254037844387076, 1.000000000000000000, 0.8660254037844387076, 1.000000000000000000, 0.8660254037844387076, 1.000000000000000000, 0.8660254037844387076, 1.000000000000000000, 0.8660254037844387076, 1.000000000000000000, 0.8660254037844387076, 1.000000000000000000, 0.8660254037844387076, 1.000000000000000000, 0.8660254037844387076, 1.000000000000000000, 0.8660254037844387076, 1.000000000000000000, 0.8660254037844387076, 1.000000000000000000, 0.8660254037844387076, 1.000000000000000000, 0.8660254037844387076, 1.000000000000000000, 0.8660254037844387076, 1.000000000000000000, 0.8660254037844387076, 1.000000000000000000, 0.8660254037844387076, 1.000000000000000000, 0.8660254037844387076, 1.000000000000000000, 0.8660254037844387076, 1.000000000000000000, 0.8660254037844387076, 1.000000000000000000, 0.8660254037844387076, 1.000000000000000000, 0.8660254037844387076, 1.000000000000000000, 0.8660254037844387076, 1.000000000000000000, 0.8660254037844387076, 1.000000000000000000, 0.8660254037844387076, 1.000000000000000000, 0.8660254037844387076, 1.000000000000000000, 0.8660254037844387076, 1.000000000000000000, 0.8660254037844387076, 1.000000000000000000, 0.8660254037844387076, 1.000000000000000000, 0.8660254037844387076, 1.000000000000000000, 0.8660254037844387076, 1.000000000000000000, 0.8660254037844387076, 1.000000000000000000, 0.8660254037844387076, 1.000000000000000000, 0.8660254037844387076, 1.000000000000000000, 0.8660254037844387076, 1.000000000000000000, 0.8660254037844387076, 1.000000000000000000, 0.9548847324609573972, 0.9401541411607521326 ) ) 
 REPRESENTATION_ITEM ( '' )  );
#32309=EDGE_CURVE ( 'NONE', #483, #30424, #20698, .T. ) ;
#32311=CARTESIAN_POINT ( 'NONE',  ( 0.000000000000000000, 210.0000000000000284, 0.000000000000000000 ) ) ;
#32317=CARTESIAN_POINT ( 'NONE',  ( 15.24356964374999990, 246.2593750006145399, 0.000000000000000000 ) ) ;
#32318=ORIENTED_EDGE ( 'NONE', *, *, #12017, .T. ) ;
#32323=AXIS2_PLACEMENT_3D ( 'NONE', #36486, #33467, #10530 ) ;
#32325=CARTESIAN_POINT ( 'NONE',  ( 15.00000000000000000, 240.5500000000000114, 0.000000000000000000 ) ) ;
#32327=VECTOR ( 'NONE', #21887, 1000.000000000000000 ) ;
#32333=CARTESIAN_POINT ( 'NONE',  ( 24.00000000000000000, 242.9499999999999886, 5.196152422706629359 ) ) ;
#32338=CARTESIAN_POINT ( 'NONE',  ( 23.87821517812500005, 241.0093750006145399, 4.985214923628404016 ) ) ;
#32343=ADVANCED_FACE ( 'NONE', ( #6544 ), #3971, .F. ) ;
#32348=CARTESIAN_POINT ( 'NONE',  ( -27.24356964375000345, 196.2593750006145399, 0.000000000000000000 ) ) ;
#32351=( BOUNDED_CURVE ( )  B_SPLINE_CURVE ( 2, ( #5139, #28814, #14423, #8738, #19942, #28998, #17090, #16720, #25424 ),
 .UNSPECIFIED., .F., .F. ) 
 B_SPLINE_CURVE_WITH_KNOTS ( ( 3, 2, 2, 2, 3 ),
 ( 0.6847826086956522174, 0.6884057971014492239, 0.6956521739130434590, 0.7028985507246376940, 0.7065217391304348116 ),
 .UNSPECIFIED. ) 
 CURVE ( )  GEOMETRIC_REPRESENTATION_ITEM ( )  RATIONAL_B_SPLINE_CURVE ( ( 0.9330127018922192983, 0.9330127018922202975, 1.000000000000000000, 0.8660254037844387076, 1.000000000000000000, 0.8660254037844387076, 1.000000000000000000, 0.9330127018922194093, 0.9330127018922194093 ) ) 
 REPRESENTATION_ITEM ( '' )  );
#32354=CARTESIAN_POINT ( 'NONE',  ( -29.00000000000002487, 222.9518338469886203, -12.50000000000000000 ) ) ;
#32362=CARTESIAN_POINT ( 'NONE',  ( 26.99999999999999645, 245.7249999999999943, -7.347880794884117764E-16 ) ) ;
#32364=CARTESIAN_POINT ( 'NONE',  ( 13.49999999999999645, 199.5125000012290286, -23.38268590217984766 ) ) ;
#32365=FACE_OUTER_BOUND ( 'NONE', #34383, .T. ) ;
#32374=CARTESIAN_POINT ( 'NONE',  ( 24.00000000000000000, 248.7999999999999829, 5.196152422706629359 ) ) ;
#32375=CARTESIAN_POINT ( 'NONE',  ( 5.778771075727756162E-15, 197.2156250006145513, 31.45816453501076637 ) ) ;
#32379=VERTEX_POINT ( 'NONE', #32698 ) ;
#32381=CARTESIAN_POINT ( 'NONE',  ( 5.778771075727756162E-15, 195.8656250006145285, 31.45816453501075927 ) ) ;
#32384=CARTESIAN_POINT ( 'NONE',  ( 18.12178482187499640, 246.6343750006145115, -4.985214923628404904 ) ) ;
#32390=CARTESIAN_POINT ( 'NONE',  ( 18.12178482187500350, 240.8218750006145399, 4.985214923628407568 ) ) ;
#32403=CARTESIAN_POINT ( 'NONE',  ( 13.49999999999999645, 198.5000000000000000, -23.38268590217984766 ) ) ;
#32408=CARTESIAN_POINT ( 'NONE',  ( 23.87821517812499650, 242.3968750006145285, -4.985214923628404904 ) ) ;
#32412=CARTESIAN_POINT ( 'NONE',  ( 13.62178482187501416, 199.1093750006145342, 23.59362340125806767 ) ) ;
#32420=CARTESIAN_POINT ( 'NONE',  ( 23.87821517812500005, 247.1968750006145115, 4.985214923628404016 ) ) ;
#32432=VECTOR ( 'NONE', #18403, 1000.000000000000000 ) ;
#32434=CARTESIAN_POINT ( 'NONE',  ( 15.24356964374999990, 248.3968750006145285, 0.000000000000000000 ) ) ;
#32440=CARTESIAN_POINT ( 'NONE',  ( -28.36931066777353294, 204.7133184642976005, 6.026954303579515226 ) ) ;
#32444=CARTESIAN_POINT ( 'NONE',  ( 19.39230484541324628, 246.3638461906613486, -5.999999999999989342 ) ) ;
#32448=LINE ( 'NONE', #15407, #26994 ) ;
#32457=AXIS2_PLACEMENT_3D ( 'NONE', #33870, #10375, #27625 ) ;
#32461=CARTESIAN_POINT ( 'NONE',  ( 26.99999999999999645, 246.1937500012290343, 3.464101615137751278 ) ) ;
#32464=CARTESIAN_POINT ( 'NONE',  ( 18.00000000000000000, 246.7750000000000057, -5.196152422706630247 ) ) ;
#32469=ORIENTED_EDGE ( 'NONE', *, *, #2301, .F. ) ;
#32471=CARTESIAN_POINT ( 'NONE',  ( 26.75643035624999655, 246.3718750006145228, -7.049594010296217766E-16 ) ) ;
#32500=CARTESIAN_POINT ( 'NONE',  ( 26.75643035624999655, 247.3468750006145171, 3.323476615752267271 ) ) ;
#32507=( BOUNDED_CURVE ( )  B_SPLINE_CURVE ( 2, ( #935, #29941, #32403, #15163, #24262, #23695, #29367, #29746, #3968 ),
 .UNSPECIFIED., .F., .T. ) 
 B_SPLINE_CURVE_WITH_KNOTS ( ( 3, 2, 2, 2, 3 ),
 ( 0.2708333333333333703, 0.2777777777777777901, 0.2916666666666666852, 0.3055555555555555802, 0.3125000000000000000 ),
 .UNSPECIFIED. ) 
 CURVE ( )  GEOMETRIC_REPRESENTATION_ITEM ( )  RATIONAL_B_SPLINE_CURVE ( ( 0.9330127018922194093, 0.9330127018922196314, 1.000000000000000000, 0.8660254037844387076, 1.000000000000000000, 0.8660254037844387076, 1.000000000000000000, 0.9330127018922194093, 0.9330127018922194093 ) ) 
 REPRESENTATION_ITEM ( '' )  );
#32508=CARTESIAN_POINT ( 'NONE',  ( 26.99999999999999645, 240.7749999999999773, -7.347880794884117764E-16 ) ) ;
#32511=ORIENTED_EDGE ( 'NONE', *, *, #2301, .T. ) ;
#32512=VERTEX_POINT ( 'NONE', #35541 ) ;
#32513=CARTESIAN_POINT ( 'NONE',  ( 13.50000000000001421, 196.6625000012290343, 23.38268590217984055 ) ) ;
#32516=CARTESIAN_POINT ( 'NONE',  ( 21.00000000000000000, 249.0437500012290570, -5.999999999999998224 ) ) ;
#32525=CARTESIAN_POINT ( 'NONE',  ( 21.00000000000000000, 245.6125000000000114, 5.999999999999998224 ) ) ;
#32530=ADVANCED_FACE ( 'NONE', ( #21160 ), #21536, .F. ) ;
#32534=CARTESIAN_POINT ( 'NONE',  ( 27.24356964375000345, 198.2281250006145399, -3.336375036156643733E-15 ) ) ;
#32545=CARTESIAN_POINT ( 'NONE',  ( 20.99999999999999645, 185.0294372515228645, -5.999999999999999112 ) ) ;
#32546=CARTESIAN_POINT ( 'NONE',  ( 24.00000000000000000, 244.7500000000000000, 5.196152422706629359 ) ) ;
#32548=CARTESIAN_POINT ( 'NONE',  ( 27.00000000000001421, 199.4000000012290457, 15.58845726811988897 ) ) ;
#32549=CARTESIAN_POINT ( 'NONE',  ( -26.99999999999999645, 195.2000000012290286, 15.58845726811991561 ) ) ;
#32554=CARTESIAN_POINT ( 'NONE',  ( 1.069080835302379631E-14, 198.4250000012290229, 27.00000000000000000 ) ) ;
#32558=CARTESIAN_POINT ( 'NONE',  ( 3.306546357697853733E-15, 210.0000000000000284, 27.00000000000000000 ) ) ;
#32559=CARTESIAN_POINT ( 'NONE',  ( 15.00000000000000000, 248.6500000000000057, 0.000000000000000000 ) ) ;
#32560=CARTESIAN_POINT ( 'NONE',  ( -27.24356964375000345, 197.0656250006145171, -15.72908226750537786 ) ) ;
#32563=VECTOR ( 'NONE', #32078, 1000.000000000000000 ) ;
#32565=CARTESIAN_POINT ( 'NONE',  ( -13.62178482187500528, 195.2281250006145399, -23.59362340125807123 ) ) ;
#32566=DIRECTION ( 'NONE',  ( 0.000000000000000000, 0.000000000000000000, 1.000000000000000000 ) ) ;
#32570=CARTESIAN_POINT ( 'NONE',  ( 21.00000000000000000, 247.4968750006145513, -6.646953231504538984 ) ) ;
#32577=CARTESIAN_POINT ( 'NONE',  ( -27.24356964374999990, 199.8218750006145399, -15.72908226750537786 ) ) ;
#32589=CARTESIAN_POINT ( 'NONE',  ( 22.60769515458673240, 248.3325961894322518, 6.000000000000000000 ) ) ;
#32593=CYLINDRICAL_SURFACE ( 'NONE', #23737, 5.999999999999999112 ) ;
#32596=CARTESIAN_POINT ( 'NONE',  ( 21.00000000000000000, 241.7593750006145115, 6.646953231504538984 ) ) ;
#32601=CARTESIAN_POINT ( 'NONE',  ( -27.24356964375000345, 199.8593750006145342, 0.000000000000000000 ) ) ;
#32602=DIRECTION ( 'NONE',  ( 0.1736605105622160139, 0.000000000000000000, 0.9848055783103945027 ) ) ;
#32608=CIRCLE ( 'NONE', #34421, 17.99999999999998934 ) ;
#32611=CARTESIAN_POINT ( 'NONE',  ( 15.24356964375000167, 247.0843750006145285, 3.323476615752272600 ) ) ;
#32616=DIRECTION ( 'NONE',  ( 0.000000000000000000, -0.000000000000000000, -1.000000000000000000 ) ) ;
#32617=EDGE_LOOP ( 'NONE', ( #29344, #5474, #24162, #17270 ) ) ;
#32624=CARTESIAN_POINT ( 'NONE',  ( 15.24356964374999990, 249.2593750006145115, -3.323476615752268604 ) ) ;
#32626=CARTESIAN_POINT ( 'NONE',  ( 1.069080835302379631E-14, 199.3250000012290286, 27.00000000000000000 ) ) ;
#32628=CARTESIAN_POINT ( 'NONE',  ( 0.000000000000000000, 202.0000000000000000, 0.000000000000000000 ) ) ;
#32631=CARTESIAN_POINT ( 'NONE',  ( -28.09635861911301546, 206.4454563690075588, 7.185930831749626435 ) ) ;
#32647=CARTESIAN_POINT ( 'NONE',  ( 20.99999999999998579, 248.5374999999999659, -5.999999999999997335 ) ) ;
#32648=CARTESIAN_POINT ( 'NONE',  ( 0.000000000000000000, 210.0000000000000284, -27.00000000000000000 ) ) ;
#32650=CYLINDRICAL_SURFACE ( 'NONE', #7583, 27.00000000000000000 ) ;
#32651=ORIENTED_EDGE ( 'NONE', *, *, #21739, .F. ) ;
#32652=CARTESIAN_POINT ( 'NONE',  ( 24.00000000000000000, 243.0062500012290627, 5.196152422706629359 ) ) ;
#32662=CARTESIAN_POINT ( 'NONE',  ( 15.24356964374999990, 243.8593750006145342, -3.323476615752268604 ) ) ;
#32675=AXIS2_PLACEMENT_3D ( 'NONE', #8590, #5548, #25834 ) ;
#32676=CARTESIAN_POINT ( 'NONE',  ( 26.99999999999999645, 240.7749999999999773, -7.347880794884117764E-16 ) ) ;
#32684=DIRECTION ( 'NONE',  ( 0.000000000000000000, 0.000000000000000000, 1.000000000000000000 ) ) ;
#32688=CYLINDRICAL_SURFACE ( 'NONE', #1431, 8.000000000000000000 ) ;
#32690=CARTESIAN_POINT ( 'NONE',  ( 15.24356964374999990, 247.6093750006145342, 0.000000000000000000 ) ) ;
#32694=CARTESIAN_POINT ( 'NONE',  ( 18.00000000000000355, 245.1812500012290457, 5.196152422706632912 ) ) ;
#32698=CARTESIAN_POINT ( 'NONE',  ( 1.069080835302379631E-14, 195.2750000012290457, 27.00000000000000000 ) ) ;
#32703=ORIENTED_EDGE ( 'NONE', *, *, #14005, .T. ) ;
#32704=CARTESIAN_POINT ( 'NONE',  ( 20.99999999999999645, 185.0294372515228645, 0.000000000000000000 ) ) ;
#32706=CARTESIAN_POINT ( 'NONE',  ( 26.99999999999999645, 246.6625000000000227, -3.464101615137755275 ) ) ;
#32713=CARTESIAN_POINT ( 'NONE',  ( 21.00000000000000000, 243.8687500012290172, 5.999999999999998224 ) ) ;
#32715=CARTESIAN_POINT ( 'NONE',  ( 20.99999999999997513, 245.3875000000000455, -5.999999999999999112 ) ) ;
#32719=EDGE_CURVE ( 'NONE', #5744, #8565, #11074, .T. ) ;
#32724=CARTESIAN_POINT ( 'NONE',  ( -13.62178482187500528, 198.3781250006145171, -23.59362340125807123 ) ) ;
#32729=CARTESIAN_POINT ( 'NONE',  ( 19.39230484541324984, 244.7486538117967143, 5.999999999999991118 ) ) ;
#32730=DIRECTION ( 'NONE',  ( -1.000000000000000000, -0.000000000000000000, -0.000000000000000000 ) ) ;
#32737=CARTESIAN_POINT ( 'NONE',  ( 18.00000000000000000, 240.5312500012290400, -5.196152422706630247 ) ) ;
#32742=DIRECTION ( 'NONE',  ( 1.000000000000000000, 0.000000000000000000, -0.000000000000000000 ) ) ;
#32750=CARTESIAN_POINT ( 'NONE',  ( 26.99999999999999645, 247.0374999999999943, 3.464101615137751278 ) ) ;
#32751=CARTESIAN_POINT ( 'NONE',  ( 5.778771075727756162E-15, 196.3156250006145171, 31.45816453501076637 ) ) ;
#32756=EDGE_LOOP ( 'NONE', ( #5700, #31957, #52, #8935 ) ) ;
#32757=CARTESIAN_POINT ( 'NONE',  ( -13.50000000000000533, 199.5875000012290457, -23.38268590217984411 ) ) ;
#32758=CARTESIAN_POINT ( 'NONE',  ( 18.12178482187500350, 239.9218750006145058, 4.985214923628407568 ) ) ;
#32761=CARTESIAN_POINT ( 'NONE',  ( 23.87821517812499650, 245.6593750006145171, -4.985214923628404904 ) ) ;
#32764=CARTESIAN_POINT ( 'NONE',  ( 20.99999999999999289, 243.1937500012290343, -5.999999999999997335 ) ) ;
#32767=EDGE_CURVE ( 'NONE', #17657, #32139, #11724, .T. ) ;
#32769=CARTESIAN_POINT ( 'NONE',  ( 15.24356964374999990, 240.2593750006144830, -3.323476615752268604 ) ) ;
#32784=APPLICATION_CONTEXT ( 'automotive_design' ) ;
#32786=CARTESIAN_POINT ( 'NONE',  ( 23.87821517812499650, 240.1468750006145285, -4.985214923628404904 ) ) ;
#32787=ORIENTED_EDGE ( 'NONE', *, *, #17824, .T. ) ;
#32791=CARTESIAN_POINT ( 'NONE',  ( 26.99999999999999645, 242.6125000000000114, -3.464101615137755275 ) ) ;
#32792=CARTESIAN_POINT ( 'NONE',  ( 20.99999999999999645, 185.0294372515228645, 5.999999999999999112 ) ) ;
#32797=VERTEX_POINT ( 'NONE', #28693 ) ;
#32799=CARTESIAN_POINT ( 'NONE',  ( 26.75643035624999655, 247.3093750006144944, -3.323476615752271712 ) ) ;
#32811=CARTESIAN_POINT ( 'NONE',  ( 20.99999999999999645, 247.8343750006144717, -6.646953231504538984 ) ) ;
#32812=LINE ( 'NONE', #23921, #6724 ) ;
#32817=CARTESIAN_POINT ( 'NONE',  ( 20.99999999999998579, 248.1437500012290229, -5.999999999999997335 ) ) ;
#32832=CARTESIAN_POINT ( 'NONE',  ( -26.99999999999998934, 195.5374999999999943, 15.58845726811991561 ) ) ;
#32837=FACE_OUTER_BOUND ( 'NONE', #36687, .T. ) ;
#32839=CARTESIAN_POINT ( 'NONE',  ( 21.00000000000000000, 242.9687500012290684, 6.928203230275506996 ) ) ;
#32847=CARTESIAN_POINT ( 'NONE',  ( 23.87821517812499650, 244.1968750006145115, -4.985214923628404904 ) ) ;
#32849=VECTOR ( 'NONE', #33740, 1000.000000000000000 ) ;
#32858=ADVANCED_FACE ( 'NONE', ( #14304 ), #21923, .F. ) ;
#32859=( BOUNDED_CURVE ( )  B_SPLINE_CURVE ( 2, ( #6560, #27026, #12054, #23626, #32143, #18135, #18517, #18322, #29489 ),
 .UNSPECIFIED., .F., .F. ) 
 B_SPLINE_CURVE_WITH_KNOTS ( ( 3, 2, 2, 2, 3 ),
 ( 0.1630434782608695676, 0.1666666666666666574, 0.1739130434782608647, 0.1811594202898550721, 0.1847826086956521618 ),
 .UNSPECIFIED. ) 
 CURVE ( )  GEOMETRIC_REPRESENTATION_ITEM ( )  RATIONAL_B_SPLINE_CURVE ( ( 0.9330127018922194093, 0.9330127018922196314, 1.000000000000000000, 0.8660254037844387076, 1.000000000000000000, 0.8660254037844387076, 1.000000000000000000, 0.9330127018922196314, 0.9330127018922194093 ) ) 
 REPRESENTATION_ITEM ( '' )  );
#32870=CARTESIAN_POINT ( 'NONE',  ( 20.99999999999999645, 185.0294372515228645, 0.000000000000000000 ) ) ;
#32881=CARTESIAN_POINT ( 'NONE',  ( 20.99999999999999645, 244.1218750006145228, 6.646953231504538984 ) ) ;
#32882=ORIENTED_EDGE ( 'NONE', *, *, #34481, .T. ) ;
#32891=VERTEX_POINT ( 'NONE', #12249 ) ;
#32895=CARTESIAN_POINT ( 'NONE',  ( 22.60769515458673595, 249.4736538117967370, -6.000000000000001776 ) ) ;
#32901=CARTESIAN_POINT ( 'NONE',  ( 10.42677199038629787, 213.9649605036052833, 4.520320870633288912 ) ) ;
#32910=CARTESIAN_POINT ( 'NONE',  ( -13.62178482187498396, 198.0781250006145342, 23.59362340125808188 ) ) ;
#32915=CARTESIAN_POINT ( 'NONE',  ( 19.39230484541326049, 244.5638461906613657, -5.999999999999997335 ) ) ;
#32930=CARTESIAN_POINT ( 'NONE',  ( 27.00000000000001421, 199.2874999999999943, 15.58845726811988897 ) ) ;
#32937=CARTESIAN_POINT ( 'NONE',  ( 21.00000000000000000, 246.9624999999999773, 6.928203230275506996 ) ) ;
#32938=CARTESIAN_POINT ( 'NONE',  ( -27.24356964374999279, 197.1406250006145342, 15.72908226750539384 ) ) ;
#32943=CARTESIAN_POINT ( 'NONE',  ( -13.62178482187498396, 196.2781250006145228, 23.59362340125808188 ) ) ;
#32944=CYLINDRICAL_SURFACE ( 'NONE', #2317, 5.999999999999999112 ) ;
#32947=CARTESIAN_POINT ( 'NONE',  ( 15.24356964375000167, 245.3968750006145285, 3.323476615752272600 ) ) ;
#32949=VECTOR ( 'NONE', #34968, 1000.000000000000000 ) ;
#32951=CARTESIAN_POINT ( 'NONE',  ( 22.60769515458672885, 242.9888461906614054, 5.999999999999997335 ) ) ;
#32956=DIRECTION ( 'NONE',  ( 0.000000000000000000, 1.000000000000000000, 0.000000000000000000 ) ) ;
#32962=DIRECTION ( 'NONE',  ( 0.000000000000000000, 1.000000000000000000, 0.000000000000000000 ) ) ;
#32969=CARTESIAN_POINT ( 'NONE',  ( 3.306546357697853733E-15, 210.0000000000000284, 27.00000000000000000 ) ) ;
#32972=CARTESIAN_POINT ( 'NONE',  ( 18.12178482187499640, 239.7718750006145001, -4.985214923628404904 ) ) ;
#32976=CARTESIAN_POINT ( 'NONE',  ( 13.62178482187501416, 199.5593750006145513, 23.59362340125806767 ) ) ;
#32980=CARTESIAN_POINT ( 'NONE',  ( 15.24356964374999990, 243.9718750006145456, -3.323476615752268604 ) ) ;
#32985=VERTEX_POINT ( 'NONE', #37455 ) ;
#32987=CARTESIAN_POINT ( 'NONE',  ( 18.12178482187500350, 246.6718750006145342, 4.985214923628407568 ) ) ;
#32992=EDGE_CURVE ( 'NONE', #529, #23005, #33534, .T. ) ;
#32996=ORIENTED_EDGE ( 'NONE', *, *, #28836, .T. ) ;
#33002=CARTESIAN_POINT ( 'NONE',  ( 15.24356964374999990, 247.0468750006145058, 0.000000000000000000 ) ) ;
#33014=CARTESIAN_POINT ( 'NONE',  ( 15.00000000000000000, 241.4499999999999886, 0.000000000000000000 ) ) ;
#33017=ORIENTED_EDGE ( 'NONE', *, *, #36583, .T. ) ;
#33020=( BOUNDED_CURVE ( )  B_SPLINE_CURVE ( 2, ( #26337, #29369, #11939, #32218, #19606, #23697, #25274, #23508, #3408 ),
 .UNSPECIFIED., .F., .F. ) 
 B_SPLINE_CURVE_WITH_KNOTS ( ( 3, 2, 2, 2, 3 ),
 ( 0.1041666666666666713, 0.1111111111111111049, 0.1250000000000000000, 0.1388888888888888951, 0.1458333333333333426 ),
 .UNSPECIFIED. ) 
 CURVE ( )  GEOMETRIC_REPRESENTATION_ITEM ( )  RATIONAL_B_SPLINE_CURVE ( ( 0.9330127018922194093, 0.9330127018922194093, 1.000000000000000000, 0.8660254037844387076, 1.000000000000000000, 0.8660254037844387076, 1.000000000000000000, 0.9330127018922194093, 0.9330127018922194093 ) ) 
 REPRESENTATION_ITEM ( '' )  );
#33025=CARTESIAN_POINT ( 'NONE',  ( -1.909035429704832693E-15, 195.3874999999999886, -31.17691453623979214 ) ) ;
#33032=CARTESIAN_POINT ( 'NONE',  ( 15.00000000000000000, 242.8187500012290627, -3.464101615137752166 ) ) ;
#33034=ADVANCED_FACE ( 'NONE', ( #10344 ), #30879, .T. ) ;
#33042=CYLINDRICAL_SURFACE ( 'NONE', #1980, 27.00000000000000000 ) ;
#33043=CARTESIAN_POINT ( 'NONE',  ( 23.87821517812500005, 244.9468750006145115, 4.985214923628404016 ) ) ;
#33073=CARTESIAN_POINT ( 'NONE',  ( 26.75643035624999655, 249.1468750006145285, 3.323476615752267715 ) ) ;
#33075=CARTESIAN_POINT ( 'NONE',  ( 26.75643035624999655, 244.1968750006145683, 3.323476615752267271 ) ) ;
#33077=FACE_BOUND ( 'NONE', #20552, .T. ) ;
#33084=ORIENTED_EDGE ( 'NONE', *, *, #8768, .F. ) ;
#33088=CARTESIAN_POINT ( 'NONE',  ( -7.234628195640263826, 195.8575961894323711, -27.00000000000003553 ) ) ;
#33090=LINE ( 'NONE', #18707, #17815 ) ;
#33098=DIRECTION ( 'NONE',  ( -0.000000000000000000, -1.000000000000000000, -0.000000000000000000 ) ) ;
#33104=CARTESIAN_POINT ( 'NONE',  ( -27.24356964374999635, 197.5906250006145228, 15.72908226750539384 ) ) ;
#33110=CARTESIAN_POINT ( 'NONE',  ( 3.306546357697853733E-15, 210.0000000000000284, 27.00000000000000000 ) ) ;
#33129=DIRECTION ( 'NONE',  ( -0.000000000000000000, 1.000000000000000000, -0.000000000000000000 ) ) ;
#33132=CARTESIAN_POINT ( 'NONE',  ( 21.00000000000000000, 245.6124999999999829, 6.928203230275506996 ) ) ;
#33139=PRODUCT_DEFINITION ( 'UNKNOWN', '', #25670, #5807 ) ;
#33140=CARTESIAN_POINT ( 'NONE',  ( 13.50000000000001421, 198.9125000012290343, 23.38268590217984055 ) ) ;
#33145=CARTESIAN_POINT ( 'NONE',  ( 21.00000000000000000, 244.5718750006145115, 6.646953231504538984 ) ) ;
#33151=FACE_OUTER_BOUND ( 'NONE', #13419, .T. ) ;
#33160=CARTESIAN_POINT ( 'NONE',  ( -27.00000000000000355, 199.6250000012290400, -15.58845726811989429 ) ) ;
#33165=CARTESIAN_POINT ( 'NONE',  ( 23.87821517812500005, 240.4468750006145115, 4.985214923628404016 ) ) ;
#33166=ORIENTED_EDGE ( 'NONE', *, *, #14594, .T. ) ;
#33174=CARTESIAN_POINT ( 'NONE',  ( 15.24356964375000167, 241.7968750006145342, 3.323476615752272600 ) ) ;
#33180=CARTESIAN_POINT ( 'NONE',  ( 21.00000000000000000, 248.0593750006145228, 6.646953231504538984 ) ) ;
#33188=ORIENTED_EDGE ( 'NONE', *, *, #18627, .F. ) ;
#33194=CARTESIAN_POINT ( 'NONE',  ( 20.99999999999999645, 246.2593750006145115, 6.646953231504538984 ) ) ;
#33196=CARTESIAN_POINT ( 'NONE',  ( 26.99999999999999645, 196.6625000000000512, -15.58845726811990495 ) ) ;
#33198=CARTESIAN_POINT ( 'NONE',  ( 20.99999999999999289, 245.8374999999999773, -5.999999999999997335 ) ) ;
#33206=CARTESIAN_POINT ( 'NONE',  ( 18.00000000000000355, 241.5249999999999773, 5.196152422706632912 ) ) ;
#33209=VERTEX_POINT ( 'NONE', #20238 ) ;
#33216=CARTESIAN_POINT ( 'NONE',  ( -27.24356964374999990, 197.5718750006145399, -15.72908226750537786 ) ) ;
#33221=EDGE_LOOP ( 'NONE', ( #5928, #15960, #6918, #3464, #2036, #12953 ) ) ;
#33222=CARTESIAN_POINT ( 'NONE',  ( 26.99999999999999645, 244.4687500012290684, -3.464101615137755275 ) ) ;
#33225=CARTESIAN_POINT ( 'NONE',  ( 15.00000000000000178, 242.8375000000000057, 3.464101615137757051 ) ) ;
#33231=CARTESIAN_POINT ( 'NONE',  ( 21.00000000000000000, 245.1343750006145115, -6.646953231504538984 ) ) ;
#33244=DIRECTION ( 'NONE',  ( 0.000000000000000000, 1.000000000000000000, 0.000000000000000000 ) ) ;
#33253=DIRECTION ( 'NONE',  ( -0.000000000000000000, -1.000000000000000000, -0.000000000000000000 ) ) ;
#33254=CARTESIAN_POINT ( 'NONE',  ( -26.99999999999999645, 199.1375000000000171, 15.58845726811991561 ) ) ;
#33258=CARTESIAN_POINT ( 'NONE',  ( 20.99999999999999645, 185.0294372515228645, -5.999999999999999112 ) ) ;
#33260=CARTESIAN_POINT ( 'NONE',  ( 20.99999999999999645, 243.8968750006145285, -6.646953231504538984 ) ) ;
#33262=CARTESIAN_POINT ( 'NONE',  ( 18.00000000000000000, 249.5312500012290684, -5.196152422706630247 ) ) ;
#33272=ORIENTED_EDGE ( 'NONE', *, *, #27886, .T. ) ;
#33274=CARTESIAN_POINT ( 'NONE',  ( 20.99999999999999645, 250.0000000000000000, 0.000000000000000000 ) ) ;
#33282=EDGE_CURVE ( 'NONE', #149, #21332, #8850, .T. ) ;
#33283=CARTESIAN_POINT ( 'NONE',  ( 21.00000000000000000, 210.0000000000000000, 5.999999999999996447 ) ) ;
#33291=CARTESIAN_POINT ( 'NONE',  ( -27.24356964375000345, 199.3531250006145399, 0.000000000000000000 ) ) ;
#33294=EDGE_CURVE ( 'NONE', #33538, #14209, #31124, .T. ) ;
#33295=ORIENTED_EDGE ( 'NONE', *, *, #36699, .F. ) ;
#33296=( BOUNDED_CURVE ( )  B_SPLINE_CURVE ( 2, ( #3743, #29333, #15509, #9628, #3369, #15316, #26869, #6781, #18356 ),
 .UNSPECIFIED., .F., .F. ) 
 B_SPLINE_CURVE_WITH_KNOTS ( ( 3, 2, 2, 2, 3 ),
 ( 0.4456521739130434590, 0.4492753623188405765, 0.4565217391304347561, 0.4637681159420289911, 0.4673913043478261087 ),
 .UNSPECIFIED. ) 
 CURVE ( )  GEOMETRIC_REPRESENTATION_ITEM ( )  RATIONAL_B_SPLINE_CURVE ( ( 0.9330127018922191873, 0.9330127018922187432, 1.000000000000000000, 0.8660254037844387076, 1.000000000000000000, 0.8660254037844387076, 1.000000000000000000, 0.9330127018922188542, 0.9330127018922194093 ) ) 
 REPRESENTATION_ITEM ( '' )  );
#33310=CARTESIAN_POINT ( 'NONE',  ( 5.727106289114498080E-15, 199.2125000000000057, 31.17691453623979214 ) ) ;
#33319=CARTESIAN_POINT ( 'NONE',  ( 26.99999999999999645, 244.8625000000000114, -3.464101615137755275 ) ) ;
#33321=( BOUNDED_CURVE ( )  B_SPLINE_CURVE ( 2, ( #28221, #5095, #22176, #2249, #11160, #13828, #8325, #2066, #31254 ),
 .UNSPECIFIED., .F., .F. ) 
 B_SPLINE_CURVE_WITH_KNOTS ( ( 3, 2, 2, 2, 3 ),
 ( 0.09782608695652174335, 0.1014492753623188470, 0.1086956521739130405, 0.1159420289855072478, 0.1195652173913043653 ),
 .UNSPECIFIED. ) 
 CURVE ( )  GEOMETRIC_REPRESENTATION_ITEM ( )  RATIONAL_B_SPLINE_CURVE ( ( 0.9330127018922194093, 0.9330127018922194093, 1.000000000000000000, 0.8660254037844387076, 1.000000000000000000, 0.8660254037844387076, 1.000000000000000000, 0.9330127018922190762, 0.9330127018922194093 ) ) 
 REPRESENTATION_ITEM ( '' )  );
#33326=CARTESIAN_POINT ( 'NONE',  ( 26.99999999999999645, 197.6750000012290513, -15.58845726811990495 ) ) ;
#33330=CARTESIAN_POINT ( 'NONE',  ( 15.24356964374999990, 244.8718750006145513, -3.323476615752268604 ) ) ;
#33340=EDGE_CURVE ( 'NONE', #36194, #30424, #22447, .T. ) ;
#33343=ADVANCED_FACE ( 'NONE', ( #4993 ), #28485, .F. ) ;
#33354=CARTESIAN_POINT ( 'NONE',  ( 21.00000000000000000, 249.7468750006145797, -6.646953231504538984 ) ) ;
#33359=CARTESIAN_POINT ( 'NONE',  ( -27.24356964375000345, 197.6093750006145342, 0.000000000000000000 ) ) ;
#33362=CARTESIAN_POINT ( 'NONE',  ( 21.00000000000000000, 242.3218750006145115, 6.646953231504538984 ) ) ;
#33367=CARTESIAN_POINT ( 'NONE',  ( 21.00000000000000000, 243.5593750006145228, 6.646953231504538984 ) ) ;
#33379=MANIFOLD_SOLID_BREP ( 'Thread1', #19303 ) ;
#33383=CARTESIAN_POINT ( 'NONE',  ( 15.24356964374999990, 246.5968750006145171, 0.000000000000000000 ) ) ;
#33396=ORIENTED_EDGE ( 'NONE', *, *, #2504, .T. ) ;
#33402=CARTESIAN_POINT ( 'NONE',  ( -27.24356964374999990, 198.0218750006145569, -15.72908226750537786 ) ) ;
#33403=CARTESIAN_POINT ( 'NONE',  ( -14.50000000000000000, 215.7563705986615901, 5.555555555555558023 ) ) ;
#33404=CARTESIAN_POINT ( 'NONE',  ( 22.60769515458672885, 243.8325961894323086, 5.999999999999997335 ) ) ;
#33408=CARTESIAN_POINT ( 'NONE',  ( 15.00000000000000000, 243.7562500012290627, 0.000000000000000000 ) ) ;
#33411=FACE_OUTER_BOUND ( 'NONE', #17838, .T. ) ;
#33427=CARTESIAN_POINT ( 'NONE',  ( 27.00000000000000355, 199.7750000000000057, -3.306546357697854128E-15 ) ) ;
#33437=DIRECTION ( 'NONE',  ( 0.000000000000000000, 0.000000000000000000, -1.000000000000000000 ) ) ;
#33438=FACE_OUTER_BOUND ( 'NONE', #25479, .T. ) ;
#33440=CARTESIAN_POINT ( 'NONE',  ( 15.24356964374999990, 247.1593750006145171, 0.000000000000000000 ) ) ;
#33442=CARTESIAN_POINT ( 'NONE',  ( 20.99999999999999645, 245.0218750006145285, 6.646953231504538984 ) ) ;
#33451=EDGE_CURVE ( 'NONE', #19674, #32379, #16610, .T. ) ;
#33452=EDGE_LOOP ( 'NONE', ( #24595, #2659, #1001, #15773 ) ) ;
#33463=CARTESIAN_POINT ( 'NONE',  ( -26.99999999999999645, 197.3375000000000057, 15.58845726811991561 ) ) ;
#33465=CARTESIAN_POINT ( 'NONE',  ( 18.00000000000000000, 243.6812500012290457, -5.196152422706630247 ) ) ;
#33467=DIRECTION ( 'NONE',  ( -0.000000000000000000, 1.000000000000000000, -0.000000000000000000 ) ) ;
#33473=CARTESIAN_POINT ( 'NONE',  ( -13.62178482187500528, 196.5781250006145342, -23.59362340125807123 ) ) ;
#33481=CARTESIAN_POINT ( 'NONE',  ( 15.24356964374999990, 249.8593750006145342, 0.000000000000000000 ) ) ;
#33495=LINE ( 'NONE', #21950, #6435 ) ;
#33498=STYLED_ITEM ( 'NONE', ( #12582 ), #21035 ) ;
#33501=CARTESIAN_POINT ( 'NONE',  ( 21.00000000000000000, 246.5125000000000171, 6.928203230275506996 ) ) ;
#33502=CARTESIAN_POINT ( 'NONE',  ( 10.49999999999999467, 222.9518338469886203, -12.50000000000000000 ) ) ;
#33505=ORIENTED_EDGE ( 'NONE', *, *, #1699, .T. ) ;
#33507=CARTESIAN_POINT ( 'NONE',  ( -26.99999999999998934, 197.4500000012290570, 15.58845726811991561 ) ) ;
#33508=CARTESIAN_POINT ( 'NONE',  ( -13.49999999999998401, 196.9250000000000114, 23.38268590217985476 ) ) ;
#33509=EDGE_CURVE ( 'NONE', #20600, #21259, #28218, .T. ) ;
#33512=CARTESIAN_POINT ( 'NONE',  ( 18.12178482187499640, 245.2843750006145456, -4.985214923628404904 ) ) ;
#33520=CARTESIAN_POINT ( 'NONE',  ( -13.62178482187500528, 198.4343750006145228, -23.59362340125807123 ) ) ;
#33525=DIRECTION ( 'NONE',  ( -0.000000000000000000, -1.000000000000000000, -0.000000000000000000 ) ) ;
#33533=EDGE_CURVE ( 'NONE', #33538, #10561, #29423, .T. ) ;
#33534=( BOUNDED_CURVE ( )  B_SPLINE_CURVE ( 2, ( #32713, #15287, #9969, #1243, #4279, #21732, #33465, #1433, #24011 ),
 .UNSPECIFIED., .F., .F. ) 
 B_SPLINE_CURVE_WITH_KNOTS ( ( 3, 2, 2, 2, 3 ),
 ( 0.5543478260869565410, 0.5579710144927536586, 0.5652173913043477826, 0.5724637681159420177, 0.5760869565217391353 ),
 .UNSPECIFIED. ) 
 CURVE ( )  GEOMETRIC_REPRESENTATION_ITEM ( )  RATIONAL_B_SPLINE_CURVE ( ( 0.9330127018922194093, 0.9330127018922194093, 1.000000000000000000, 0.8660254037844387076, 1.000000000000000000, 0.8660254037844387076, 1.000000000000000000, 0.9330127018922194093, 0.9330127018922194093 ) ) 
 REPRESENTATION_ITEM ( '' )  );
#33537=CARTESIAN_POINT ( 'NONE',  ( 26.75643035624999655, 249.5968750006145171, 3.323476615752267715 ) ) ;
#33538=VERTEX_POINT ( 'NONE', #17313 ) ;
#33541=CARTESIAN_POINT ( 'NONE',  ( 13.62178482187501416, 197.3093750006145513, 23.59362340125806767 ) ) ;
#33543=CARTESIAN_POINT ( 'NONE',  ( 19.39230484541326760, 239.7986538117967257, 5.999999999999999112 ) ) ;
#33544=CARTESIAN_POINT ( 'NONE',  ( 21.00000000000000000, 244.1218750006145513, 6.646953231504538984 ) ) ;
#33545=FACE_OUTER_BOUND ( 'NONE', #16675, .T. ) ;
#33548=ORIENTED_EDGE ( 'NONE', *, *, #27085, .F. ) ;
#33552=CARTESIAN_POINT ( 'NONE',  ( 26.75643035624999655, 245.0218750006145001, -7.049594010296217766E-16 ) ) ;
#33554=EDGE_CURVE ( 'NONE', #21332, #8445, #34733, .T. ) ;
#33561=EDGE_CURVE ( 'NONE', #25530, #11819, #8777, .T. ) ;
#33569=CARTESIAN_POINT ( 'NONE',  ( 20.99999999999999645, 247.1593750006145171, 6.646953231504538984 ) ) ;
#33577=CARTESIAN_POINT ( 'NONE',  ( 15.00000000000000000, 244.6000000000000227, 0.000000000000000000 ) ) ;
#33583=CARTESIAN_POINT ( 'NONE',  ( 21.00000000000000000, 210.0000000000000284, 8.000000000000000000 ) ) ;
#33588=CARTESIAN_POINT ( 'NONE',  ( -27.24356964375000345, 198.0593750006145513, 0.000000000000000000 ) ) ;
#33590=CARTESIAN_POINT ( 'NONE',  ( 12.48663586349064403, 194.9999999999999716, 24.21355016816918493 ) ) ;
#33595=CARTESIAN_POINT ( 'NONE',  ( 26.99999999999999645, 241.2437500012290457, 3.464101615137751278 ) ) ;
#33598=CARTESIAN_POINT ( 'NONE',  ( 27.24356964375000345, 198.2281250006145399, -3.336375036156643733E-15 ) ) ;
#33602=VERTEX_POINT ( 'NONE', #35105 ) ;
#33614=CARTESIAN_POINT ( 'NONE',  ( -8.147294799025798895, 219.8188806670532358, -2.997157372947703458 ) ) ;
#33617=CARTESIAN_POINT ( 'NONE',  ( 20.99999999999997868, 216.0000000000000000, 7.347880794884120722E-16 ) ) ;
#33621=CARTESIAN_POINT ( 'NONE',  ( -28.92641906063026269, 202.2706296558042993, -2.079858847736485661 ) ) ;
#33627=CARTESIAN_POINT ( 'NONE',  ( 26.99999999999999645, 247.4875000000000682, 3.464101615137751278 ) ) ;
#33632=CARTESIAN_POINT ( 'NONE',  ( 18.12178482187500350, 246.7843750006145456, 4.985214923628407568 ) ) ;
#33634=CARTESIAN_POINT ( 'NONE',  ( 18.12178482187500350, 243.1843750006145513, 4.985214923628407568 ) ) ;
#33636=CARTESIAN_POINT ( 'NONE',  ( 15.00000000000000178, 249.1937500012290627, 3.464101615137757051 ) ) ;
#33649=CARTESIAN_POINT ( 'NONE',  ( 23.87821517812499650, 249.5968750006145171, -4.985214923628404904 ) ) ;
#33653=CARTESIAN_POINT ( 'NONE',  ( 15.04813726045348155, 225.8716339721264319, -0.7835069059937238567 ) ) ;
#33655=CARTESIAN_POINT ( 'NONE',  ( 26.99999999999999645, 197.1125000000000114, -15.58845726811990495 ) ) ;
#33661=CARTESIAN_POINT ( 'NONE',  ( 27.24356964375000345, 195.0781250006145342, -3.336375036156643733E-15 ) ) ;
#33675=CARTESIAN_POINT ( 'NONE',  ( 15.00000000000000178, 246.4375000000000000, 3.464101615137757051 ) ) ;
#33683=CARTESIAN_POINT ( 'NONE',  ( 18.00000000000000355, 241.9749999999999943, 5.196152422706632912 ) ) ;
#33688=CARTESIAN_POINT ( 'NONE',  ( 26.99999999999999645, 243.4375000000000000, 3.464101615137751278 ) ) ;
#33695=ORIENTED_EDGE ( 'NONE', *, *, #18060, .T. ) ;
#33696=CARTESIAN_POINT ( 'NONE',  ( 26.99999999999999645, 199.0250000012290457, -15.58845726811990495 ) ) ;
#33697=CYLINDRICAL_SURFACE ( 'NONE', #11406, 5.999999999999999112 ) ;
#33701=CARTESIAN_POINT ( 'NONE',  ( 26.75643035624999655, 242.8468750006145456, 3.323476615752267715 ) ) ;
#33706=CARTESIAN_POINT ( 'NONE',  ( 13.62178482187499640, 198.3593750006145342, -23.59362340125807123 ) ) ;
#33714=VECTOR ( 'NONE', #3687, 1000.000000000000000 ) ;
#33726=CIRCLE ( 'NONE', #30705, 5.999999999999999112 ) ;
#33727=CARTESIAN_POINT ( 'NONE',  ( -27.24356964374999279, 197.6468750006145285, 15.72908226750539384 ) ) ;
#33732=CARTESIAN_POINT ( 'NONE',  ( 15.24356964374999990, 242.1718750006145342, -3.323476615752268604 ) ) ;
#33738=CARTESIAN_POINT ( 'NONE',  ( 18.12178482187499640, 244.2718750006145001, -4.985214923628404904 ) ) ;
#33740=DIRECTION ( 'NONE',  ( -0.000000000000000000, -1.000000000000000000, -0.000000000000000000 ) ) ;
#33744=CARTESIAN_POINT ( 'NONE',  ( 21.00000000000000000, 244.2624999999999886, 5.999999999999998224 ) ) ;
#33747=ORIENTED_EDGE ( 'NONE', *, *, #37101, .T. ) ;
#33753=CARTESIAN_POINT ( 'NONE',  ( 15.24356964374999990, 245.2093750006145285, -3.323476615752268604 ) ) ;
#33754=CARTESIAN_POINT ( 'NONE',  ( -7.234628195640328663, 197.5049038117967086, 26.99999999999999289 ) ) ;
#33759=( BOUNDED_CURVE ( )  B_SPLINE_CURVE ( 2, ( #36745, #25745, #19714, #16486, #20073, #25193, #31072, #8142, #5280 ),
 .UNSPECIFIED., .F., .F. ) 
 B_SPLINE_CURVE_WITH_KNOTS ( ( 3, 2, 2, 2, 3 ),
 ( 0.8804347826086956763, 0.8840579710144927938, 0.8913043478260869179, 0.8985507246376811530, 0.9021739130434782705 ),
 .UNSPECIFIED. ) 
 CURVE ( )  GEOMETRIC_REPRESENTATION_ITEM ( )  RATIONAL_B_SPLINE_CURVE ( ( 0.9330127018922194093, 0.9330127018922194093, 1.000000000000000000, 0.8660254037844387076, 1.000000000000000000, 0.8660254037844387076, 1.000000000000000000, 0.9330127018922194093, 0.9330127018922194093 ) ) 
 REPRESENTATION_ITEM ( '' )  );
#33765=CARTESIAN_POINT ( 'NONE',  ( 26.99999999999999645, 242.6312500012290343, -7.347880794884117764E-16 ) ) ;
#33771=CARTESIAN_POINT ( 'NONE',  ( 20.99999999999999645, 185.0294372515228645, 0.000000000000000000 ) ) ;
#33774=CARTESIAN_POINT ( 'NONE',  ( 19.39230484541327471, 246.9986538117966859, 6.000000000000002665 ) ) ;
#33775=CARTESIAN_POINT ( 'NONE',  ( 13.62178482187499640, 197.9093750006145456, -23.59362340125807123 ) ) ;
#33777=CARTESIAN_POINT ( 'NONE',  ( 23.99999999999999645, 244.0000000000000000, -5.196152422706631135 ) ) ;
#33782=CARTESIAN_POINT ( 'NONE',  ( 26.99999999999999645, 242.5937500012290400, 3.464101615137751278 ) ) ;
#33785=CARTESIAN_POINT ( 'NONE',  ( 13.62178482187499640, 197.8531250006145399, -23.59362340125807123 ) ) ;
#33789=CIRCLE ( 'NONE', #35594, 8.000000000000000000 ) ;
#33794=( BOUNDED_CURVE ( )  B_SPLINE_CURVE ( 2, ( #11613, #23000, #26018, #20537, #35288, #31893, #29037, #23371, #26201 ),
 .UNSPECIFIED., .F., .F. ) 
 B_SPLINE_CURVE_WITH_KNOTS ( ( 3, 2, 2, 2, 3 ),
 ( 0.4375000000000000000, 0.4444444444444444198, 0.4583333333333333148, 0.4722222222222222099, 0.4791666666666666852 ),
 .UNSPECIFIED. ) 
 CURVE ( )  GEOMETRIC_REPRESENTATION_ITEM ( )  RATIONAL_B_SPLINE_CURVE ( ( 0.9330127018922194093, 0.9330127018922194093, 1.000000000000000000, 0.8660254037844387076, 1.000000000000000000, 0.8660254037844387076, 1.000000000000000000, 0.9330127018922190762, 0.9330127018922194093 ) ) 
 REPRESENTATION_ITEM ( '' )  );
#33802=LINE ( 'NONE', #4424, #7704 ) ;
#33810=CARTESIAN_POINT ( 'NONE',  ( -27.87471972953270338, 209.4684846313719788, -8.000000000000003553 ) ) ;
#33811=ORIENTED_EDGE ( 'NONE', *, *, #23727, .F. ) ;
#33816=DIRECTION ( 'NONE',  ( 0.000000000000000000, 1.000000000000000000, 0.000000000000000000 ) ) ;
#33819=CARTESIAN_POINT ( 'NONE',  ( 26.75643035624999655, 248.2843750006145456, -7.049594010296217766E-16 ) ) ;
#33821=CARTESIAN_POINT ( 'NONE',  ( 20.99999999999999645, 241.1968750006145399, -6.646953231504538984 ) ) ;
#33825=CARTESIAN_POINT ( 'NONE',  ( 26.99999999999999645, 247.9937500012290457, 3.464101615137751278 ) ) ;
#33839=CARTESIAN_POINT ( 'NONE',  ( 21.00000000000000000, 248.5093750006144830, 6.646953231504538984 ) ) ;
#33842=CARTESIAN_POINT ( 'NONE',  ( 14.68278727570712761, 216.3172127243002478, -0.6964482669459951536 ) ) ;
#33849=CARTESIAN_POINT ( 'NONE',  ( 27.24356964374999635, 197.3656250006145285, -15.72908226750539029 ) ) ;
#33856=CARTESIAN_POINT ( 'NONE',  ( 20.99999999999997868, 245.6687500012290855, 5.999999999999999112 ) ) ;
#33864=EDGE_CURVE ( 'NONE', #33538, #33209, #7200, .T. ) ;
#33866=CARTESIAN_POINT ( 'NONE',  ( -1.909035429704832693E-15, 196.7374999999999829, -31.17691453623979214 ) ) ;
#33870=CARTESIAN_POINT ( 'NONE',  ( 0.000000000000000000, 210.0000000000000284, 0.000000000000000000 ) ) ;
#33877=CARTESIAN_POINT ( 'NONE',  ( 23.99999999999999645, 244.0000000000000000, -5.196152422706631135 ) ) ;
#33883=CARTESIAN_POINT ( 'NONE',  ( -13.50000000000000533, 199.1375000012290286, -23.38268590217984411 ) ) ;
#33887=CARTESIAN_POINT ( 'NONE',  ( 15.24356964374999990, 242.2093750006145285, 0.000000000000000000 ) ) ;
#33893=CARTESIAN_POINT ( 'NONE',  ( -13.62178482187500528, 199.3343750006145569, -23.59362340125807123 ) ) ;
#33905=CARTESIAN_POINT ( 'NONE',  ( 1.120210788295102201E-13, 196.8500000012290343, -27.00000000000000711 ) ) ;
#33907=CARTESIAN_POINT ( 'NONE',  ( -14.50000000000000000, 210.0000000000000000, 0.000000000000000000 ) ) ;
#33908=DIRECTION ( 'NONE',  ( -0.000000000000000000, -1.000000000000000000, -0.000000000000000000 ) ) ;
#33912=CARTESIAN_POINT ( 'NONE',  ( 27.24356964375000700, 197.3468750006145740, 15.72908226750537075 ) ) ;
#33916=CARTESIAN_POINT ( 'NONE',  ( 15.24356964375000167, 240.8968750006145001, 3.323476615752272600 ) ) ;
#33923=CARTESIAN_POINT ( 'NONE',  ( 18.12178482187500350, 243.9718750006145171, 4.985214923628407568 ) ) ;
#33927=CARTESIAN_POINT ( 'NONE',  ( 22.60769515458672885, 244.4674038105676743, -5.999999999999998224 ) ) ;
#33936=CARTESIAN_POINT ( 'NONE',  ( 20.99999999999999645, 245.3593750006145342, 6.646953231504538984 ) ) ;
#33945=EDGE_CURVE ( 'NONE', #27888, #13079, #33789, .T. ) ;
#33946=CARTESIAN_POINT ( 'NONE',  ( 20.99999999999995381, 242.5187500012290513, 5.999999999999998224 ) ) ;
#33954=( BOUNDED_CURVE ( )  B_SPLINE_CURVE ( 2, ( #15958, #9884, #30734, #6857, #7056, #27321, #4569, #27512, #33198 ),
 .UNSPECIFIED., .F., .F. ) 
 B_SPLINE_CURVE_WITH_KNOTS ( ( 3, 2, 2, 2, 3 ),
 ( 0.3804347826086956763, 0.3840579710144927383, 0.3913043478260869734, 0.3985507246376811530, 0.4021739130434782705 ),
 .UNSPECIFIED. ) 
 CURVE ( )  GEOMETRIC_REPRESENTATION_ITEM ( )  RATIONAL_B_SPLINE_CURVE ( ( 0.9330127018922194093, 0.9330127018922198534, 1.000000000000000000, 0.8660254037844387076, 1.000000000000000000, 0.8660254037844387076, 1.000000000000000000, 0.9330127018922194093, 0.9330127018922194093 ) ) 
 REPRESENTATION_ITEM ( '' )  );
#33956=CARTESIAN_POINT ( 'NONE',  ( -27.24356964374999990, 197.1218750006145228, -15.72908226750537786 ) ) ;
#33962=CARTESIAN_POINT ( 'NONE',  ( 24.00000000000000000, 240.7562500012290627, 5.196152422706629359 ) ) ;
#33968=VERTEX_POINT ( 'NONE', #33403 ) ;
#33989=ORIENTED_EDGE ( 'NONE', *, *, #20704, .F. ) ;
#33996=CARTESIAN_POINT ( 'NONE',  ( 15.00000000000000000, 247.7500000000000000, 0.000000000000000000 ) ) ;
#33997=CARTESIAN_POINT ( 'NONE',  ( 18.12178482187499640, 248.8843750006145399, -4.985214923628404904 ) ) ;
#33999=CARTESIAN_POINT ( 'NONE',  ( 26.75643035624999655, 242.0218750006145285, -3.323476615752271268 ) ) ;
#34000=ORIENTED_EDGE ( 'NONE', *, *, #4553, .T. ) ;
#34001=FACE_OUTER_BOUND ( 'NONE', #18120, .T. ) ;
#34003=CARTESIAN_POINT ( 'NONE',  ( 15.00000000000000000, 247.8062500012290457, 0.000000000000000000 ) ) ;
#34011=ORIENTED_EDGE ( 'NONE', *, *, #21970, .T. ) ;
#34015=( BOUNDED_CURVE ( )  B_SPLINE_CURVE ( 2, ( #24546, #9207, #32694, #30234, #18503, #29476, #6549, #30042, #17932 ),
 .UNSPECIFIED., .F., .F. ) 
 B_SPLINE_CURVE_WITH_KNOTS ( ( 3, 2, 2, 2, 3 ),
 ( 0.4239130434782608647, 0.4275362318840579823, 0.4347826086956521618, 0.4420289855072463969, 0.4456521739130434590 ),
 .UNSPECIFIED. ) 
 CURVE ( )  GEOMETRIC_REPRESENTATION_ITEM ( )  RATIONAL_B_SPLINE_CURVE ( ( 0.9330127018922194093, 0.9330127018922194093, 1.000000000000000000, 0.8660254037844387076, 1.000000000000000000, 0.8660254037844387076, 1.000000000000000000, 0.9330127018922198534, 0.9330127018922191873 ) ) 
 REPRESENTATION_ITEM ( '' )  );
#34017=CARTESIAN_POINT ( 'NONE',  ( 15.24356964375000167, 247.9843750006145058, 3.323476615752272600 ) ) ;
#34022=CARTESIAN_POINT ( 'NONE',  ( 14.14550961275246621, 216.8544903872546286, -0.3345106846829432046 ) ) ;
#34029=EDGE_CURVE ( 'NONE', #15992, #8565, #36185, .T. ) ;
#34032=CARTESIAN_POINT ( 'NONE',  ( -27.24356964375000345, 197.1031250006145399, 0.000000000000000000 ) ) ;
#34036=CARTESIAN_POINT ( 'NONE',  ( 26.99999999999999645, 248.8937500012290513, 3.464101615137751278 ) ) ;
#34049=CARTESIAN_POINT ( 'NONE',  ( -27.00000000000000355, 197.3000000000000114, 0.000000000000000000 ) ) ;
#34053=CARTESIAN_POINT ( 'NONE',  ( 23.87821517812500005, 249.1093750006145342, 4.985214923628404016 ) ) ;
#34060=CARTESIAN_POINT ( 'NONE',  ( 21.00000000000000000, 243.3625000000000398, 6.928203230275506996 ) ) ;
#34065=CARTESIAN_POINT ( 'NONE',  ( 27.00000000000000355, 194.9375000012290400, -3.306546357697854128E-15 ) ) ;
#34066=CARTESIAN_POINT ( 'NONE',  ( -7.234628195640302017, 196.9424038105676971, 27.00000000000000711 ) ) ;
#34069=CARTESIAN_POINT ( 'NONE',  ( 18.12178482187499640, 243.0343750006145456, -4.985214923628404904 ) ) ;
#34076=CARTESIAN_POINT ( 'NONE',  ( -1.926257025242585782E-15, 198.8468750006145740, -31.45816453501075927 ) ) ;
#34079=LINE ( 'NONE', #8131, #18362 ) ;
#34080=( BOUNDED_CURVE ( )  B_SPLINE_CURVE ( 2, ( #13084, #33543, #30889, #36753, #24638, #10979, #10794, #7217, #36189 ),
 .UNSPECIFIED., .F., .F. ) 
 B_SPLINE_CURVE_WITH_KNOTS ( ( 3, 2, 2, 2, 3 ),
 ( 0.9456521739130434590, 0.9492753623188405765, 0.9565217391304348116, 0.9637681159420289356, 0.9662082966761270653 ),
 .UNSPECIFIED. ) 
 CURVE ( )  GEOMETRIC_REPRESENTATION_ITEM ( )  RATIONAL_B_SPLINE_CURVE ( ( 0.9330127018922194093, 0.9330127018922194093, 1.000000000000000000, 0.8660254037844387076, 1.000000000000000000, 0.8660254037844387076, 1.000000000000000000, 0.9548847324609573972, 0.9401541411607521326 ) ) 
 REPRESENTATION_ITEM ( '' )  );
#34081=CARTESIAN_POINT ( 'NONE',  ( 15.00000000000000178, 247.3374999999999773, 3.464101615137757051 ) ) ;
#34083=FACE_OUTER_BOUND ( 'NONE', #577, .T. ) ;
#34086=CARTESIAN_POINT ( 'NONE',  ( 23.99999999999999645, 247.2062500012290229, -5.196152422706631135 ) ) ;
#34091=CARTESIAN_POINT ( 'NONE',  ( 26.99999999999999645, 248.8750000000000000, -7.347880794884117764E-16 ) ) ;
#34092=LINE ( 'NONE', #16674, #431 ) ;
#34096=CARTESIAN_POINT ( 'NONE',  ( 13.62178482187499640, 197.0093750006145399, -23.59362340125807123 ) ) ;
#34100=CARTESIAN_POINT ( 'NONE',  ( 23.87821517812500005, 241.4593750006145285, 4.985214923628404016 ) ) ;
#34105=CARTESIAN_POINT ( 'NONE',  ( 23.87821517812499650, 243.7468750006145228, -4.985214923628404904 ) ) ;
#34116=AXIS2_PLACEMENT_3D ( 'NONE', #704, #6404, #29138 ) ;
#34118=CARTESIAN_POINT ( 'NONE',  ( 18.12178482187500350, 244.4218750006145058, 4.985214923628407568 ) ) ;
#34119=CARTESIAN_POINT ( 'NONE',  ( 26.99999999999999645, 240.3625000000000114, -3.464101615137755275 ) ) ;
#34140=CARTESIAN_POINT ( 'NONE',  ( 19.39230484541324628, 246.8138461906613372, -5.999999999999989342 ) ) ;
#34141=CARTESIAN_POINT ( 'NONE',  ( 13.62178482187501416, 195.0593750006145513, 23.59362340125806767 ) ) ;
#34147=CARTESIAN_POINT ( 'NONE',  ( 26.99999999999999645, 242.6687500012290570, -3.464101615137755275 ) ) ;
#34156=CARTESIAN_POINT ( 'NONE',  ( 21.00000000000000000, 246.1187500012290457, 5.999999999999998224 ) ) ;
#34163=CARTESIAN_POINT ( 'NONE',  ( -9.014689842941500331, 195.0000000000000000, 25.72782777481439709 ) ) ;
#34172=( BOUNDED_CURVE ( )  B_SPLINE_CURVE ( 2, ( #35439, #9487, #4170, #32791, #7030, #24455, #6640, #944, #24082 ),
 .UNSPECIFIED., .F., .F. ) 
 B_SPLINE_CURVE_WITH_KNOTS ( ( 3, 2, 2, 2, 3 ),
 ( 0.7065217391304348116, 0.7101449275362319291, 0.7173913043478260532, 0.7246376811594202882, 0.7282608695652174058 ),
 .UNSPECIFIED. ) 
 CURVE ( )  GEOMETRIC_REPRESENTATION_ITEM ( )  RATIONAL_B_SPLINE_CURVE ( ( 0.9330127018922194093, 0.9330127018922194093, 1.000000000000000000, 0.8660254037844387076, 1.000000000000000000, 0.8660254037844387076, 1.000000000000000000, 0.9330127018922194093, 0.9330127018922194093 ) ) 
 REPRESENTATION_ITEM ( '' )  );
#34176=CARTESIAN_POINT ( 'NONE',  ( 15.00000000000000000, 247.8062500012290457, 0.000000000000000000 ) ) ;
#34177=ORIENTED_EDGE ( 'NONE', *, *, #29538, .F. ) ;
#34185=CARTESIAN_POINT ( 'NONE',  ( 15.24356964374999990, 248.9218750006145058, -3.323476615752268604 ) ) ;
#34187=CARTESIAN_POINT ( 'NONE',  ( 23.87821517812499650, 242.0593750006145228, -4.985214923628404904 ) ) ;
#34190=CARTESIAN_POINT ( 'NONE',  ( 18.00000000000000000, 248.1812500012290457, -5.196152422706630247 ) ) ;
#34195=CARTESIAN_POINT ( 'NONE',  ( 21.00000000000000000, 240.7187500012290400, 5.999999999999998224 ) ) ;
#34200=EDGE_LOOP ( 'NONE', ( #28046, #6764, #30040, #19445, #17300, #20275, #7642, #6227 ) ) ;
#34205=CARTESIAN_POINT ( 'NONE',  ( 26.75643035624999655, 248.6218750006145228, -7.049594010296217766E-16 ) ) ;
#34206=EDGE_CURVE ( 'NONE', #20737, #8598, #23774, .T. ) ;
#34209=CARTESIAN_POINT ( 'NONE',  ( 15.31535524866699483, 225.1590526702200634, -1.929602858955059341 ) ) ;
#34217=CARTESIAN_POINT ( 'NONE',  ( 13.62178482187501416, 197.2531250006145456, 23.59362340125806767 ) ) ;
#34235=CARTESIAN_POINT ( 'NONE',  ( 27.00000000000000355, 198.8750000000000284, -3.306546357697854128E-15 ) ) ;
#34236=CARTESIAN_POINT ( 'NONE',  ( 20.99999999999999645, 185.0294372515228645, 0.000000000000000000 ) ) ;
#34239=CARTESIAN_POINT ( 'NONE',  ( 20.99999999999999645, 249.0718750006145399, 6.646953231504538984 ) ) ;
#34240=ORIENTED_EDGE ( 'NONE', *, *, #35989, .F. ) ;
#34247=CARTESIAN_POINT ( 'NONE',  ( 15.00000000000000000, 243.2125000000000057, -3.464101615137752166 ) ) ;
#34252=CARTESIAN_POINT ( 'NONE',  ( -13.49999999999998401, 197.0375000012290627, 23.38268590217985476 ) ) ;
#34257=CARTESIAN_POINT ( 'NONE',  ( 15.24356964374999990, 241.7218750006145171, -3.323476615752268604 ) ) ;
#34265=CARTESIAN_POINT ( 'NONE',  ( 27.24356964374999635, 197.8718750006145513, -15.72908226750539029 ) ) ;
#34267=EDGE_CURVE ( 'NONE', #19072, #26373, #22965, .T. ) ;
#34275=CARTESIAN_POINT ( 'NONE',  ( 20.99999999999999289, 244.0374999999999943, -5.999999999999997335 ) ) ;
#34278=EDGE_CURVE ( 'NONE', #23622, #32985, #13725, .T. ) ;
#34279=AXIS2_PLACEMENT_3D ( 'NONE', #36228, #31115, #25420 ) ;
#34281=CARTESIAN_POINT ( 'NONE',  ( 21.00000000000000000, 248.7624999999999886, 5.999999999999998224 ) ) ;
#34286=CARTESIAN_POINT ( 'NONE',  ( 27.24356964375000345, 196.0343750006145456, -3.336375036156643733E-15 ) ) ;
#34291=CARTESIAN_POINT ( 'NONE',  ( 15.24356964374999990, 241.7218750006145171, -3.323476615752268604 ) ) ;
#34292=CARTESIAN_POINT ( 'NONE',  ( 13.62178482187501416, 198.6031250006145399, 23.59362340125806767 ) ) ;
#34297=CARTESIAN_POINT ( 'NONE',  ( 26.75643035624999655, 241.4218750006145058, -7.049594010296217766E-16 ) ) ;
#34306=CARTESIAN_POINT ( 'NONE',  ( 20.99999999999999645, 244.9093750006145171, 6.646953231504538984 ) ) ;
#34312=CARTESIAN_POINT ( 'NONE',  ( 0.000000000000000000, 210.0000000000000284, 0.000000000000000000 ) ) ;
#34326=CARTESIAN_POINT ( 'NONE',  ( 13.62178482187499640, 196.5593750006145513, -23.59362340125807123 ) ) ;
#34333=CARTESIAN_POINT ( 'NONE',  ( 21.00000000000000000, 240.0437500012290570, -6.928203230275506996 ) ) ;
#34352=ORIENTED_EDGE ( 'NONE', *, *, #7286, .T. ) ;
#34361=CARTESIAN_POINT ( 'NONE',  ( -26.99999999999999645, 196.1000000012290627, 15.58845726811991561 ) ) ;
#34367=EDGE_CURVE ( 'NONE', #2166, #36568, #27727, .T. ) ;
#34368=CARTESIAN_POINT ( 'NONE',  ( 26.99999999999999645, 246.2312500012290570, -7.347880794884117764E-16 ) ) ;
#34369=CARTESIAN_POINT ( 'NONE',  ( 26.75643035624999655, 244.2343750006145342, -7.049594010296217766E-16 ) ) ;
#34371=CARTESIAN_POINT ( 'NONE',  ( 18.12178482187499640, 242.5843750006145285, -4.985214923628404904 ) ) ;
#34376=CARTESIAN_POINT ( 'NONE',  ( 23.99999999999999645, 247.6562500012290400, -5.196152422706631135 ) ) ;
#34383=EDGE_LOOP ( 'NONE', ( #9215, #23594, #29139, #4319 ) ) ;
#34384=ORIENTED_EDGE ( 'NONE', *, *, #13611, .T. ) ;
#34389=CARTESIAN_POINT ( 'NONE',  ( 26.75643035624999655, 248.1718750006145342, -7.049594010296217766E-16 ) ) ;
#34393=CARTESIAN_POINT ( 'NONE',  ( 15.53186252112518417, 224.5816999436668482, 2.477503916096319703 ) ) ;
#34395=AXIS2_PLACEMENT_3D ( 'NONE', #28997, #6064, #31664 ) ;
#34408=CARTESIAN_POINT ( 'NONE',  ( 26.99999999999999645, 242.1437500012289945, 3.464101615137751278 ) ) ;
#34411=CARTESIAN_POINT ( 'NONE',  ( 18.00000000000000355, 243.3250000000000171, 5.196152422706632912 ) ) ;
#34420=CARTESIAN_POINT ( 'NONE',  ( 5.727106289114498080E-15, 196.9625000000000057, 31.17691453623979214 ) ) ;
#34421=AXIS2_PLACEMENT_3D ( 'NONE', #22166, #16476, #13632 ) ;
#34424=CARTESIAN_POINT ( 'NONE',  ( 26.75643035624999655, 248.2843750006145456, -7.049594010296217766E-16 ) ) ;
#34431=CARTESIAN_POINT ( 'NONE',  ( 26.99999999999999645, 242.6125000000000114, -3.464101615137755275 ) ) ;
#34436=CARTESIAN_POINT ( 'NONE',  ( -1.909035429704832693E-15, 196.4000000012290457, -31.17691453623979214 ) ) ;
#34440=CARTESIAN_POINT ( 'NONE',  ( 26.75643035624999655, 243.7843750006145456, -7.049594010296217766E-16 ) ) ;
#34442=CARTESIAN_POINT ( 'NONE',  ( 15.00000000000000000, 242.8562500012290286, 0.000000000000000000 ) ) ;
#34448=CARTESIAN_POINT ( 'NONE',  ( 24.32002691557804397, 195.0000000000000284, -11.86068704861160938 ) ) ;
#34449=CARTESIAN_POINT ( 'NONE',  ( -13.62178482187498396, 195.8843750006145399, 23.59362340125808188 ) ) ;
#34453=CARTESIAN_POINT ( 'NONE',  ( 18.00000000000000355, 240.6250000000000000, 5.196152422706632912 ) ) ;
#34454=DIRECTION ( 'NONE',  ( -0.000000000000000000, 1.000000000000000000, -0.000000000000000000 ) ) ;
#34468=CARTESIAN_POINT ( 'NONE',  ( 27.24356964375000700, 196.4468750006145399, 15.72908226750537075 ) ) ;
#34471=CYLINDRICAL_SURFACE ( 'NONE', #406, 5.999999999999999112 ) ;
#34472=CARTESIAN_POINT ( 'NONE',  ( 26.75643035624999655, 241.5343750006145456, -7.049594010296217766E-16 ) ) ;
#34473=CARTESIAN_POINT ( 'NONE',  ( -13.62178482187498396, 198.5281250006145228, 23.59362340125808188 ) ) ;
#34478=CARTESIAN_POINT ( 'NONE',  ( -13.62178482187498396, 197.6281250006145171, 23.59362340125808188 ) ) ;
#34479=CARTESIAN_POINT ( 'NONE',  ( 15.24356964375000167, 241.2343750006145058, 3.323476615752272600 ) ) ;
#34481=EDGE_CURVE ( 'NONE', #22146, #2118, #35630, .T. ) ;
#34490=CARTESIAN_POINT ( 'NONE',  ( 26.75643035624999655, 245.4718750006145171, -7.049594010296217766E-16 ) ) ;
#34491=CARTESIAN_POINT ( 'NONE',  ( 21.00000000000000000, 240.2125000000000057, 5.999999999999998224 ) ) ;
#34495=DIRECTION ( 'NONE',  ( -0.000000000000000000, -1.000000000000000000, -0.000000000000000000 ) ) ;
#34496=CARTESIAN_POINT ( 'NONE',  ( 20.99999999999999645, 249.2687500012290513, 5.999999999999998224 ) ) ;
#34500=( BOUNDED_CURVE ( )  B_SPLINE_CURVE ( 2, ( #234, #12171, #34730, #29033, #32074, #9341, #6103, #17686, #26573 ),
 .UNSPECIFIED., .F., .F. ) 
 B_SPLINE_CURVE_WITH_KNOTS ( ( 3, 2, 2, 2, 3 ),
 ( 0.7282608695652174058, 0.7318840579710145233, 0.7391304347826086474, 0.7463768115942028825, 0.7500000000000000000 ),
 .UNSPECIFIED. ) 
 CURVE ( )  GEOMETRIC_REPRESENTATION_ITEM ( )  RATIONAL_B_SPLINE_CURVE ( ( 0.9330127018922194093, 0.9330127018922194093, 1.000000000000000000, 0.8660254037844387076, 1.000000000000000000, 0.8660254037844387076, 1.000000000000000000, 0.9330127018922194093, 0.9330127018922194093 ) ) 
 REPRESENTATION_ITEM ( '' )  );
#34503=CARTESIAN_POINT ( 'NONE',  ( 24.00000000000000000, 245.7062500012290513, 5.196152422706629359 ) ) ;
#34511=CARTESIAN_POINT ( 'NONE',  ( -13.62178482187498396, 194.9843750006145626, 23.59362340125808188 ) ) ;
#34512=DIRECTION ( 'NONE',  ( 0.000000000000000000, 1.000000000000000000, 0.000000000000000000 ) ) ;
#34518=CARTESIAN_POINT ( 'NONE',  ( 23.87821517812499650, 248.6968750006145115, -4.985214923628404904 ) ) ;
#34527=CARTESIAN_POINT ( 'NONE',  ( 18.00000000000000000, 245.9312500012290457, -5.196152422706630247 ) ) ;
#34532=CARTESIAN_POINT ( 'NONE',  ( -26.99693289488239500, 195.0000000000001137, 2.389390116437581479 ) ) ;
#34551=CARTESIAN_POINT ( 'NONE',  ( 21.00000000000000000, 245.4718750006145456, 6.646953231504538984 ) ) ;
#34553=CARTESIAN_POINT ( 'NONE',  ( 23.87821517812500005, 242.8093750006145228, 4.985214923628404016 ) ) ;
#34558=CARTESIAN_POINT ( 'NONE',  ( 15.00000000000000000, 246.4187500012290286, -3.464101615137752166 ) ) ;
#34572=CARTESIAN_POINT ( 'NONE',  ( 21.00000000000000000, 247.3843750006145399, -6.646953231504538984 ) ) ;
#34587=CARTESIAN_POINT ( 'NONE',  ( 20.99999999999999289, 242.2937500012290570, -5.999999999999997335 ) ) ;
#34599=CARTESIAN_POINT ( 'NONE',  ( 13.49999999999999645, 196.2500000000000000, -23.38268590217984766 ) ) ;
#34602=CARTESIAN_POINT ( 'NONE',  ( 18.12178482187500350, 248.1343750006145399, 4.985214923628407568 ) ) ;
#34609=CARTESIAN_POINT ( 'NONE',  ( 21.00000000000000000, 240.6625000000000227, 6.928203230275506996 ) ) ;
#34611=EDGE_CURVE ( 'NONE', #483, #7130, #30210, .T. ) ;
#34615=CARTESIAN_POINT ( 'NONE',  ( -1.909035429704832693E-15, 195.5000000012290400, -31.17691453623979214 ) ) ;
#34619=CARTESIAN_POINT ( 'NONE',  ( 15.24356964375000167, 240.8968750006145001, 3.323476615752272600 ) ) ;
#34622=CARTESIAN_POINT ( 'NONE',  ( 19.39230484541323918, 242.7638461906614396, -5.999999999999987566 ) ) ;
#34627=CARTESIAN_POINT ( 'NONE',  ( 17.12995869703641816, 195.0000000000000284, 21.16104912388787795 ) ) ;
#34628=CARTESIAN_POINT ( 'NONE',  ( 27.24356964375000700, 196.4468750006145115, 15.72908226750537075 ) ) ;
#34630=EDGE_LOOP ( 'NONE', ( #3840, #25234, #20247, #7778 ) ) ;
#34633=CARTESIAN_POINT ( 'NONE',  ( 10.49999999999999645, 244.5000000000000000, 2.500000000000000000 ) ) ;
#34637=LINE ( 'NONE', #37293, #25805 ) ;
#34639=FACE_OUTER_BOUND ( 'NONE', #6791, .T. ) ;
#34643=CARTESIAN_POINT ( 'NONE',  ( -1.045839947578415010E-13, 195.1625000000000512, 27.00000000000000355 ) ) ;
#34644=ORIENTED_EDGE ( 'NONE', *, *, #30417, .F. ) ;
#34647=CARTESIAN_POINT ( 'NONE',  ( 27.24356964374999279, 196.5218750006145569, -15.72908226750539207 ) ) ;
#34651=CARTESIAN_POINT ( 'NONE',  ( 20.99999999999999645, 185.0294372515228645, -5.999999999999999112 ) ) ;
#34652=CARTESIAN_POINT ( 'NONE',  ( 18.00000000000000355, 249.1750000000000114, 5.196152422706632912 ) ) ;
#34653=CARTESIAN_POINT ( 'NONE',  ( -13.62178482187500528, 197.9281250006145569, -23.59362340125807123 ) ) ;
#34658=CARTESIAN_POINT ( 'NONE',  ( 5.778771075727756162E-15, 199.0156250006145342, 31.45816453501075927 ) ) ;
#34659=CARTESIAN_POINT ( 'NONE',  ( 15.24356964374999990, 242.9593750006145001, -3.323476615752268604 ) ) ;
#34660=CARTESIAN_POINT ( 'NONE',  ( 19.39230484541326049, 243.6075961894323143, -5.999999999999997335 ) ) ;
#34661=EDGE_CURVE ( 'NONE', #35593, #24310, #29759, .T. ) ;
#34669=CARTESIAN_POINT ( 'NONE',  ( 20.99999999999999645, 241.9843750006145058, -6.646953231504538984 ) ) ;
#34672=CARTESIAN_POINT ( 'NONE',  ( 20.99999999999997513, 246.7937500012290286, -5.999999999999999112 ) ) ;
#34677=DIRECTION ( 'NONE',  ( -0.000000000000000000, -1.000000000000000000, -0.000000000000000000 ) ) ;
#34684=CARTESIAN_POINT ( 'NONE',  ( 18.12178482187499640, 243.3718750006145228, -4.985214923628404904 ) ) ;
#34688=CARTESIAN_POINT ( 'NONE',  ( 26.99999999999999645, 243.9812500012290570, -7.347880794884117764E-16 ) ) ;
#34689=ADVANCED_FACE ( 'NONE', ( #24085 ), #18404, .F. ) ;
#34692=CARTESIAN_POINT ( 'NONE',  ( 27.24356964375000345, 196.4843750006145626, -3.336375036156643733E-15 ) ) ;
#34693=CARTESIAN_POINT ( 'NONE',  ( 26.99999999999999645, 246.1375000000000171, 3.464101615137751278 ) ) ;
#34699=CARTESIAN_POINT ( 'NONE',  ( 15.24356964375000167, 249.3343750006145001, 3.323476615752272600 ) ) ;
#34710=CARTESIAN_POINT ( 'NONE',  ( 23.87821517812500005, 248.0968750006144887, 4.985214923628404016 ) ) ;
#34712=CARTESIAN_POINT ( 'NONE',  ( -26.89802933101758242, 194.9999999999999432, -3.124506137021467289 ) ) ;
#34714=( BOUNDED_CURVE ( )  B_SPLINE_CURVE ( 2, ( #11010, #10635, #21840, #22397, #33765, #16522, #4578, #36406, #33946 ),
 .UNSPECIFIED., .F., .F. ) 
 B_SPLINE_CURVE_WITH_KNOTS ( ( 3, 2, 2, 2, 3 ),
 ( 0.6630434782608695121, 0.6666666666666666297, 0.6739130434782608647, 0.6811594202898550998, 0.6847826086956522174 ),
 .UNSPECIFIED. ) 
 CURVE ( )  GEOMETRIC_REPRESENTATION_ITEM ( )  RATIONAL_B_SPLINE_CURVE ( ( 0.9330127018922192983, 0.9330127018922182991, 1.000000000000000000, 0.8660254037844387076, 1.000000000000000000, 0.8660254037844387076, 1.000000000000000000, 0.9330127018922182991, 0.9330127018922192983 ) ) 
 REPRESENTATION_ITEM ( '' )  );
#34730=CARTESIAN_POINT ( 'NONE',  ( 18.00000000000000355, 242.4250000000000114, 5.196152422706632912 ) ) ;
#34733=LINE ( 'NONE', #29229, #32563 ) ;
#34734=ADVANCED_FACE ( 'NONE', ( #7772 ), #28228, .T. ) ;
#34738=CARTESIAN_POINT ( 'NONE',  ( 21.00000000000000000, 245.0218750006145285, 6.646953231504538984 ) ) ;
#34741=ORIENTED_EDGE ( 'NONE', *, *, #14005, .F. ) ;
#34744=CARTESIAN_POINT ( 'NONE',  ( 26.99999999999999645, 247.1687500012290570, -3.464101615137755275 ) ) ;
#34753=ORIENTED_EDGE ( 'NONE', *, *, #5250, .T. ) ;
#34758=CARTESIAN_POINT ( 'NONE',  ( 23.87821517812500005, 246.2968750006145058, 4.985214923628404016 ) ) ;
#34762=CARTESIAN_POINT ( 'NONE',  ( 19.55576478543629193, 211.4442352145561586, -5.894939585092063616 ) ) ;
#34774=CARTESIAN_POINT ( 'NONE',  ( 23.99999999999999645, 240.8500000000000227, -5.196152422706631135 ) ) ;
#34785=CARTESIAN_POINT ( 'NONE',  ( 5.727106289114498080E-15, 195.1625000000000227, 31.17691453623979214 ) ) ;
#34788=CARTESIAN_POINT ( 'NONE',  ( 26.75643035624999655, 247.8343750006145285, -7.049594010296217766E-16 ) ) ;
#34792=DIRECTION ( 'NONE',  ( 1.000000000000000000, 0.000000000000000000, 0.000000000000000000 ) ) ;
#34795=CARTESIAN_POINT ( 'NONE',  ( 24.00000000000000000, 242.0499999999999829, 5.196152422706629359 ) ) ;
#34801=CARTESIAN_POINT ( 'NONE',  ( 27.00000000000001066, 194.9000000012290457, 15.58845726811988897 ) ) ;
#34805=CARTESIAN_POINT ( 'NONE',  ( 23.87821517812500005, 240.1093750006145342, 4.985214923628404016 ) ) ;
#34814=FACE_OUTER_BOUND ( 'NONE', #7870, .T. ) ;
#34815=CARTESIAN_POINT ( 'NONE',  ( -27.24356964375001056, 194.8857344423495874, -9.915847621322177119 ) ) ;
#34817=ORIENTED_EDGE ( 'NONE', *, *, #1028, .T. ) ;
#34820=CARTESIAN_POINT ( 'NONE',  ( 7.234628195640309123, 198.9674038105676743, -27.00000000000000711 ) ) ;
#34826=CYLINDRICAL_SURFACE ( 'NONE', #15268, 5.999999999999999112 ) ;
#34834=CIRCLE ( 'NONE', #4485, 8.000000000000007105 ) ;
#34836=CARTESIAN_POINT ( 'NONE',  ( -27.24356964374999279, 195.3968750006145285, 15.72908226750539384 ) ) ;
#34839=CARTESIAN_POINT ( 'NONE',  ( 5.438367727407757144E-14, 198.0875000000000057, -27.00000000000000000 ) ) ;
#34840=CARTESIAN_POINT ( 'NONE',  ( 26.99999999999999645, 248.4250000000000114, -7.347880794884117764E-16 ) ) ;
#34841=CARTESIAN_POINT ( 'NONE',  ( 13.62178482187501416, 197.7031250006145342, 23.59362340125806767 ) ) ;
#34848=CARTESIAN_POINT ( 'NONE',  ( 13.62178482187501416, 198.1531250006145228, 23.59362340125806767 ) ) ;
#34849=CARTESIAN_POINT ( 'NONE',  ( 15.24356964375000167, 243.0343750006144887, 3.323476615752272600 ) ) ;
#34852=CARTESIAN_POINT ( 'NONE',  ( 26.75643035624999655, 246.5218750006145285, -3.323476615752271712 ) ) ;
#34856=CARTESIAN_POINT ( 'NONE',  ( 15.24356964374999990, 241.1968750006145115, 0.000000000000000000 ) ) ;
#34868=CARTESIAN_POINT ( 'NONE',  ( -20.68320042480035426, 195.0000000000000000, -17.35526491262920956 ) ) ;
#34872=CARTESIAN_POINT ( 'NONE',  ( 20.99999999999998579, 247.6937500012290059, -5.999999999999997335 ) ) ;
#34874=CARTESIAN_POINT ( 'NONE',  ( 23.87821517812500005, 243.1468750006145285, 4.985214923628404016 ) ) ;
#34881=CARTESIAN_POINT ( 'NONE',  ( 21.00000000000000000, 241.1125000000000114, 5.999999999999998224 ) ) ;
#34882=DIRECTION ( 'NONE',  ( 0.000000000000000000, 0.000000000000000000, -1.000000000000000000 ) ) ;
#34883=CARTESIAN_POINT ( 'NONE',  ( -27.24356964374999990, 196.6718750006145342, -15.72908226750537786 ) ) ;
#34884=CARTESIAN_POINT ( 'NONE',  ( 20.99999999999999645, 185.0294372515228645, 0.000000000000000000 ) ) ;
#34889=CARTESIAN_POINT ( 'NONE',  ( 15.24356964374999990, 249.7093750006145285, -3.323476615752268604 ) ) ;
#34894=EDGE_CURVE ( 'NONE', #27300, #9547, #18658, .T. ) ;
#34895=VERTEX_POINT ( 'NONE', #30710 ) ;
#34900=CARTESIAN_POINT ( 'NONE',  ( 26.75643035624999655, 249.5218750006145001, -7.049594010296217766E-16 ) ) ;
#34901=AXIS2_PLACEMENT_3D ( 'NONE', #3582, #9459, #3763 ) ;
#34902=CARTESIAN_POINT ( 'NONE',  ( -25.24001216047315310, 194.9999999999999716, 9.971080493324555150 ) ) ;
#34903=EDGE_CURVE ( 'NONE', #20369, #18467, #34080, .T. ) ;
#34908=DIRECTION ( 'NONE',  ( -0.000000000000000000, 1.000000000000000000, -0.000000000000000000 ) ) ;
#34914=ORIENTED_EDGE ( 'NONE', *, *, #34206, .F. ) ;
#34920=CARTESIAN_POINT ( 'NONE',  ( 7.234628195640269155, 196.1950961906613600, 27.00000000000003197 ) ) ;
#34923=CARTESIAN_POINT ( 'NONE',  ( 15.24356964374999990, 244.4218750006145058, -3.323476615752268604 ) ) ;
#34928=CARTESIAN_POINT ( 'NONE',  ( 18.00000000000000355, 246.0812500012290513, 5.196152422706632912 ) ) ;
#34931=CARTESIAN_POINT ( 'NONE',  ( 13.49999999999999645, 198.1625000012290343, -23.38268590217984766 ) ) ;
#34935=ORIENTED_EDGE ( 'NONE', *, *, #1776, .T. ) ;
#34939=CARTESIAN_POINT ( 'NONE',  ( 18.12178482187499640, 246.9718750006145171, -4.985214923628404904 ) ) ;
#34944=CARTESIAN_POINT ( 'NONE',  ( 20.60729646369627943, 211.0472094301501045, -5.999999999999998224 ) ) ;
#34952=CARTESIAN_POINT ( 'NONE',  ( 13.62178482187501416, 195.0031250006145456, 23.59362340125806767 ) ) ;
#34968=DIRECTION ( 'NONE',  ( -0.000000000000000000, 1.000000000000000000, -0.000000000000000000 ) ) ;
#34970=CARTESIAN_POINT ( 'NONE',  ( -27.00000000000000355, 195.9500000000000171, 0.000000000000000000 ) ) ;
#34971=CARTESIAN_POINT ( 'NONE',  ( 15.00000000000000000, 240.0625000000000000, -3.464101615137752610 ) ) ;
#34973=CARTESIAN_POINT ( 'NONE',  ( 15.24356964374999990, 246.7093750006145569, 0.000000000000000000 ) ) ;
#34978=CARTESIAN_POINT ( 'NONE',  ( 20.99999999999999645, 185.0294372515228645, 0.000000000000000000 ) ) ;
#34981=CARTESIAN_POINT ( 'NONE',  ( 15.00000000000000178, 240.1374999999999886, 3.464101615137757051 ) ) ;
#34993=CARTESIAN_POINT ( 'NONE',  ( 26.75643035624999655, 240.6718750006145910, -3.323476615752271712 ) ) ;
#35002=CARTESIAN_POINT ( 'NONE',  ( 24.79149224591586886, 195.0000000000000284, -10.85399214561028280 ) ) ;
#35003=CARTESIAN_POINT ( 'NONE',  ( -1.926257025242585782E-15, 196.1468750006145285, -31.45816453501075927 ) ) ;
#35024=CARTESIAN_POINT ( 'NONE',  ( 5.778771075727756162E-15, 195.4718750006145171, 31.45816453501076637 ) ) ;
#35028=CARTESIAN_POINT ( 'NONE',  ( 26.99999999999999645, 248.0125000000000171, -3.464101615137755275 ) ) ;
#35029=CARTESIAN_POINT ( 'NONE',  ( -27.24356964374999279, 197.5906250006144944, 15.72908226750539384 ) ) ;
#35033=ORIENTED_EDGE ( 'NONE', *, *, #16847, .F. ) ;
#35034=CARTESIAN_POINT ( 'NONE',  ( -27.24356964374999990, 196.6156250006145285, -15.72908226750537786 ) ) ;
#35035=CARTESIAN_POINT ( 'NONE',  ( 26.75643035624999655, 242.7718750006145001, -7.049594010296217766E-16 ) ) ;
#35038=CARTESIAN_POINT ( 'NONE',  ( 23.87821517812500005, 247.7593750006145399, 4.985214923628404016 ) ) ;
#35042=CARTESIAN_POINT ( 'NONE',  ( 15.24356964374999990, 241.6093750006145342, -3.323476615752268604 ) ) ;
#35051=CARTESIAN_POINT ( 'NONE',  ( 26.99999999999999645, 248.3875000000000171, 3.464101615137751278 ) ) ;
#35058=CARTESIAN_POINT ( 'NONE',  ( 21.00000000000000000, 242.2093750006145285, 6.646953231504538984 ) ) ;
#35059=ORIENTED_EDGE ( 'NONE', *, *, #4506, .T. ) ;
#35063=CARTESIAN_POINT ( 'NONE',  ( 22.60769515458671108, 241.5825961894323086, 6.000000000000010658 ) ) ;
#35066=CARTESIAN_POINT ( 'NONE',  ( -7.946041369334237991, 195.0000000000000000, 26.05901981062767092 ) ) ;
#35071=EDGE_LOOP ( 'NONE', ( #20368, #16570, #1748, #36796 ) ) ;
#35072=CARTESIAN_POINT ( 'NONE',  ( 19.95811728174978228, 239.6067735352071679, -5.908847637349563087 ) ) ;
#35083=CARTESIAN_POINT ( 'NONE',  ( 15.00000000000000000, 245.5562500012290457, 0.000000000000000000 ) ) ;
#35085=ADVANCED_FACE ( 'NONE', ( #22550 ), #34471, .F. ) ;
#35086=CARTESIAN_POINT ( 'NONE',  ( -25.03348993865347438, 194.9999999999999432, 10.48541407139706649 ) ) ;
#35102=AXIS2_PLACEMENT_3D ( 'NONE', #34884, #17277, #8924 ) ;
#35105=CARTESIAN_POINT ( 'NONE',  ( 20.99999999999999289, 244.4874999999999829, -5.999999999999997335 ) ) ;
#35108=CARTESIAN_POINT ( 'NONE',  ( 18.12178482187499640, 244.8343750006145285, -4.985214923628404904 ) ) ;
#35113=CARTESIAN_POINT ( 'NONE',  ( 18.00000000000000000, 247.2812500012290400, -5.196152422706630247 ) ) ;
#35124=CARTESIAN_POINT ( 'NONE',  ( 15.24356964374999990, 247.0093750006145115, -3.323476615752268604 ) ) ;
#35133=CARTESIAN_POINT ( 'NONE',  ( 2.999999999999997335, 244.5000000000000000, 2.500000000000000000 ) ) ;
#35140=CARTESIAN_POINT ( 'NONE',  ( 21.00000000000000000, 243.3624999999999829, 5.999999999999998224 ) ) ;
#35151=CARTESIAN_POINT ( 'NONE',  ( 19.39230484541326760, 240.1924038105676686, 5.999999999999999112 ) ) ;
#35153=CARTESIAN_POINT ( 'NONE',  ( 23.87821517812500005, 246.8593750006145342, 4.985214923628404016 ) ) ;
#35156=CARTESIAN_POINT ( 'NONE',  ( -29.00000000000002487, 210.0000000000000000, 8.000000000000000000 ) ) ;
#35161=( BOUNDED_CURVE ( )  B_SPLINE_CURVE ( 2, ( #37332, #23320, #37153, #25969, #8726, #2842, #20108, #11194, #11382 ),
 .UNSPECIFIED., .F., .F. ) 
 B_SPLINE_CURVE_WITH_KNOTS ( ( 3, 2, 2, 2, 3 ),
 ( 0.7717391304347825942, 0.7753623188405797118, 0.7826086956521739468, 0.7898550724637680709, 0.7934782608695651884 ),
 .UNSPECIFIED. ) 
 CURVE ( )  GEOMETRIC_REPRESENTATION_ITEM ( )  RATIONAL_B_SPLINE_CURVE ( ( 0.9330127018922194093, 0.9330127018922194093, 1.000000000000000000, 0.8660254037844387076, 1.000000000000000000, 0.8660254037844387076, 1.000000000000000000, 0.9330127018922194093, 0.9330127018922194093 ) ) 
 REPRESENTATION_ITEM ( '' )  );
#35162=CARTESIAN_POINT ( 'NONE',  ( 18.00000000000000000, 241.3750000000000000, -5.196152422706630247 ) ) ;
#35163=CARTESIAN_POINT ( 'NONE',  ( -6.797719915734056428, 221.2600545691329330, 2.615526397346993992 ) ) ;
#35164=EDGE_CURVE ( 'NONE', #7787, #12569, #24132, .T. ) ;
#35175=CARTESIAN_POINT ( 'NONE',  ( 21.00000000000000000, 241.4218750006145626, 6.646953231504538984 ) ) ;
#35178=CARTESIAN_POINT ( 'NONE',  ( -4.914563035147740067, 224.9123314610253317, 2.500000000000000000 ) ) ;
#35183=( BOUNDED_CURVE ( )  B_SPLINE_CURVE ( 2, ( #11013, #7990, #14235, #16714, #28807, #22957, #34503, #28261, #28621 ),
 .UNSPECIFIED., .F., .F. ) 
 B_SPLINE_CURVE_WITH_KNOTS ( ( 3, 2, 2, 2, 3 ),
 ( 0.3586956521739130266, 0.3623188405797101441, 0.3695652173913043237, 0.3768115942028985588, 0.3804347826086956763 ),
 .UNSPECIFIED. ) 
 CURVE ( )  GEOMETRIC_REPRESENTATION_ITEM ( )  RATIONAL_B_SPLINE_CURVE ( ( 0.9330127018922191873, 0.9330127018922187432, 1.000000000000000000, 0.8660254037844387076, 1.000000000000000000, 0.8660254037844387076, 1.000000000000000000, 0.9330127018922188542, 0.9330127018922194093 ) ) 
 REPRESENTATION_ITEM ( '' )  );
#35185=CARTESIAN_POINT ( 'NONE',  ( 19.20301275210649905, 194.9999999999999147, -19.02731729069157396 ) ) ;
#35186=CARTESIAN_POINT ( 'NONE',  ( 5.778771075727756162E-15, 195.0218750006145569, 31.45816453501075927 ) ) ;
#35191=CARTESIAN_POINT ( 'NONE',  ( 22.60769515458672885, 245.4236538117966973, -5.999999999999998224 ) ) ;
#35197=CARTESIAN_POINT ( 'NONE',  ( 18.00000000000000355, 240.6812500012290457, 5.196152422706632912 ) ) ;
#35198=CARTESIAN_POINT ( 'NONE',  ( 20.99999999999999289, 244.9374999999999716, -5.999999999999997335 ) ) ;
#35200=CARTESIAN_POINT ( 'NONE',  ( 13.50000000000001421, 199.3625000012290513, 23.38268590217984055 ) ) ;
#35202=VERTEX_POINT ( 'NONE', #8333 ) ;
#35210=CARTESIAN_POINT ( 'NONE',  ( 23.99999999999999645, 249.4000000000000057, -5.196152422706631135 ) ) ;
#35211=CARTESIAN_POINT ( 'NONE',  ( -27.24356964375000345, 196.6156250006145285, -15.72908226750537786 ) ) ;
#35217=CARTESIAN_POINT ( 'NONE',  ( 13.62178482187499640, 196.0531250006145285, -23.59362340125807123 ) ) ;
#35221=CARTESIAN_POINT ( 'NONE',  ( 26.75643035624999655, 246.9718750006145740, -3.323476615752271712 ) ) ;
#35228=CARTESIAN_POINT ( 'NONE',  ( 26.75643035624999655, 240.9343750006145228, 3.323476615752267271 ) ) ;
#35239=CARTESIAN_POINT ( 'NONE',  ( 3.551475717527324030E-15, 195.0000000000000000, 28.99999999999999645 ) ) ;
#35244=CARTESIAN_POINT ( 'NONE',  ( 15.24356964375000167, 242.5843750006145285, 3.323476615752272600 ) ) ;
#35248=CARTESIAN_POINT ( 'NONE',  ( 27.24356964375000345, 199.1843750006145228, -3.336375036156643733E-15 ) ) ;
#35254=ORIENTED_EDGE ( 'NONE', *, *, #15502, .T. ) ;
#35255=CARTESIAN_POINT ( 'NONE',  ( 18.12178482187499640, 247.4218750006145342, -4.985214923628404904 ) ) ;
#35266=LINE ( 'NONE', #12345, #9512 ) ;
#35267=CARTESIAN_POINT ( 'NONE',  ( -25.48128045151071319, 194.9999999999999432, -9.080314936885052646 ) ) ;
#35270=EDGE_CURVE ( 'NONE', #9065, #5908, #5653, .T. ) ;
#35273=CARTESIAN_POINT ( 'NONE',  ( 21.00000000000000000, 248.7624999999999886, 5.999999999999998224 ) ) ;
#35277=CARTESIAN_POINT ( 'NONE',  ( 15.00000000000000000, 246.4562500012290513, 0.000000000000000000 ) ) ;
#35288=CARTESIAN_POINT ( 'NONE',  ( 27.00000000000000355, 197.5250000000000057, -3.306546357697854128E-15 ) ) ;
#35291=CARTESIAN_POINT ( 'NONE',  ( 26.75643035624999655, 242.8468750006145456, 3.323476615752267715 ) ) ;
#35294=ORIENTED_EDGE ( 'NONE', *, *, #24986, .F. ) ;
#35295=CARTESIAN_POINT ( 'NONE',  ( 21.00000000000000000, 245.4437500012290059, -6.928203230275506996 ) ) ;
#35302=ADVANCED_FACE ( 'NONE', ( #28587 ), #19903, .T. ) ;
#35304=CIRCLE ( 'NONE', #30495, 8.000000000000000000 ) ;
#35305=ORIENTED_EDGE ( 'NONE', *, *, #2652, .F. ) ;
#35308=CARTESIAN_POINT ( 'NONE',  ( 26.75643035624999655, 246.3343750006145285, 3.323476615752267715 ) ) ;
#35311=CARTESIAN_POINT ( 'NONE',  ( 18.34109276191939841, 217.0904193015636281, -5.392997762649389237 ) ) ;
#35336=CARTESIAN_POINT ( 'NONE',  ( 20.99999999999999645, 247.7218750006145456, 6.646953231504538984 ) ) ;
#35340=CARTESIAN_POINT ( 'NONE',  ( 15.24356964375000167, 242.5843750006145285, 3.323476615752272600 ) ) ;
#35341=CYLINDRICAL_SURFACE ( 'NONE', #12959, 8.000000000000000000 ) ;
#35347=CARTESIAN_POINT ( 'NONE',  ( 24.00000000000000000, 241.1500000000000057, 5.196152422706629359 ) ) ;
#35348=DIRECTION ( 'NONE',  ( -0.000000000000000000, 1.000000000000000000, -0.000000000000000000 ) ) ;
#35353=CARTESIAN_POINT ( 'NONE',  ( 26.99999999999999645, 196.7750000012290172, -15.58845726811990495 ) ) ;
#35355=CARTESIAN_POINT ( 'NONE',  ( -20.68320086892770604, 194.6619763917542514, -17.35526438333879540 ) ) ;
#35361=CARTESIAN_POINT ( 'NONE',  ( 21.00000000000000000, 240.5218750006145285, 6.646953231504538984 ) ) ;
#35369=CARTESIAN_POINT ( 'NONE',  ( 19.39230484541326760, 241.0924038105676743, 5.999999999999999112 ) ) ;
#35370=CARTESIAN_POINT ( 'NONE',  ( 27.24356964375000700, 198.1906250006145740, 15.72908226750537075 ) ) ;
#35376=CARTESIAN_POINT ( 'NONE',  ( 21.00000000000000000, 245.2187500012290116, 5.999999999999998224 ) ) ;
#35377=CARTESIAN_POINT ( 'NONE',  ( -3.253724281355068545E-15, 198.9874999999999829, -27.00000000000000000 ) ) ;
#35384=CARTESIAN_POINT ( 'NONE',  ( 20.99999999999995381, 241.5625000000000000, 5.999999999999998224 ) ) ;
#35397=CARTESIAN_POINT ( 'NONE',  ( 15.00000000000000000, 248.6125000000000114, -3.464101615137752166 ) ) ;
#35398=CARTESIAN_POINT ( 'NONE',  ( 27.24356964375000345, 196.4281250006145569, -3.336375036156643733E-15 ) ) ;
#35402=CARTESIAN_POINT ( 'NONE',  ( 27.24356964375000700, 196.8406250006145513, 15.72908226750537075 ) ) ;
#35403=CARTESIAN_POINT ( 'NONE',  ( 18.12178482187499640, 240.2218750006145171, -4.985214923628404904 ) ) ;
#35405=AXIS2_PLACEMENT_3D ( 'NONE', #31081, #16683, #25385 ) ;
#35407=CARTESIAN_POINT ( 'NONE',  ( 21.00000000000000000, 247.2718750006145569, 6.646953231504538984 ) ) ;
#35410=CARTESIAN_POINT ( 'NONE',  ( 26.99999999999999645, 243.0437500012290855, 3.464101615137751278 ) ) ;
#35428=CARTESIAN_POINT ( 'NONE',  ( 5.438367727407757775E-14, 198.2000000012290002, -27.00000000000000355 ) ) ;
#35434=CARTESIAN_POINT ( 'NONE',  ( 21.00000000000000000, 241.0843750006145285, -6.646953231504538984 ) ) ;
#35437=B_SPLINE_CURVE_WITH_KNOTS ( 'NONE', 3,
 ( #31933, #23228, #12029, #645 ),
 .UNSPECIFIED., .F., .F.,
 ( 4, 4 ),
 ( 0.000000000000000000, 1.000000000000000000 ),
 .UNSPECIFIED. ) ;
#35439=CARTESIAN_POINT ( 'NONE',  ( 20.99999999999999289, 242.6875000000000000, -5.999999999999997335 ) ) ;
#35441=FACE_OUTER_BOUND ( 'NONE', #17240, .T. ) ;
#35448=CARTESIAN_POINT ( 'NONE',  ( 18.12178482187500350, 246.2218750006145171, 4.985214923628407568 ) ) ;
#35459=AXIS2_PLACEMENT_3D ( 'NONE', #14746, #18159, #17970 ) ;
#35461=CARTESIAN_POINT ( 'NONE',  ( 20.99999999999997868, 245.6687500012291139, 5.999999999999999112 ) ) ;
#35467=DIRECTION ( 'NONE',  ( -0.000000000000000000, 1.000000000000000000, -0.000000000000000000 ) ) ;
#35482=LINE ( 'NONE', #605, #20201 ) ;
#35488=VERTEX_POINT ( 'NONE', #3569 ) ;
#35489=CARTESIAN_POINT ( 'NONE',  ( 26.99999999999999645, 244.8437500012290400, 3.464101615137751278 ) ) ;
#35498=ADVANCED_FACE ( 'NONE', ( #29715 ), #30616, .F. ) ;
#35501=CARTESIAN_POINT ( 'NONE',  ( 18.12178482187500350, 245.3218750006145115, 4.985214923628407568 ) ) ;
#35514=DIRECTION ( 'NONE',  ( -0.000000000000000000, 1.000000000000000000, -0.000000000000000000 ) ) ;
#35517=VECTOR ( 'NONE', #26997, 1000.000000000000000 ) ;
#35521=EDGE_CURVE ( 'NONE', #22884, #23722, #27575, .T. ) ;
#35530=CARTESIAN_POINT ( 'NONE',  ( -13.49999999999998401, 195.5749999999999886, 23.38268590217985476 ) ) ;
#35532=CARTESIAN_POINT ( 'NONE',  ( 15.00000000000000000, 247.3562500012290570, 0.000000000000000000 ) ) ;
#35534=CARTESIAN_POINT ( 'NONE',  ( 15.24356964374999990, 245.3593750006145342, 0.000000000000000000 ) ) ;
#35541=CARTESIAN_POINT ( 'NONE',  ( -29.00000000000002487, 204.0000000000000000, 0.000000000000000000 ) ) ;
#35547=FACE_BOUND ( 'NONE', #26103, .T. ) ;
#35550=CARTESIAN_POINT ( 'NONE',  ( 26.99999999999999645, 243.0625000000000284, -3.464101615137755275 ) ) ;
#35554=CARTESIAN_POINT ( 'NONE',  ( 23.99999999999999645, 243.6062500012290286, -5.196152422706631135 ) ) ;
#35564=CARTESIAN_POINT ( 'NONE',  ( -27.24356964375000345, 198.0031250006145456, 0.000000000000000000 ) ) ;
#35568=ORIENTED_EDGE ( 'NONE', *, *, #12401, .F. ) ;
#35570=CARTESIAN_POINT ( 'NONE',  ( 20.99999999999999645, 243.8687500012290172, 5.999999999999998224 ) ) ;
#35577=DIRECTION ( 'NONE',  ( -0.000000000000000000, 1.000000000000000000, -0.000000000000000000 ) ) ;
#35580=CARTESIAN_POINT ( 'NONE',  ( -5.732297079746171420, 222.9518338469886203, 2.500000000000000000 ) ) ;
#35586=DIRECTION ( 'NONE',  ( 0.000000000000000000, 0.000000000000000000, 1.000000000000000000 ) ) ;
#35589=CARTESIAN_POINT ( 'NONE',  ( 18.00000000000000000, 245.4250000000000114, -5.196152422706630247 ) ) ;
#35590=CARTESIAN_POINT ( 'NONE',  ( 13.62178482187501416, 195.9031250006145513, 23.59362340125806767 ) ) ;
#35593=VERTEX_POINT ( 'NONE', #16211 ) ;
#35594=AXIS2_PLACEMENT_3D ( 'NONE', #1926, #10834, #28269 ) ;
#35596=CARTESIAN_POINT ( 'NONE',  ( -27.24356964375000345, 194.8531250006145115, 0.000000000000000000 ) ) ;
#35597=CARTESIAN_POINT ( 'NONE',  ( 21.00000000000000000, 239.9593750006145001, 6.646953231504538984 ) ) ;
#35600=CARTESIAN_POINT ( 'NONE',  ( 26.75643035624999655, 247.8718750006145228, -3.323476615752271712 ) ) ;
#35602=CYLINDRICAL_SURFACE ( 'NONE', #34901, 27.00000000000000000 ) ;
#35608=CARTESIAN_POINT ( 'NONE',  ( 26.75643035624999655, 240.5593750006145228, -3.323476615752271268 ) ) ;
#35623=CARTESIAN_POINT ( 'NONE',  ( 23.87821517812500005, 240.8968750006145285, 4.985214923628404016 ) ) ;
#35627=CARTESIAN_POINT ( 'NONE',  ( -27.24356964375000345, 199.8218750006145399, -15.72908226750537786 ) ) ;
#35629=DIRECTION ( 'NONE',  ( -0.000000000000000000, -1.000000000000000000, -0.000000000000000000 ) ) ;
#35630=LINE ( 'NONE', #24275, #25910 ) ;
#35636=CARTESIAN_POINT ( 'NONE',  ( 23.87821517812500005, 246.7468750006145228, 4.985214923628404016 ) ) ;
#35638=EDGE_CURVE ( 'NONE', #9537, #21289, #25347, .T. ) ;
#35641=ADVANCED_FACE ( 'NONE', ( #36657 ), #28977, .F. ) ;
#35643=CARTESIAN_POINT ( 'NONE',  ( 20.99999999999999289, 244.0937500012290116, -5.999999999999997335 ) ) ;
#35646=ORIENTED_EDGE ( 'NONE', *, *, #24836, .F. ) ;
#35650=ADVANCED_FACE ( 'NONE', ( #9453 ), #32944, .F. ) ;
#35652=CARTESIAN_POINT ( 'NONE',  ( 20.99999999999999645, 247.3843750006145399, -6.646953231504538984 ) ) ;
#35653=DIRECTION ( 'NONE',  ( -0.000000000000000000, -1.000000000000000000, -0.000000000000000000 ) ) ;
#35657=ORIENTED_EDGE ( 'NONE', *, *, #12973, .F. ) ;
#35658=CARTESIAN_POINT ( 'NONE',  ( 23.99999999999999645, 248.1062500012290570, -5.196152422706631135 ) ) ;
#35672=CARTESIAN_POINT ( 'NONE',  ( 13.50000000000001421, 196.5500000000000114, 23.38268590217984055 ) ) ;
#35677=CARTESIAN_POINT ( 'NONE',  ( 20.99999999999997513, 246.3437500012290684, -5.999999999999999112 ) ) ;
#35679=CARTESIAN_POINT ( 'NONE',  ( 23.99999999999999645, 244.9562500012290513, -5.196152422706631135 ) ) ;
#35682=CARTESIAN_POINT ( 'NONE',  ( 19.39230484541326049, 242.7075961894323655, -5.999999999999997335 ) ) ;
#35687=CARTESIAN_POINT ( 'NONE',  ( 21.00000000000000000, 244.4593750006145001, 6.646953231504538984 ) ) ;
#35711=DIRECTION ( 'NONE',  ( 0.000000000000000000, 0.000000000000000000, 1.000000000000000000 ) ) ;
#35713=CYLINDRICAL_SURFACE ( 'NONE', #6841, 5.999999999999999112 ) ;
#35715=CARTESIAN_POINT ( 'NONE',  ( 19.39230484541326049, 247.2638461906613827, -5.999999999999994671 ) ) ;
#35717=CARTESIAN_POINT ( 'NONE',  ( 26.75643035624999655, 246.0343750006145456, -7.049594010296217766E-16 ) ) ;
#35735=AXIS2_PLACEMENT_3D ( 'NONE', #3904, #1241, #9784 ) ;
#35739=CARTESIAN_POINT ( 'NONE',  ( 17.34006124879866917, 219.7598366698699692, 4.770645753574776826 ) ) ;
#35748=CARTESIAN_POINT ( 'NONE',  ( 13.62178482187499640, 198.7531250006145456, -23.59362340125807123 ) ) ;
#35761=CARTESIAN_POINT ( 'NONE',  ( 3.306546357697853733E-15, 210.0000000000000284, 27.00000000000000000 ) ) ;
#35767=CARTESIAN_POINT ( 'NONE',  ( 7.234628195640318005, 199.4174038105677198, -26.99999999999999645 ) ) ;
#35769=EDGE_LOOP ( 'NONE', ( #7152, #36610, #23057, #22259 ) ) ;
#35775=CARTESIAN_POINT ( 'NONE',  ( 15.00000000000000000, 246.4000000000000057, 0.000000000000000000 ) ) ;
#35776=CARTESIAN_POINT ( 'NONE',  ( -27.24356964374999279, 195.3406250006145228, 15.72908226750539384 ) ) ;
#35782=ORIENTED_EDGE ( 'NONE', *, *, #7760, .T. ) ;
#35783=CARTESIAN_POINT ( 'NONE',  ( 27.24356964375000700, 196.3906250006145058, 15.72908226750537075 ) ) ;
#35788=CARTESIAN_POINT ( 'NONE',  ( 15.24356964375000167, 244.9468750006145399, 3.323476615752272600 ) ) ;
#35794=CARTESIAN_POINT ( 'NONE',  ( 23.87821517812500005, 240.4468750006145115, 4.985214923628404016 ) ) ;
#35800=CARTESIAN_POINT ( 'NONE',  ( 20.99999999999999645, 185.0294372515228645, 0.000000000000000000 ) ) ;
#35803=CARTESIAN_POINT ( 'NONE',  ( 24.00000000000000000, 248.3499999999999943, 5.196152422706629359 ) ) ;
#35805=EDGE_CURVE ( 'NONE', #26422, #18816, #19050, .T. ) ;
#35807=CARTESIAN_POINT ( 'NONE',  ( 15.00000000000000000, 248.2562500012290627, 0.000000000000000000 ) ) ;
#35808=ADVANCED_FACE ( 'NONE', ( #13242 ), #33697, .F. ) ;
#35811=CARTESIAN_POINT ( 'NONE',  ( 15.24356964374999990, 248.9218750006145058, -3.323476615752268604 ) ) ;
#35815=CARTESIAN_POINT ( 'NONE',  ( -27.24356964375000345, 199.3718750006145513, -15.72908226750537786 ) ) ;
#35817=CARTESIAN_POINT ( 'NONE',  ( 19.98631459334238514, 239.9067735275330904, -5.748934852092073555 ) ) ;
#35818=CARTESIAN_POINT ( 'NONE',  ( 20.99999999999999645, 185.0294372515228645, 0.000000000000000000 ) ) ;
#35824=ORIENTED_EDGE ( 'NONE', *, *, #10189, .T. ) ;
#35825=CARTESIAN_POINT ( 'NONE',  ( 15.24356964375000167, 247.9843750006145058, 3.323476615752272600 ) ) ;
#35831=DIRECTION ( 'NONE',  ( 0.000000000000000000, -1.000000000000000000, 0.000000000000000000 ) ) ;
#35839=CARTESIAN_POINT ( 'NONE',  ( 26.75643035624999655, 245.8843750006145115, 3.323476615752267271 ) ) ;
#35845=CARTESIAN_POINT ( 'NONE',  ( 26.99999999999999645, 241.7687500012290513, -3.464101615137755275 ) ) ;
#35850=CARTESIAN_POINT ( 'NONE',  ( 19.39230484541324273, 241.5424038105676914, 5.999999999999987566 ) ) ;
#35859=CARTESIAN_POINT ( 'NONE',  ( 20.99999999999997868, 245.1625000000000227, 5.999999999999999112 ) ) ;
#35860=CARTESIAN_POINT ( 'NONE',  ( -1.909035429704832693E-15, 196.2875000000000227, -31.17691453623979214 ) ) ;
#35862=CARTESIAN_POINT ( 'NONE',  ( 10.49999999999999645, 244.5000000000000000, -2.500000000000000000 ) ) ;
#35866=CARTESIAN_POINT ( 'NONE',  ( 15.00000000000000000, 243.7187500012290684, -3.464101615137752166 ) ) ;
#35872=ORIENTED_EDGE ( 'NONE', *, *, #10512, .F. ) ;
#35873=FACE_OUTER_BOUND ( 'NONE', #27636, .T. ) ;
#35874=CARTESIAN_POINT ( 'NONE',  ( 26.75643035624999655, 244.5343750006144887, 3.323476615752267715 ) ) ;
#35876=VECTOR ( 'NONE', #32962, 1000.000000000000000 ) ;
#35888=CIRCLE ( 'NONE', #19582, 6.000000000000005329 ) ;
#35894=CARTESIAN_POINT ( 'NONE',  ( -28.29769750636678793, 205.1215485303246453, -6.345809158763446867 ) ) ;
#35895=EDGE_LOOP ( 'NONE', ( #30528, #5011, #1466, #9715 ) ) ;
#35899=DIRECTION ( 'NONE',  ( -0.000000000000000000, -1.000000000000000000, -0.000000000000000000 ) ) ;
#35901=DIRECTION ( 'NONE',  ( 0.000000000000000000, 0.000000000000000000, 1.000000000000000000 ) ) ;
#35903=CARTESIAN_POINT ( 'NONE',  ( 26.75643035624999655, 249.2218750006144887, -3.323476615752271712 ) ) ;
#35905=CARTESIAN_POINT ( 'NONE',  ( 20.99999999999999645, 244.3468750006145171, -6.646953231504538984 ) ) ;
#35914=ORIENTED_EDGE ( 'NONE', *, *, #27085, .T. ) ;
#35917=VERTEX_POINT ( 'NONE', #13617 ) ;
#35927=CARTESIAN_POINT ( 'NONE',  ( 16.85147890419444394, 211.5556954109258641, 5.808099892140972109 ) ) ;
#35937=CARTESIAN_POINT ( 'NONE',  ( -27.24356964374999990, 197.5156250006145626, -15.72908226750537786 ) ) ;
#35940=ORIENTED_EDGE ( 'NONE', *, *, #14499, .F. ) ;
#35953=AXIS2_PLACEMENT_3D ( 'NONE', #19801, #25465, #33437 ) ;
#35956=CARTESIAN_POINT ( 'NONE',  ( 13.50000000000001421, 199.7000000000000171, 23.38268590217984055 ) ) ;
#35957=DIRECTION ( 'NONE',  ( 0.000000000000000000, 0.000000000000000000, 1.000000000000000000 ) ) ;
#35960=DIRECTION ( 'NONE',  ( -0.000000000000000000, -0.000000000000000000, 1.000000000000000000 ) ) ;
#35966=CARTESIAN_POINT ( 'NONE',  ( 26.99999999999999645, 246.1375000000000171, 3.464101615137751278 ) ) ;
#35967=CARTESIAN_POINT ( 'NONE',  ( -27.24356964375000345, 196.6531250006145513, 0.000000000000000000 ) ) ;
#35971=ORIENTED_EDGE ( 'NONE', *, *, #25685, .F. ) ;
#35973=CARTESIAN_POINT ( 'NONE',  ( -1.909035429704832693E-15, 198.6500000012290457, -31.17691453623979214 ) ) ;
#35978=CARTESIAN_POINT ( 'NONE',  ( 26.75643035624999655, 246.0343750006145456, -7.049594010296217766E-16 ) ) ;
#35985=CARTESIAN_POINT ( 'NONE',  ( 20.99999999999999645, 240.6343750006145115, -6.646953231504538984 ) ) ;
#35989=EDGE_CURVE ( 'NONE', #10943, #37177, #16383, .T. ) ;
#35994=CARTESIAN_POINT ( 'NONE',  ( 19.39230484541326049, 244.0575961894323598, -5.999999999999997335 ) ) ;
#36000=CARTESIAN_POINT ( 'NONE',  ( 21.00000000000000000, 240.4093750006145171, 6.646953231504538984 ) ) ;
#36006=CYLINDRICAL_SURFACE ( 'NONE', #28778, 5.999999999999999112 ) ;
#36008=CARTESIAN_POINT ( 'NONE',  ( 26.75643035624999655, 242.3968750006145001, 3.323476615752267715 ) ) ;
#36013=ORIENTED_EDGE ( 'NONE', *, *, #6679, .F. ) ;
#36014=CARTESIAN_POINT ( 'NONE',  ( 15.24356964374999990, 247.9093750006145171, -3.323476615752268604 ) ) ;
#36021=VERTEX_POINT ( 'NONE', #31411 ) ;
#36026=CARTESIAN_POINT ( 'NONE',  ( 26.75643035624999655, 247.7218750006145171, -7.049594010296217766E-16 ) ) ;
#36027=CARTESIAN_POINT ( 'NONE',  ( -27.00000000000000355, 199.2125000012290457, 0.000000000000000000 ) ) ;
#36032=ORIENTED_EDGE ( 'NONE', *, *, #25579, .F. ) ;
#36042=ORIENTED_EDGE ( 'NONE', *, *, #28448, .F. ) ;
#36048=CARTESIAN_POINT ( 'NONE',  ( 13.62178482187501416, 198.6593750006145456, 23.59362340125806767 ) ) ;
#36050=DIRECTION ( 'NONE',  ( 0.000000000000000000, 0.000000000000000000, -1.000000000000000000 ) ) ;
#36055=CARTESIAN_POINT ( 'NONE',  ( 21.00000000000000000, 244.7687500012290513, 6.928203230275506996 ) ) ;
#36064=CARTESIAN_POINT ( 'NONE',  ( 23.87821517812499650, 243.7468750006145228, -4.985214923628404904 ) ) ;
#36069=DIRECTION ( 'NONE',  ( 0.000000000000000000, 0.000000000000000000, 1.000000000000000000 ) ) ;
#36077=FACE_OUTER_BOUND ( 'NONE', #13531, .T. ) ;
#36082=CARTESIAN_POINT ( 'NONE',  ( 15.00000000000000000, 244.1687500012290286, -3.464101615137752610 ) ) ;
#36087=CARTESIAN_POINT ( 'NONE',  ( -7.234628195640302017, 199.1924038105676686, 27.00000000000000711 ) ) ;
#36089=CARTESIAN_POINT ( 'NONE',  ( 20.99999999999999645, 185.0294372515228645, 0.000000000000000000 ) ) ;
#36093=CARTESIAN_POINT ( 'NONE',  ( 20.99999999999999645, 245.2468750006145797, -6.646953231504538984 ) ) ;
#36107=CARTESIAN_POINT ( 'NONE',  ( 10.49999999999999467, 222.9518338469886203, 2.500000000000000000 ) ) ;
#36109=CARTESIAN_POINT ( 'NONE',  ( 14.99999999999999822, 204.0000000000000284, -3.514718625761426019 ) ) ;
#36115=EDGE_CURVE ( 'NONE', #29774, #20600, #3299, .T. ) ;
#36116=CARTESIAN_POINT ( 'NONE',  ( 21.00000000000000000, 243.4187500012290002, 5.999999999999998224 ) ) ;
#36117=CARTESIAN_POINT ( 'NONE',  ( 20.60729646369923529, 211.0472094301353536, 5.999999999999996447 ) ) ;
#36125=CARTESIAN_POINT ( 'NONE',  ( -27.24356964374999635, 199.3906250006145342, 15.72908226750539384 ) ) ;
#36128=VECTOR ( 'NONE', #26095, 1000.000000000000000 ) ;
#36130=DIRECTION ( 'NONE',  ( 0.8660254037844187236, -0.5000000000000346390, 0.000000000000000000 ) ) ;
#36138=CARTESIAN_POINT ( 'NONE',  ( 15.00000000000000000, 246.4000000000000057, 0.000000000000000000 ) ) ;
#36142=CARTESIAN_POINT ( 'NONE',  ( 27.00000000000001066, 199.2875000000000227, 15.58845726811988897 ) ) ;
#36145=CARTESIAN_POINT ( 'NONE',  ( 13.49999999999999645, 198.6125000012290513, -23.38268590217984766 ) ) ;
#36146=EDGE_LOOP ( 'NONE', ( #25350, #25032, #4917, #27540, #23377, #24605 ) ) ;
#36150=CARTESIAN_POINT ( 'NONE',  ( 15.00000000000000000, 245.0124999999999602, -3.464101615137752166 ) ) ;
#36155=VERTEX_POINT ( 'NONE', #28553 ) ;
#36156=CARTESIAN_POINT ( 'NONE',  ( -1.909035429704832693E-15, 197.7500000012290400, -31.17691453623979214 ) ) ;
#36160=CARTESIAN_POINT ( 'NONE',  ( 15.24356964374999990, 246.2218750006145456, -3.323476615752268604 ) ) ;
#36167=CARTESIAN_POINT ( 'NONE',  ( 7.234628195640295800, 197.8825961894323484, 27.00000000000001066 ) ) ;
#36178=CARTESIAN_POINT ( 'NONE',  ( 18.00000000000000000, 248.1812500012290457, -5.196152422706630247 ) ) ;
#36182=CARTESIAN_POINT ( 'NONE',  ( 26.75643035624999655, 240.1093750006145342, -3.323476615752271712 ) ) ;
#36185=CIRCLE ( 'NONE', #19284, 2.649999999999990585 ) ;
#36187=CARTESIAN_POINT ( 'NONE',  ( -1.926257025242585782E-15, 197.9468750006145399, -31.45816453501076637 ) ) ;
#36189=CARTESIAN_POINT ( 'NONE',  ( 19.95811093400027403, 239.6067736145540152, -5.908846518073574750 ) ) ;
#36190=CARTESIAN_POINT ( 'NONE',  ( 23.87821517812500005, 243.2593750006145399, 4.985214923628404016 ) ) ;
#36194=VERTEX_POINT ( 'NONE', #14165 ) ;
#36195=CARTESIAN_POINT ( 'NONE',  ( 21.00000000000000000, 243.7843750006144887, -6.646953231504538984 ) ) ;
#36201=ORIENTED_EDGE ( 'NONE', *, *, #28836, .F. ) ;
#36210=CARTESIAN_POINT ( 'NONE',  ( 18.12178482187500350, 247.1218750006145228, 4.985214923628407568 ) ) ;
#36227=ORIENTED_EDGE ( 'NONE', *, *, #36458, .T. ) ;
#36228=CARTESIAN_POINT ( 'NONE',  ( 20.99999999999999645, 185.0294372515228645, 0.000000000000000000 ) ) ;
#36230=CARTESIAN_POINT ( 'NONE',  ( 20.99999999999999645, 185.0294372515228645, 0.000000000000000000 ) ) ;
#36233=CARTESIAN_POINT ( 'NONE',  ( -13.62178482187498396, 198.1343750006145399, 23.59362340125808188 ) ) ;
#36235=FACE_OUTER_BOUND ( 'NONE', #31438, .T. ) ;
#36238=VERTEX_POINT ( 'NONE', #8660 ) ;
#36239=CARTESIAN_POINT ( 'NONE',  ( 15.00000000000000178, 245.1437500012290513, 3.464101615137757051 ) ) ;
#36256=B_SPLINE_CURVE_WITH_KNOTS ( 'NONE', 3,
 ( #12067, #23449, #35185, #3351, #26282, #31422, #25731, #8671, #34448, #35002, #19880, #37282, #25917, #17024, #11330, #5627, #2603, #23642, #31602, #17769, #5819, #8489, #2976, #20433, #20058, #316, #28564, #17210, #9045, #28751, #20617, #2789, #34627, #14362, #14546, #20242, #37462, #11512 ),
 .UNSPECIFIED., .F., .F.,
 ( 4, 2, 2, 2, 2, 2, 2, 2, 2, 2, 2, 2, 2, 2, 2, 2, 2, 2, 4 ),
 ( 0.000000000000000000, 0.003347226634339490244, 0.006694453268678980488, 0.01004167990301847030, 0.01171529322018821477, 0.01338890653735796098, 0.02008335980603693019, 0.02175697312320667293, 0.02343058644037641566, 0.02677781307471589767, 0.03012503970905539008, 0.03179865302622512935, 0.03347226634339488249, 0.03681949297773436103, 0.04016671961207383262, 0.04686117288075281051, 0.04853478619792254978, 0.05020839951509228904, 0.05355562614943176064 ),
 .UNSPECIFIED. ) ;
#36258=CARTESIAN_POINT ( 'NONE',  ( -6.797732988389737052, 221.2600366402566010, -2.615528913832024127 ) ) ;
#36261=CARTESIAN_POINT ( 'NONE',  ( 20.99999999999999645, 185.0294372515228645, 0.000000000000000000 ) ) ;
#36265=ORIENTED_EDGE ( 'NONE', *, *, #2054, .F. ) ;
#36270=DIRECTION ( 'NONE',  ( -1.000000000000000000, -6.123233995736766036E-17, 0.000000000000000000 ) ) ;
#36273=CARTESIAN_POINT ( 'NONE',  ( 23.87821517812499650, 247.9093750006145171, -4.985214923628404904 ) ) ;
#36275=CARTESIAN_POINT ( 'NONE',  ( 15.24356964374999990, 244.9093750006145171, 0.000000000000000000 ) ) ;
#36287=ORIENTED_EDGE ( 'NONE', *, *, #34894, .F. ) ;
#36288=VERTEX_POINT ( 'NONE', #32516 ) ;
#36291=DIRECTION ( 'NONE',  ( 0.000000000000000000, 0.000000000000000000, -1.000000000000000000 ) ) ;
#36305=CARTESIAN_POINT ( 'NONE',  ( -27.24356964374999635, 197.1406250006145058, 15.72908226750539384 ) ) ;
#36309=CARTESIAN_POINT ( 'NONE',  ( -27.12178482187499995, 199.7328125009217956, 0.000000000000000000 ) ) ;
#36329=EDGE_CURVE ( 'NONE', #6323, #10609, #20041, .T. ) ;
#36334=CARTESIAN_POINT ( 'NONE',  ( 26.99999999999999645, 247.1125000000000114, -3.464101615137755275 ) ) ;
#36335=DIRECTION ( 'NONE',  ( 1.000000000000000000, 0.000000000000000000, 0.000000000000000000 ) ) ;
#36338=ORIENTED_EDGE ( 'NONE', *, *, #28562, .T. ) ;
#36341=CARTESIAN_POINT ( 'NONE',  ( 27.00000000000001066, 197.6000000012290627, 15.58845726811988897 ) ) ;
#36345=CARTESIAN_POINT ( 'NONE',  ( 21.00000000000000000, 245.9218750006145058, 6.646953231504538984 ) ) ;
#36348=DIRECTION ( 'NONE',  ( -1.000000000000000000, 0.000000000000000000, -0.000000000000000000 ) ) ;
#36352=CARTESIAN_POINT ( 'NONE',  ( -1.926257025242585782E-15, 199.2968750006145342, -31.45816453501075927 ) ) ;
#36354=EDGE_CURVE ( 'NONE', #12534, #2167, #32859, .T. ) ;
#36357=FACE_OUTER_BOUND ( 'NONE', #9308, .T. ) ;
#36364=LINE ( 'NONE', #10412, #17680 ) ;
#36368=CARTESIAN_POINT ( 'NONE',  ( 21.00000000000000000, 239.9593750006145001, 6.646953231504538984 ) ) ;
#36369=CIRCLE ( 'NONE', #647, 7.500000000000000000 ) ;
#36373=CARTESIAN_POINT ( 'NONE',  ( -27.24356964375000345, 198.9218750006145626, -15.72908226750537786 ) ) ;
#36376=CARTESIAN_POINT ( 'NONE',  ( 15.24356964374999990, 242.2093750006145285, 0.000000000000000000 ) ) ;
#36381=ORIENTED_EDGE ( 'NONE', *, *, #18282, .F. ) ;
#36382=CARTESIAN_POINT ( 'NONE',  ( 18.12178482187500350, 245.7718750006145001, 4.985214923628407568 ) ) ;
#36386=( BOUNDED_CURVE ( )  B_SPLINE_CURVE ( 2, ( #21425, #24446, #18587, #15542, #30129, #9477, #4161, #35994, #3406 ),
 .UNSPECIFIED., .F., .F. ) 
 B_SPLINE_CURVE_WITH_KNOTS ( ( 3, 2, 2, 2, 3 ),
 ( 0.5543478260869565410, 0.5579710144927536586, 0.5652173913043477826, 0.5724637681159420177, 0.5760869565217391353 ),
 .UNSPECIFIED. ) 
 CURVE ( )  GEOMETRIC_REPRESENTATION_ITEM ( )  RATIONAL_B_SPLINE_CURVE ( ( 0.9330127018922194093, 0.9330127018922194093, 1.000000000000000000, 0.8660254037844387076, 1.000000000000000000, 0.8660254037844387076, 1.000000000000000000, 0.9330127018922194093, 0.9330127018922194093 ) ) 
 REPRESENTATION_ITEM ( '' )  );
#36396=CARTESIAN_POINT ( 'NONE',  ( 23.87821517812500005, 245.8468750006145171, 4.985214923628404016 ) ) ;
#36401=ORIENTED_EDGE ( 'NONE', *, *, #13141, .F. ) ;
#36402=( BOUNDED_CURVE ( )  B_SPLINE_CURVE ( 2, ( #32817, #20707, #35658, #23734, #32250, #12735, #15395, #3255, #4008 ),
 .UNSPECIFIED., .F., .F. ) 
 B_SPLINE_CURVE_WITH_KNOTS ( ( 3, 2, 2, 2, 3 ),
 ( 0.1413043478260869457, 0.1449275362318840632, 0.1521739130434782705, 0.1594202898550724501, 0.1630434782608695676 ),
 .UNSPECIFIED. ) 
 CURVE ( )  GEOMETRIC_REPRESENTATION_ITEM ( )  RATIONAL_B_SPLINE_CURVE ( ( 0.9330127018922194093, 0.9330127018922190762, 1.000000000000000000, 0.8660254037844387076, 1.000000000000000000, 0.8660254037844387076, 1.000000000000000000, 0.9330127018922190762, 0.9330127018922194093 ) ) 
 REPRESENTATION_ITEM ( '' )  );
#36406=CARTESIAN_POINT ( 'NONE',  ( 22.60769515458671108, 242.5388461906613600, 6.000000000000010658 ) ) ;
#36416=CARTESIAN_POINT ( 'NONE',  ( 27.24356964374999635, 198.3218750006145399, -15.72908226750539029 ) ) ;
#36423=CARTESIAN_POINT ( 'NONE',  ( 21.00000000000000000, 241.3937500012290229, -6.928203230275506996 ) ) ;
#36426=CARTESIAN_POINT ( 'NONE',  ( -27.24356964374999635, 198.4906250006145569, 15.72908226750539384 ) ) ;
#36446=DIRECTION ( 'NONE',  ( -0.000000000000000000, 1.000000000000000000, -0.000000000000000000 ) ) ;
#36451=CARTESIAN_POINT ( 'NONE',  ( 15.00000000000000178, 244.2437500012290457, 3.464101615137757051 ) ) ;
#36454=CARTESIAN_POINT ( 'NONE',  ( -13.49999999999998401, 196.1375000012290286, 23.38268590217985476 ) ) ;
#36456=CARTESIAN_POINT ( 'NONE',  ( -29.00000000000002487, 210.0000000000000000, 0.000000000000000000 ) ) ;
#36457=CARTESIAN_POINT ( 'NONE',  ( 1.120210788295102201E-13, 195.5000000012290400, -27.00000000000000711 ) ) ;
#36458=EDGE_CURVE ( 'NONE', #22517, #14644, #4751, .T. ) ;
#36460=CARTESIAN_POINT ( 'NONE',  ( 18.12178482187500350, 247.6843750006145228, 4.985214923628407568 ) ) ;
#36462=CARTESIAN_POINT ( 'NONE',  ( 26.75643035624999655, 243.7843750006145456, -7.049594010296217766E-16 ) ) ;
#36471=AXIS2_PLACEMENT_3D ( 'NONE', #27618, #30472, #21386 ) ;
#36480=CARTESIAN_POINT ( 'NONE',  ( 26.75643035624999655, 249.5593750006145228, -3.323476615752271712 ) ) ;
#36484=CARTESIAN_POINT ( 'NONE',  ( 5.536961926790850086, 215.7986392774537308, -1.553813268097582245 ) ) ;
#36486=CARTESIAN_POINT ( 'NONE',  ( 20.99999999999999645, 185.0294372515228645, 0.000000000000000000 ) ) ;
#36493=CARTESIAN_POINT ( 'NONE',  ( 5.778771075727756162E-15, 195.4156250006145399, 31.45816453501075927 ) ) ;
#36497=ORIENTED_EDGE ( 'NONE', *, *, #23618, .T. ) ;
#36512=CARTESIAN_POINT ( 'NONE',  ( -27.00000000000000355, 199.5500000000000114, 0.000000000000000000 ) ) ;
#36521=CARTESIAN_POINT ( 'NONE',  ( 26.99999999999999645, 242.9874999999999829, 3.464101615137751278 ) ) ;
#36527=VERTEX_POINT ( 'NONE', #7687 ) ;
#36528=CARTESIAN_POINT ( 'NONE',  ( -13.50000000000000533, 197.3375000012290457, -23.38268590217984411 ) ) ;
#36529=CARTESIAN_POINT ( 'NONE',  ( -27.00000000000000355, 196.8500000000000227, 0.000000000000000000 ) ) ;
#36532=CARTESIAN_POINT ( 'NONE',  ( 23.87821517812499650, 243.4093750006145171, -4.985214923628404904 ) ) ;
#36535=LINE ( 'NONE', #30682, #2228 ) ;
#36540=CARTESIAN_POINT ( 'NONE',  ( 13.62178482187501416, 199.5593750006145513, 23.59362340125806767 ) ) ;
#36559=CARTESIAN_POINT ( 'NONE',  ( 13.62178482187499640, 198.3593750006145342, -23.59362340125807123 ) ) ;
#36563=CARTESIAN_POINT ( 'NONE',  ( 15.24356964374999990, 242.6218750006145228, -3.323476615752268604 ) ) ;
#36564=DIRECTION ( 'NONE',  ( -0.000000000000000000, 1.000000000000000000, -0.000000000000000000 ) ) ;
#36568=VERTEX_POINT ( 'NONE', #24742 ) ;
#36570=CARTESIAN_POINT ( 'NONE',  ( 15.24356964375000167, 244.8343750006145285, 3.323476615752272600 ) ) ;
#36579=ORIENTED_EDGE ( 'NONE', *, *, #11717, .F. ) ;
#36583=EDGE_CURVE ( 'NONE', #2189, #18678, #13560, .T. ) ;
#36585=CARTESIAN_POINT ( 'NONE',  ( 23.87821517812499650, 243.2968750006145058, -4.985214923628404904 ) ) ;
#36587=CARTESIAN_POINT ( 'NONE',  ( -13.50000000000000533, 197.3375000012290457, -23.38268590217984411 ) ) ;
#36591=ORIENTED_EDGE ( 'NONE', *, *, #414, .T. ) ;
#36593=CARTESIAN_POINT ( 'NONE',  ( -13.49999999999998401, 199.6250000000000284, 23.38268590217985476 ) ) ;
#36599=CYLINDRICAL_SURFACE ( 'NONE', #3400, 8.000000000000000000 ) ;
#36603=( BOUNDED_CURVE ( )  B_SPLINE_CURVE ( 2, ( #35377, #34820, #8863, #20624, #21005, #9053, #29510, #17776, #6394 ),
 .UNSPECIFIED., .F., .F. ) 
 B_SPLINE_CURVE_WITH_KNOTS ( ( 3, 2, 2, 2, 3 ),
 ( 0.1875000000000000000, 0.1944444444444444475, 0.2083333333333333426, 0.2222222222222222099, 0.2291666666666666574 ),
 .UNSPECIFIED. ) 
 CURVE ( )  GEOMETRIC_REPRESENTATION_ITEM ( )  RATIONAL_B_SPLINE_CURVE ( ( 0.9330127018922194093, 0.9330127018922194093, 1.000000000000000000, 0.8660254037844387076, 1.000000000000000000, 0.8660254037844387076, 1.000000000000000000, 0.9330127018922194093, 0.9330127018922194093 ) ) 
 REPRESENTATION_ITEM ( '' )  );
#36605=CARTESIAN_POINT ( 'NONE',  ( -13.62178482187498396, 199.0343750006145456, 23.59362340125808188 ) ) ;
#36607=CARTESIAN_POINT ( 'NONE',  ( 21.00000000000000000, 243.8125000000000284, 5.999999999999998224 ) ) ;
#36609=DIRECTION ( 'NONE',  ( 0.000000000000000000, 0.000000000000000000, -1.000000000000000000 ) ) ;
#36610=ORIENTED_EDGE ( 'NONE', *, *, #13192, .T. ) ;
#36611=CARTESIAN_POINT ( 'NONE',  ( 15.00000000000000000, 241.0187500012290513, -3.464101615137752166 ) ) ;
#36614=CARTESIAN_POINT ( 'NONE',  ( -27.24356964374999990, 197.9656250006145228, -15.72908226750537786 ) ) ;
#36640=CARTESIAN_POINT ( 'NONE',  ( -28.09666271755782674, 206.4427866876137045, -7.184768031510477826 ) ) ;
#36643=CIRCLE ( 'NONE', #10027, 7.500000000000000000 ) ;
#36644=CARTESIAN_POINT ( 'NONE',  ( -7.234628195640316228, 195.9700961906613372, -27.00000000000000000 ) ) ;
#36651=CARTESIAN_POINT ( 'NONE',  ( 15.24356964374999990, 248.0593750006145228, 0.000000000000000000 ) ) ;
#36653=CARTESIAN_POINT ( 'NONE',  ( 15.24356964374999990, 241.2718750006145001, -3.323476615752268604 ) ) ;
#36657=FACE_OUTER_BOUND ( 'NONE', #31929, .T. ) ;
#36661=CARTESIAN_POINT ( 'NONE',  ( 23.99999999999999645, 240.9062500012290684, -5.196152422706631135 ) ) ;
#36666=ORIENTED_EDGE ( 'NONE', *, *, #15755, .F. ) ;
#36669=CARTESIAN_POINT ( 'NONE',  ( 20.99999999999999289, 249.4937500012290457, -5.999999999999998224 ) ) ;
#36672=CARTESIAN_POINT ( 'NONE',  ( 15.24356964374999990, 248.8093750006144944, -3.323476615752268604 ) ) ;
#36676=CARTESIAN_POINT ( 'NONE',  ( 14.06542688029398036, 216.9345731196990243, -0.01200585064250309433 ) ) ;
#36678=CYLINDRICAL_SURFACE ( 'NONE', #22662, 5.999999999999999112 ) ;
#36684=CARTESIAN_POINT ( 'NONE',  ( -13.62178482187500528, 197.0281250006145228, -23.59362340125807123 ) ) ;
#36687=EDGE_LOOP ( 'NONE', ( #14875, #16508, #18699, #30883, #959 ) ) ;
#36699=EDGE_CURVE ( 'NONE', #6323, #9298, #33090, .T. ) ;
#36702=CARTESIAN_POINT ( 'NONE',  ( 26.99999999999999645, 198.9124999999999943, -15.58845726811990495 ) ) ;
#36703=DIRECTION ( 'NONE',  ( -0.000000000000000000, 1.000000000000000000, -0.000000000000000000 ) ) ;
#36706=CARTESIAN_POINT ( 'NONE',  ( 1.069080835302379631E-14, 198.4250000012290229, 27.00000000000000000 ) ) ;
#36713=CARTESIAN_POINT ( 'NONE',  ( 24.00000000000000000, 244.7500000000000000, 5.196152422706629359 ) ) ;
#36719=CARTESIAN_POINT ( 'NONE',  ( 13.49999999999999645, 198.1625000012290343, -23.38268590217984766 ) ) ;
#36720=CARTESIAN_POINT ( 'NONE',  ( 1.069080835302379631E-14, 196.9624999999999773, 27.00000000000000000 ) ) ;
#36723=CARTESIAN_POINT ( 'NONE',  ( 18.12178482187500350, 243.1843750006145513, 4.985214923628407568 ) ) ;
#36730=CARTESIAN_POINT ( 'NONE',  ( -13.62178482187498396, 197.6843750006145228, 23.59362340125808188 ) ) ;
#36745=CARTESIAN_POINT ( 'NONE',  ( 20.99999999999999289, 240.4937500012290457, -5.999999999999997335 ) ) ;
#36750=CARTESIAN_POINT ( 'NONE',  ( 5.778771075727756162E-15, 197.7218750006145456, 31.45816453501076637 ) ) ;
#36753=CARTESIAN_POINT ( 'NONE',  ( 15.00000000000000178, 239.7437500012290457, 3.464101615137757051 ) ) ;
#36754=CARTESIAN_POINT ( 'NONE',  ( 15.00000000000000000, 250.0000000000000000, 0.000000000000000000 ) ) ;
#36755=CARTESIAN_POINT ( 'NONE',  ( 20.99999999999999645, 185.0294372515228645, 0.000000000000000000 ) ) ;
#36760=CARTESIAN_POINT ( 'NONE',  ( 21.00000000000000000, 245.5843750006145569, -6.646953231504538984 ) ) ;
#36764=CARTESIAN_POINT ( 'NONE',  ( -1.045839947578415010E-13, 196.5125000000000455, 27.00000000000000355 ) ) ;
#36771=CARTESIAN_POINT ( 'NONE',  ( 26.75643035624999655, 244.5343750006144887, 3.323476615752267271 ) ) ;
#36776=DIRECTION ( 'NONE',  ( 0.000000000000000000, 0.000000000000000000, -1.000000000000000000 ) ) ;
#36784=CYLINDRICAL_SURFACE ( 'NONE', #25774, 5.999999999999999112 ) ;
#36790=CARTESIAN_POINT ( 'NONE',  ( 27.24356964375000345, 198.7343750006145626, -3.336375036156643733E-15 ) ) ;
#36796=ORIENTED_EDGE ( 'NONE', *, *, #31483, .T. ) ;
#36797=CARTESIAN_POINT ( 'NONE',  ( 21.00000000000000000, 241.6187500012291025, 6.928203230275506996 ) ) ;
#36800=CARTESIAN_POINT ( 'NONE',  ( -27.24356964375000345, 198.0031250006145456, 0.000000000000000000 ) ) ;
#36818=CARTESIAN_POINT ( 'NONE',  ( -12.42035509746875022, 216.7950050350868310, -4.614743948463994272 ) ) ;
#36834=CARTESIAN_POINT ( 'NONE',  ( 15.24356964374999990, 247.1218750006145228, -3.323476615752268604 ) ) ;
#36836=CARTESIAN_POINT ( 'NONE',  ( 15.24356964374999990, 242.1718750006145058, -3.323476615752268604 ) ) ;
#36839=CARTESIAN_POINT ( 'NONE',  ( 15.00000000000000000, 249.6062500012290570, 0.000000000000000000 ) ) ;
#36840=CARTESIAN_POINT ( 'NONE',  ( 24.00000000000000000, 249.3062500012290457, 5.196152422706629359 ) ) ;
#36853=CARTESIAN_POINT ( 'NONE',  ( 15.24356964374999990, 249.2968750006145058, 0.000000000000000000 ) ) ;
#36856=CARTESIAN_POINT ( 'NONE',  ( 15.15359421270862050, 225.5904154327813842, -1.363118671455028297 ) ) ;
#36858=DIRECTION ( 'NONE',  ( 0.000000000000000000, 0.000000000000000000, 1.000000000000000000 ) ) ;
#36864=CARTESIAN_POINT ( 'NONE',  ( -13.62178482187500528, 196.1281250006145171, -23.59362340125807123 ) ) ;
#36868=CARTESIAN_POINT ( 'NONE',  ( 21.00000000000000000, 249.0437500012290570, -5.999999999999998224 ) ) ;
#36879=CARTESIAN_POINT ( 'NONE',  ( 20.99999999999999645, 250.0000000000000000, 8.000000000000000000 ) ) ;
#36881=CARTESIAN_POINT ( 'NONE',  ( -27.00000000000000355, 197.2624999999999886, -15.58845726811989429 ) ) ;
#36885=CARTESIAN_POINT ( 'NONE',  ( 26.75643035624999655, 249.6343750006145399, -7.049594010296217766E-16 ) ) ;
#36893=CARTESIAN_POINT ( 'NONE',  ( 21.00000000000000000, 243.8124999999999716, 6.928203230275506996 ) ) ;
#36896=ORIENTED_EDGE ( 'NONE', *, *, #21200, .F. ) ;
#36897=CARTESIAN_POINT ( 'NONE',  ( -13.50000000000000533, 196.8875000012290286, -23.38268590217984411 ) ) ;
#36898=CARTESIAN_POINT ( 'NONE',  ( 20.99999999999999645, 185.0294372515228645, 0.000000000000000000 ) ) ;
#36901=CARTESIAN_POINT ( 'NONE',  ( 15.24356964374999990, 242.1718750006145342, -3.323476615752268604 ) ) ;
#36905=ADVANCED_FACE ( 'NONE', ( #23721 ), #22468, .F. ) ;
#36908=CARTESIAN_POINT ( 'NONE',  ( 5.778771075727756162E-15, 198.1718750006145342, 31.45816453501075927 ) ) ;
#36928=ADVANCED_FACE ( 'NONE', ( #3242 ), #26549, .F. ) ;
#36929=CARTESIAN_POINT ( 'NONE',  ( -27.24356964375000345, 196.6718750006145342, -15.72908226750537786 ) ) ;
#36931=( BOUNDED_CURVE ( )  B_SPLINE_CURVE ( 3, ( #23511, #7576, #7024, #21431 ),
 .UNSPECIFIED., .F., .F. ) 
 B_SPLINE_CURVE_WITH_KNOTS ( ( 4, 4 ),
 ( 1.224646799147353454E-16, 1.570796326794895448 ),
 .UNSPECIFIED. ) 
 CURVE ( )  GEOMETRIC_REPRESENTATION_ITEM ( )  RATIONAL_B_SPLINE_CURVE ( ( 1.000000000000000000, 0.8047378541243652705, 0.8047378541243652705, 1.000000000000000000 ) ) 
 REPRESENTATION_ITEM ( '' )  );
#36933=DIRECTION ( 'NONE',  ( 0.000000000000000000, 0.000000000000000000, -1.000000000000000000 ) ) ;
#36934=CARTESIAN_POINT ( 'NONE',  ( 23.87821517812499650, 240.2593750006145399, -4.985214923628404904 ) ) ;
#36935=EDGE_CURVE ( 'NONE', #2167, #12999, #22706, .T. ) ;
#36941=CARTESIAN_POINT ( 'NONE',  ( 26.75643035624999655, 244.1593750006145171, -3.323476615752271712 ) ) ;
#36942=DIRECTION ( 'NONE',  ( -0.000000000000000000, -1.000000000000000000, -0.000000000000000000 ) ) ;
#36953=CARTESIAN_POINT ( 'NONE',  ( 26.75643035624999655, 244.5718750006145115, -7.049594010296217766E-16 ) ) ;
#36954=CARTESIAN_POINT ( 'NONE',  ( 20.99999999999999289, 240.4374999999999716, -5.999999999999997335 ) ) ;
#36959=ADVANCED_FACE ( 'NONE', ( #2363 ), #14815, .T. ) ;
#36978=CARTESIAN_POINT ( 'NONE',  ( -27.24356964374999635, 195.8468750006145171, 15.72908226750539384 ) ) ;
#36984=CARTESIAN_POINT ( 'NONE',  ( 18.00000000000000000, 242.3312500012290513, -5.196152422706630247 ) ) ;
#36989=VECTOR ( 'NONE', #3029, 1000.000000000000000 ) ;
#36995=CARTESIAN_POINT ( 'NONE',  ( 20.99999999999999645, 185.0294372515228645, 5.999999999999999112 ) ) ;
#37010=CARTESIAN_POINT ( 'NONE',  ( 18.00000000000000355, 247.8812500012290343, 5.196152422706632912 ) ) ;
#37018=CARTESIAN_POINT ( 'NONE',  ( 26.75643035624999655, 248.7718750006145569, -3.323476615752271712 ) ) ;
#37020=CARTESIAN_POINT ( 'NONE',  ( 15.24356964374999990, 242.2093750006145285, 0.000000000000000000 ) ) ;
#37021=ORIENTED_EDGE ( 'NONE', *, *, #17731, .T. ) ;
#37024=CARTESIAN_POINT ( 'NONE',  ( 26.99999999999999645, 248.9312500012290457, -7.347880794884117764E-16 ) ) ;
#37041=CARTESIAN_POINT ( 'NONE',  ( 14.97710761593534556, 216.0228923840610094, -0.2612666680235000150 ) ) ;
#37044=CARTESIAN_POINT ( 'NONE',  ( 27.00000000000000355, 197.0749999999999886, -3.306546357697854128E-15 ) ) ;
#37049=ADVANCED_FACE ( 'NONE', ( #1147, #18613 ), #9871, .F. ) ;
#37051=CARTESIAN_POINT ( 'NONE',  ( 27.24356964374999635, 195.1156250006145001, -15.72908226750539029 ) ) ;
#37055=VERTEX_POINT ( 'NONE', #35643 ) ;
#37068=CARTESIAN_POINT ( 'NONE',  ( 27.00000000000000355, 197.5250000000000057, -3.306546357697854128E-15 ) ) ;
#37080=CARTESIAN_POINT ( 'NONE',  ( 26.99999999999999645, 243.0625000000000284, -3.464101615137755275 ) ) ;
#37084=EDGE_LOOP ( 'NONE', ( #26931, #37449, #36381, #37299 ) ) ;
#37085=CARTESIAN_POINT ( 'NONE',  ( 5.727106289114498080E-15, 196.6250000012290400, 31.17691453623979214 ) ) ;
#37089=CARTESIAN_POINT ( 'NONE',  ( 15.24356964375000167, 243.1468750006145285, 3.323476615752272600 ) ) ;
#37097=CARTESIAN_POINT ( 'NONE',  ( -27.24356964374999990, 198.4718750006145171, -15.72908226750537786 ) ) ;
#37101=EDGE_CURVE ( 'NONE', #16873, #24643, #13499, .T. ) ;
#37111=CARTESIAN_POINT ( 'NONE',  ( 1.120210788295102201E-13, 195.0500000012290798, -27.00000000000000711 ) ) ;
#37116=CARTESIAN_POINT ( 'NONE',  ( 27.00000000000001421, 196.1375000000000171, 15.58845726811988897 ) ) ;
#37120=CARTESIAN_POINT ( 'NONE',  ( 21.00000000000000000, 240.5218750006145285, 6.646953231504538984 ) ) ;
#37121=CARTESIAN_POINT ( 'NONE',  ( -13.62178482187498396, 198.9781250006145399, 23.59362340125808188 ) ) ;
#37125=EDGE_CURVE ( 'NONE', #17695, #8916, #637, .T. ) ;
#37127=ORIENTED_EDGE ( 'NONE', *, *, #33864, .F. ) ;
#37128=CARTESIAN_POINT ( 'NONE',  ( 26.75643035624999655, 241.8718750006145228, -7.049594010296217766E-16 ) ) ;
#37129=CARTESIAN_POINT ( 'NONE',  ( 0.000000000000000000, 210.0000000000000284, -27.00000000000000000 ) ) ;
#37133=B_SPLINE_CURVE_WITH_KNOTS ( 'NONE', 3,
 ( #223, #28290, #19965, #11788, #23356, #2329, #31508, #22987, #17866, #9704, #26374, #21281, #14830, #32440, #29978, #21091, #32631, #24302, #6668, #29411, #3442, #29598, #6484, #9519 ),
 .UNSPECIFIED., .F., .F.,
 ( 4, 2, 2, 2, 2, 2, 2, 2, 2, 2, 2, 4 ),
 ( 0.01257025459185682689, 0.01413966516175825527, 0.01570907573165968366, 0.01649378101661039958, 0.01727848630156111204, 0.01806319158651182449, 0.01884789687146253695, 0.02041730744136390635, 0.02198671801126527575, 0.02355612858116664515, 0.02434083386611728822, 0.02512553915106793476 ),
 .UNSPECIFIED. ) ;
#37141=CARTESIAN_POINT ( 'NONE',  ( 15.24356964374999990, 243.4093750006145171, -3.323476615752268604 ) ) ;
#37148=LINE ( 'NONE', #37327, #7647 ) ;
#37152=( BOUNDED_CURVE ( )  B_SPLINE_CURVE ( 2, ( #22539, #15257, #34086, #2938, #10965, #9196, #26619, #26810, #649 ),
 .UNSPECIFIED., .F., .F. ) 
 B_SPLINE_CURVE_WITH_KNOTS ( ( 3, 2, 2, 2, 3 ),
 ( 0.2282608695652173780, 0.2318840579710144956, 0.2391304347826087029, 0.2463768115942029102, 0.2500000000000000000 ),
 .UNSPECIFIED. ) 
 CURVE ( )  GEOMETRIC_REPRESENTATION_ITEM ( )  RATIONAL_B_SPLINE_CURVE ( ( 0.9330127018922194093, 0.9330127018922190762, 1.000000000000000000, 0.8660254037844387076, 1.000000000000000000, 0.8660254037844387076, 1.000000000000000000, 0.9330127018922196314, 0.9330127018922194093 ) ) 
 REPRESENTATION_ITEM ( '' )  );
#37153=CARTESIAN_POINT ( 'NONE',  ( 18.00000000000000355, 241.5812500012290513, 5.196152422706632912 ) ) ;
#37158=CARTESIAN_POINT ( 'NONE',  ( 20.99999999999999289, 244.9374999999999716, -5.999999999999997335 ) ) ;
#37165=CARTESIAN_POINT ( 'NONE',  ( -27.24356964374999990, 196.2218750006145456, -15.72908226750537786 ) ) ;
#37171=CARTESIAN_POINT ( 'NONE',  ( 26.99999999999999645, 240.7937500012290570, 3.464101615137751278 ) ) ;
#37177=VERTEX_POINT ( 'NONE', #14749 ) ;
#37187=ORIENTED_EDGE ( 'NONE', *, *, #22705, .T. ) ;
#37202=CARTESIAN_POINT ( 'NONE',  ( 20.99999999999999289, 240.0437500012290570, -5.999999999999997335 ) ) ;
#37203=CARTESIAN_POINT ( 'NONE',  ( 15.24356964374999990, 245.3593750006145342, 0.000000000000000000 ) ) ;
#37205=CARTESIAN_POINT ( 'NONE',  ( 18.12178482187499640, 241.2343750006145342, -4.985214923628404904 ) ) ;
#37209=CARTESIAN_POINT ( 'NONE',  ( 18.00000000000000000, 247.7312500012290570, -5.196152422706630247 ) ) ;
#37211=ADVANCED_FACE ( 'NONE', ( #26113 ), #23464, .F. ) ;
#37219=CIRCLE ( 'NONE', #3350, 10.00000000000000888 ) ;
#37226=CARTESIAN_POINT ( 'NONE',  ( 26.75643035624999655, 249.0718750006145115, -7.049594010296217766E-16 ) ) ;
#37229=CARTESIAN_POINT ( 'NONE',  ( 5.025722718613374163, 215.9903539805198420, 0.3926987779610276452 ) ) ;
#37239=ORIENTED_EDGE ( 'NONE', *, *, #9691, .F. ) ;
#37254=CARTESIAN_POINT ( 'NONE',  ( 27.00000000000001066, 198.8374999999999773, 15.58845726811988897 ) ) ;
#37257=CARTESIAN_POINT ( 'NONE',  ( 18.12178482187499640, 249.3343750006145285, -4.985214923628404904 ) ) ;
#37261=EDGE_CURVE ( 'NONE', #21774, #1338, #28000, .T. ) ;
#37265=CARTESIAN_POINT ( 'NONE',  ( 15.00000000000000000, 244.6000000000000227, 0.000000000000000000 ) ) ;
#37266=CARTESIAN_POINT ( 'NONE',  ( 20.99999999999999289, 240.0437500012290570, -5.999999999999997335 ) ) ;
#37271=CARTESIAN_POINT ( 'NONE',  ( 5.727106289114498080E-15, 197.0750000012290570, 31.17691453623979214 ) ) ;
#37276=CARTESIAN_POINT ( 'NONE',  ( 15.24356964374999990, 241.7593750006145399, 0.000000000000000000 ) ) ;
#37278=DIRECTION ( 'NONE',  ( -0.000000000000000000, -0.000000000000000000, 1.000000000000000000 ) ) ;
#37282=CARTESIAN_POINT ( 'NONE',  ( 26.03202072822279334, 194.9999999999999716, -7.760941349413962520 ) ) ;
#37283=CARTESIAN_POINT ( 'NONE',  ( -27.24356964374999990, 197.1218750006145228, -15.72908226750537786 ) ) ;
#37286=ORIENTED_EDGE ( 'NONE', *, *, #35805, .F. ) ;
#37293=CARTESIAN_POINT ( 'NONE',  ( -4.500000000000002665, 244.5000000000000000, 2.500000000000000000 ) ) ;
#37299=ORIENTED_EDGE ( 'NONE', *, *, #1973, .F. ) ;
#37302=CARTESIAN_POINT ( 'NONE',  ( -13.62178482187500528, 195.7343750006145626, -23.59362340125807123 ) ) ;
#37306=CARTESIAN_POINT ( 'NONE',  ( 15.24356964375000167, 241.3468750006145456, 3.323476615752272600 ) ) ;
#37307=CARTESIAN_POINT ( 'NONE',  ( -13.62178482187500528, 197.4781250006145399, -23.59362340125807123 ) ) ;
#37310=VERTEX_POINT ( 'NONE', #26482 ) ;
#37312=CARTESIAN_POINT ( 'NONE',  ( 21.00000000000000000, 242.2093750006145285, 6.646953231504538984 ) ) ;
#37321=CARTESIAN_POINT ( 'NONE',  ( 20.99999999999999645, 245.1343750006145115, -6.646953231504538984 ) ) ;
#37327=CARTESIAN_POINT ( 'NONE',  ( 3.306546357697853733E-15, 210.0000000000000284, 27.00000000000000000 ) ) ;
#37332=CARTESIAN_POINT ( 'NONE',  ( 21.00000000000000000, 241.6187500012290457, 5.999999999999998224 ) ) ;
#37341=CARTESIAN_POINT ( 'NONE',  ( 5.778771075727756162E-15, 196.3718750006145513, 31.45816453501075927 ) ) ;
#37342=CARTESIAN_POINT ( 'NONE',  ( -7.102382295725191419, 195.0000000000001137, 26.31627238379491374 ) ) ;
#37343=LINE ( 'NONE', #11393, #30286 ) ;
#37348=CARTESIAN_POINT ( 'NONE',  ( 15.00000000000000000, 239.6687500012290570, -3.464101615137752166 ) ) ;
#37355=CIRCLE ( 'NONE', #34116, 8.000000000000000000 ) ;
#37356=CARTESIAN_POINT ( 'NONE',  ( 0.000000000000000000, 210.0000000000000284, 0.000000000000000000 ) ) ;
#37368=CARTESIAN_POINT ( 'NONE',  ( 20.99999999999997868, 210.0000000000000000, -5.999999999999999112 ) ) ;
#37376=ORIENTED_EDGE ( 'NONE', *, *, #29096, .T. ) ;
#37383=CARTESIAN_POINT ( 'NONE',  ( 18.12178482187499640, 245.2843750006145456, -4.985214923628404904 ) ) ;
#37385=CARTESIAN_POINT ( 'NONE',  ( 18.12178482187499640, 240.7843750006145171, -4.985214923628404904 ) ) ;
#37386=VECTOR ( 'NONE', #947, 1000.000000000000000 ) ;
#37391=CARTESIAN_POINT ( 'NONE',  ( 26.99999999999999645, 245.2937500012290570, 3.464101615137751278 ) ) ;
#37401=ORIENTED_EDGE ( 'NONE', *, *, #18000, .F. ) ;
#37404=CARTESIAN_POINT ( 'NONE',  ( 18.00000000000000000, 241.8812500012290343, -5.196152422706630247 ) ) ;
#37405=CARTESIAN_POINT ( 'NONE',  ( 26.75643035624999655, 245.9218750006145342, -7.049594010296217766E-16 ) ) ;
#37420=ADVANCED_FACE ( 'NONE', ( #25306 ), #36678, .F. ) ;
#37422=DIRECTION ( 'NONE',  ( 0.000000000000000000, 0.000000000000000000, 1.000000000000000000 ) ) ;
#37428=ADVANCED_FACE ( 'NONE', ( #13196 ), #16787, .F. ) ;
#37434=CARTESIAN_POINT ( 'NONE',  ( -27.00000000000000355, 196.8125000000000000, -15.58845726811989429 ) ) ;
#37435=VECTOR ( 'NONE', #26474, 1000.000000000000000 ) ;
#37438=CARTESIAN_POINT ( 'NONE',  ( 18.12178482187499640, 248.8843750006145399, -4.985214923628404904 ) ) ;
#37445=CARTESIAN_POINT ( 'NONE',  ( 15.00000000000000178, 240.5875000000000057, 3.464101615137757051 ) ) ;
#37446=CARTESIAN_POINT ( 'NONE',  ( 1.069080835302379631E-14, 198.7624999999999886, 27.00000000000000000 ) ) ;
#37448=EDGE_LOOP ( 'NONE', ( #14111, #28189, #33396, #10515 ) ) ;
#37449=ORIENTED_EDGE ( 'NONE', *, *, #30955, .T. ) ;
#37451=CARTESIAN_POINT ( 'NONE',  ( -27.00000000000000355, 195.5750000012290286, -15.58845726811989429 ) ) ;
#37452=CARTESIAN_POINT ( 'NONE',  ( -26.99999999999999645, 196.5500000012290513, 15.58845726811991561 ) ) ;
#37455=CARTESIAN_POINT ( 'NONE',  ( 20.99999999999997868, 246.0625000000000284, 5.999999999999999112 ) ) ;
#37457=CARTESIAN_POINT ( 'NONE',  ( 15.00000000000000178, 242.8937500012290229, 3.464101615137757051 ) ) ;
#37462=CARTESIAN_POINT ( 'NONE',  ( 13.47611835081543141, 194.9999999999999716, 23.69796585698624014 ) ) ;
#37463=CARTESIAN_POINT ( 'NONE',  ( -27.24356964374999990, 195.7718750006145569, -15.72908226750537786 ) ) ;
#37465=EDGE_CURVE ( 'NONE', #11399, #36527, #27965, .T. ) ;
#37468=DIRECTION ( 'NONE',  ( 0.000000000000000000, 0.000000000000000000, -1.000000000000000000 ) ) ;
#37470=EDGE_CURVE ( 'NONE', #21628, #26422, #31187, .T. ) ;
#37477=DIRECTION ( 'NONE',  ( -1.000000000000000000, -4.130293990420971855E-17, 0.000000000000000000 ) ) ;
#37482=CARTESIAN_POINT ( 'NONE',  ( -27.24356964374999279, 196.2968750006145342, 15.72908226750539384 ) ) ;
#37486=CARTESIAN_POINT ( 'NONE',  ( 15.24356964375000167, 240.4468750006145399, 3.323476615752272600 ) ) ;
#37487=CARTESIAN_POINT ( 'NONE',  ( 13.62178482187501416, 199.0531250006145285, 23.59362340125806767 ) ) ;
#37492=CARTESIAN_POINT ( 'NONE',  ( 27.24356964375000345, 197.3281250006145342, -3.336375036156643733E-15 ) ) ;
#37493=CARTESIAN_POINT ( 'NONE',  ( 26.75643035624999655, 242.3593750006145342, -3.323476615752271712 ) ) ;
#37494=CARTESIAN_POINT ( 'NONE',  ( 21.00000000000000000, 243.8125000000000284, 5.999999999999998224 ) ) ;
#37550=COLOUR_RGB('Off White',0.89,0.88,0.83);
#37551=FILL_AREA_STYLE_COLOUR('',#37550);
#37552=FILL_AREA_STYLE('',(#37551));
#37553=SURFACE_STYLE_FILL_AREA(#37552);
#37554=SURFACE_SIDE_STYLE('',(#37553));
#37555=SURFACE_STYLE_USAGE(.BOTH.,#37554);
#37556=PRESENTATION_STYLE_ASSIGNMENT((#37555));
ENDSEC;
END-ISO-10303-21;
